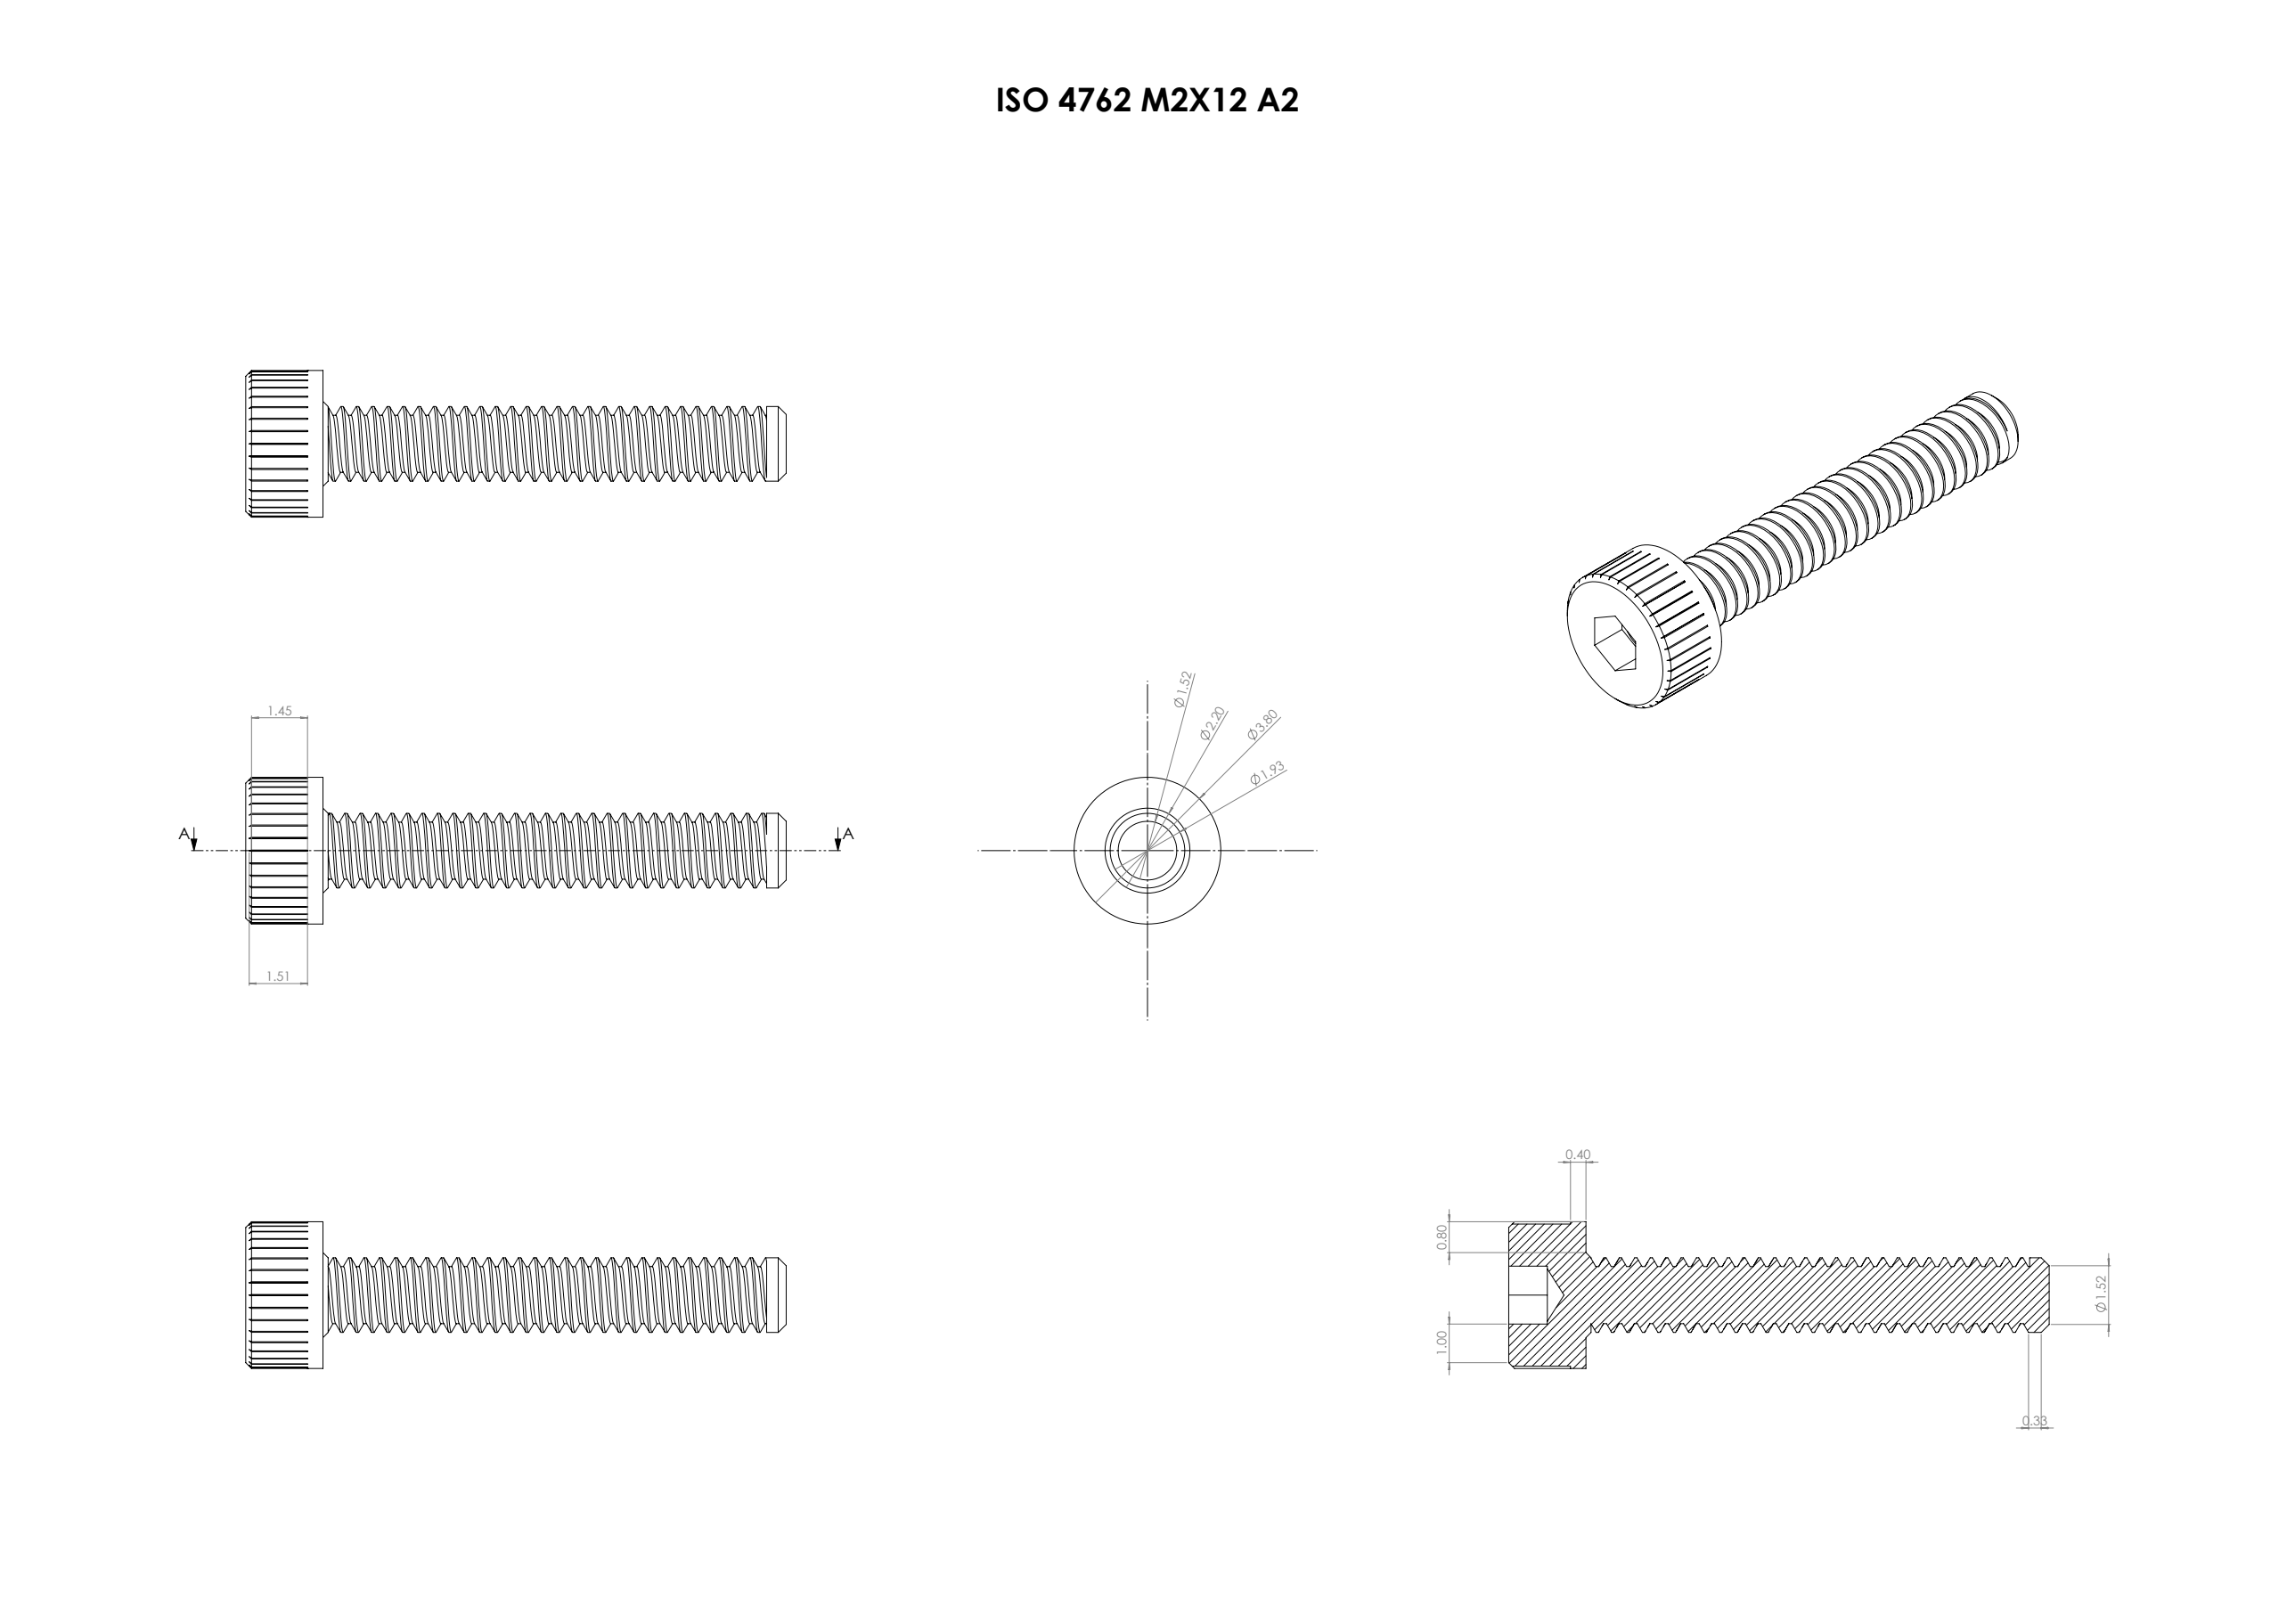
ISO-10303-21;
HEADER;
/* Generated by software containing ST-Developer
 * from STEP Tools, Inc. (www.steptools.com) 
 */

FILE_DESCRIPTION(
/* description */ (''),
/* implementation_level */ '2;1');

FILE_NAME(
/* name */ '15_ISO_4762_M2x12_A2.step',
/* time_stamp */ '2026-10-19T23:00:43-07:00',
/* author */ (''),
/* organization */ (''),
/* preprocessor_version */ 'ST-DEVELOPER v20.2',
/* originating_system */ 'Autodesk Translation Framework v15.15.0.0',
/* authorisation */ '');

FILE_SCHEMA (('AUTOMOTIVE_DESIGN { 1 0 10303 214 3 1 1 }'));
ENDSEC;

DATA;
#10=MECHANICAL_DESIGN_GEOMETRIC_PRESENTATION_REPRESENTATION('',(#1011),#55002);
#251=(
BOUNDED_CURVE()
B_SPLINE_CURVE(2,(#43783,#43784,#43785),.UNSPECIFIED.,.F.,.F.)
B_SPLINE_CURVE_WITH_KNOTS((3,3),(0.,0.00841282944278042),.UNSPECIFIED.)
CURVE()
GEOMETRIC_REPRESENTATION_ITEM()
RATIONAL_B_SPLINE_CURVE((1.,1.00035365746955,1.00043184882983))
REPRESENTATION_ITEM('')
);
#252=(
BOUNDED_CURVE()
B_SPLINE_CURVE(2,(#43789,#43790,#43791),.UNSPECIFIED.,.F.,.F.)
B_SPLINE_CURVE_WITH_KNOTS((3,3),(0.0131888113576721,0.0216016408002996),
 .UNSPECIFIED.)
CURVE()
GEOMETRIC_REPRESENTATION_ITEM()
RATIONAL_B_SPLINE_CURVE((1.00043184882948,1.00035365746926,1.))
REPRESENTATION_ITEM('')
);
#253=(
BOUNDED_CURVE()
B_SPLINE_CURVE(2,(#43804,#43805,#43806),.UNSPECIFIED.,.F.,.F.)
B_SPLINE_CURVE_WITH_KNOTS((3,3),(0.,0.0084128294426201),.UNSPECIFIED.)
CURVE()
GEOMETRIC_REPRESENTATION_ITEM()
RATIONAL_B_SPLINE_CURVE((1.,1.00035365746986,1.00043184883023))
REPRESENTATION_ITEM('')
);
#254=(
BOUNDED_CURVE()
B_SPLINE_CURVE(2,(#43810,#43811,#43812),.UNSPECIFIED.,.F.,.F.)
B_SPLINE_CURVE_WITH_KNOTS((3,3),(0.0131888113575809,0.0216016408002996),
 .UNSPECIFIED.)
CURVE()
GEOMETRIC_REPRESENTATION_ITEM()
RATIONAL_B_SPLINE_CURVE((1.00043184883059,1.00035365747017,1.))
REPRESENTATION_ITEM('')
);
#255=(
BOUNDED_CURVE()
B_SPLINE_CURVE(2,(#43825,#43826,#43827),.UNSPECIFIED.,.F.,.F.)
B_SPLINE_CURVE_WITH_KNOTS((3,3),(0.,0.00841282944278058),.UNSPECIFIED.)
CURVE()
GEOMETRIC_REPRESENTATION_ITEM()
RATIONAL_B_SPLINE_CURVE((1.,1.00035365746906,1.00043184882924))
REPRESENTATION_ITEM('')
);
#256=(
BOUNDED_CURVE()
B_SPLINE_CURVE(2,(#43831,#43832,#43833),.UNSPECIFIED.,.F.,.F.)
B_SPLINE_CURVE_WITH_KNOTS((3,3),(0.0131888113576548,0.0216016408002996),
 .UNSPECIFIED.)
CURVE()
GEOMETRIC_REPRESENTATION_ITEM()
RATIONAL_B_SPLINE_CURVE((1.00043184882846,1.00035365746842,1.))
REPRESENTATION_ITEM('')
);
#257=(
BOUNDED_CURVE()
B_SPLINE_CURVE(2,(#43846,#43847,#43848),.UNSPECIFIED.,.F.,.F.)
B_SPLINE_CURVE_WITH_KNOTS((3,3),(0.,0.00841282944280584),.UNSPECIFIED.)
CURVE()
GEOMETRIC_REPRESENTATION_ITEM()
RATIONAL_B_SPLINE_CURVE((1.,1.00035365746775,1.00043184882763))
REPRESENTATION_ITEM('')
);
#258=(
BOUNDED_CURVE()
B_SPLINE_CURVE(2,(#43852,#43853,#43854),.UNSPECIFIED.,.F.,.F.)
B_SPLINE_CURVE_WITH_KNOTS((3,3),(0.0131888113576015,0.0216016408002996),
 .UNSPECIFIED.)
CURVE()
GEOMETRIC_REPRESENTATION_ITEM()
RATIONAL_B_SPLINE_CURVE((1.00043184882681,1.00035365746707,1.))
REPRESENTATION_ITEM('')
);
#259=(
BOUNDED_CURVE()
B_SPLINE_CURVE(2,(#43867,#43868,#43869),.UNSPECIFIED.,.F.,.F.)
B_SPLINE_CURVE_WITH_KNOTS((3,3),(0.,0.00841282944278488),.UNSPECIFIED.)
CURVE()
GEOMETRIC_REPRESENTATION_ITEM()
RATIONAL_B_SPLINE_CURVE((1.,1.0003536574676,1.00043184882745))
REPRESENTATION_ITEM('')
);
#260=(
BOUNDED_CURVE()
B_SPLINE_CURVE(2,(#43873,#43874,#43875),.UNSPECIFIED.,.F.,.F.)
B_SPLINE_CURVE_WITH_KNOTS((3,3),(0.0131888113575949,0.0216016408002996),
 .UNSPECIFIED.)
CURVE()
GEOMETRIC_REPRESENTATION_ITEM()
RATIONAL_B_SPLINE_CURVE((1.000431848828,1.00035365746804,1.))
REPRESENTATION_ITEM('')
);
#261=(
BOUNDED_CURVE()
B_SPLINE_CURVE(2,(#43888,#43889,#43890),.UNSPECIFIED.,.F.,.F.)
B_SPLINE_CURVE_WITH_KNOTS((3,3),(0.,0.00841282944265237),.UNSPECIFIED.)
CURVE()
GEOMETRIC_REPRESENTATION_ITEM()
RATIONAL_B_SPLINE_CURVE((1.,1.00035365746874,1.00043184882885))
REPRESENTATION_ITEM('')
);
#262=(
BOUNDED_CURVE()
B_SPLINE_CURVE(2,(#43894,#43895,#43896),.UNSPECIFIED.,.F.,.F.)
B_SPLINE_CURVE_WITH_KNOTS((3,3),(0.0131888113575151,0.0216016408002996),
 .UNSPECIFIED.)
CURVE()
GEOMETRIC_REPRESENTATION_ITEM()
RATIONAL_B_SPLINE_CURVE((1.00043184882745,1.0003536574676,1.))
REPRESENTATION_ITEM('')
);
#263=(
BOUNDED_CURVE()
B_SPLINE_CURVE(2,(#43909,#43910,#43911),.UNSPECIFIED.,.F.,.F.)
B_SPLINE_CURVE_WITH_KNOTS((3,3),(0.,0.00841282944265245),.UNSPECIFIED.)
CURVE()
GEOMETRIC_REPRESENTATION_ITEM()
RATIONAL_B_SPLINE_CURVE((1.,1.00035365746621,1.00043184882576))
REPRESENTATION_ITEM('')
);
#264=(
BOUNDED_CURVE()
B_SPLINE_CURVE(2,(#43915,#43916,#43917),.UNSPECIFIED.,.F.,.F.)
B_SPLINE_CURVE_WITH_KNOTS((3,3),(0.013188811357676,0.0216016408002996),
 .UNSPECIFIED.)
CURVE()
GEOMETRIC_REPRESENTATION_ITEM()
RATIONAL_B_SPLINE_CURVE((1.00043184882966,1.0003536574694,1.))
REPRESENTATION_ITEM('')
);
#265=(
BOUNDED_CURVE()
B_SPLINE_CURVE(2,(#43930,#43931,#43932),.UNSPECIFIED.,.F.,.F.)
B_SPLINE_CURVE_WITH_KNOTS((3,3),(0.,0.00841282944263587),.UNSPECIFIED.)
CURVE()
GEOMETRIC_REPRESENTATION_ITEM()
RATIONAL_B_SPLINE_CURVE((1.,1.00035365746699,1.00043184882672))
REPRESENTATION_ITEM('')
);
#266=(
BOUNDED_CURVE()
B_SPLINE_CURVE(2,(#43936,#43937,#43938),.UNSPECIFIED.,.F.,.F.)
B_SPLINE_CURVE_WITH_KNOTS((3,3),(0.0131888113575321,0.0216016408002996),
 .UNSPECIFIED.)
CURVE()
GEOMETRIC_REPRESENTATION_ITEM()
RATIONAL_B_SPLINE_CURVE((1.00043184883015,1.00035365746981,1.))
REPRESENTATION_ITEM('')
);
#267=(
BOUNDED_CURVE()
B_SPLINE_CURVE(2,(#43951,#43952,#43953),.UNSPECIFIED.,.F.,.F.)
B_SPLINE_CURVE_WITH_KNOTS((3,3),(0.,0.00841282944268715),.UNSPECIFIED.)
CURVE()
GEOMETRIC_REPRESENTATION_ITEM()
RATIONAL_B_SPLINE_CURVE((1.,1.00035365746714,1.0004318488269))
REPRESENTATION_ITEM('')
);
#268=(
BOUNDED_CURVE()
B_SPLINE_CURVE(2,(#43957,#43958,#43959),.UNSPECIFIED.,.F.,.F.)
B_SPLINE_CURVE_WITH_KNOTS((3,3),(0.0131888113576173,0.0216016408002996),
 .UNSPECIFIED.)
CURVE()
GEOMETRIC_REPRESENTATION_ITEM()
RATIONAL_B_SPLINE_CURVE((1.00043184882651,1.00035365746683,1.))
REPRESENTATION_ITEM('')
);
#269=(
BOUNDED_CURVE()
B_SPLINE_CURVE(2,(#43972,#43973,#43974),.UNSPECIFIED.,.F.,.F.)
B_SPLINE_CURVE_WITH_KNOTS((3,3),(0.,0.00841282944268232),.UNSPECIFIED.)
CURVE()
GEOMETRIC_REPRESENTATION_ITEM()
RATIONAL_B_SPLINE_CURVE((1.,1.00035365746714,1.0004318488269))
REPRESENTATION_ITEM('')
);
#270=(
BOUNDED_CURVE()
B_SPLINE_CURVE(2,(#43978,#43979,#43980),.UNSPECIFIED.,.F.,.F.)
B_SPLINE_CURVE_WITH_KNOTS((3,3),(0.0131888113576523,0.0216016408002997),
 .UNSPECIFIED.)
CURVE()
GEOMETRIC_REPRESENTATION_ITEM()
RATIONAL_B_SPLINE_CURVE((1.00043184882641,1.00035365746674,1.))
REPRESENTATION_ITEM('')
);
#271=(
BOUNDED_CURVE()
B_SPLINE_CURVE(2,(#43993,#43994,#43995),.UNSPECIFIED.,.F.,.F.)
B_SPLINE_CURVE_WITH_KNOTS((3,3),(0.,0.00841282944262782),.UNSPECIFIED.)
CURVE()
GEOMETRIC_REPRESENTATION_ITEM()
RATIONAL_B_SPLINE_CURVE((1.,1.00035365747069,1.00043184883123))
REPRESENTATION_ITEM('')
);
#272=(
BOUNDED_CURVE()
B_SPLINE_CURVE(2,(#43999,#44000,#44001),.UNSPECIFIED.,.F.,.F.)
B_SPLINE_CURVE_WITH_KNOTS((3,3),(0.0131888113575803,0.0216016408002996),
 .UNSPECIFIED.)
CURVE()
GEOMETRIC_REPRESENTATION_ITEM()
RATIONAL_B_SPLINE_CURVE((1.00043184883154,1.00035365747094,1.))
REPRESENTATION_ITEM('')
);
#273=(
BOUNDED_CURVE()
B_SPLINE_CURVE(2,(#44014,#44015,#44016),.UNSPECIFIED.,.F.,.F.)
B_SPLINE_CURVE_WITH_KNOTS((3,3),(0.,0.00841282944278058),.UNSPECIFIED.)
CURVE()
GEOMETRIC_REPRESENTATION_ITEM()
RATIONAL_B_SPLINE_CURVE((1.,1.00035365746906,1.00043184882924))
REPRESENTATION_ITEM('')
);
#274=(
BOUNDED_CURVE()
B_SPLINE_CURVE(2,(#44020,#44021,#44022),.UNSPECIFIED.,.F.,.F.)
B_SPLINE_CURVE_WITH_KNOTS((3,3),(0.0131888113576548,0.0216016408002996),
 .UNSPECIFIED.)
CURVE()
GEOMETRIC_REPRESENTATION_ITEM()
RATIONAL_B_SPLINE_CURVE((1.00043184882846,1.00035365746842,1.))
REPRESENTATION_ITEM('')
);
#275=(
BOUNDED_CURVE()
B_SPLINE_CURVE(2,(#44035,#44036,#44037),.UNSPECIFIED.,.F.,.F.)
B_SPLINE_CURVE_WITH_KNOTS((3,3),(0.,0.00841282944280138),.UNSPECIFIED.)
CURVE()
GEOMETRIC_REPRESENTATION_ITEM()
RATIONAL_B_SPLINE_CURVE((1.,1.00035365746471,1.00043184882392))
REPRESENTATION_ITEM('')
);
#276=(
BOUNDED_CURVE()
B_SPLINE_CURVE(2,(#44041,#44042,#44043),.UNSPECIFIED.,.F.,.F.)
B_SPLINE_CURVE_WITH_KNOTS((3,3),(0.0131888113575931,0.0216016408002996),
 .UNSPECIFIED.)
CURVE()
GEOMETRIC_REPRESENTATION_ITEM()
RATIONAL_B_SPLINE_CURVE((1.00043184882494,1.00035365746554,1.))
REPRESENTATION_ITEM('')
);
#277=(
BOUNDED_CURVE()
B_SPLINE_CURVE(2,(#44056,#44057,#44058),.UNSPECIFIED.,.F.,.F.)
B_SPLINE_CURVE_WITH_KNOTS((3,3),(0.,0.00841282944261464),.UNSPECIFIED.)
CURVE()
GEOMETRIC_REPRESENTATION_ITEM()
RATIONAL_B_SPLINE_CURVE((1.,1.00035365746679,1.00043184882648))
REPRESENTATION_ITEM('')
);
#278=(
BOUNDED_CURVE()
B_SPLINE_CURVE(2,(#44062,#44063,#44064),.UNSPECIFIED.,.F.,.F.)
B_SPLINE_CURVE_WITH_KNOTS((3,3),(0.0131888113575887,0.0216016408002996),
 .UNSPECIFIED.)
CURVE()
GEOMETRIC_REPRESENTATION_ITEM()
RATIONAL_B_SPLINE_CURVE((1.00043184882758,1.0003536574677,1.))
REPRESENTATION_ITEM('')
);
#279=(
BOUNDED_CURVE()
B_SPLINE_CURVE(2,(#44077,#44078,#44079),.UNSPECIFIED.,.F.,.F.)
B_SPLINE_CURVE_WITH_KNOTS((3,3),(0.,0.00841282944265251),.UNSPECIFIED.)
CURVE()
GEOMETRIC_REPRESENTATION_ITEM()
RATIONAL_B_SPLINE_CURVE((1.,1.00035365746762,1.00043184882748))
REPRESENTATION_ITEM('')
);
#280=(
BOUNDED_CURVE()
B_SPLINE_CURVE(2,(#44083,#44084,#44085),.UNSPECIFIED.,.F.,.F.)
B_SPLINE_CURVE_WITH_KNOTS((3,3),(0.0131888113576473,0.0216016408002996),
 .UNSPECIFIED.)
CURVE()
GEOMETRIC_REPRESENTATION_ITEM()
RATIONAL_B_SPLINE_CURVE((1.00043184883165,1.00035365747103,1.))
REPRESENTATION_ITEM('')
);
#281=(
BOUNDED_CURVE()
B_SPLINE_CURVE(2,(#44098,#44099,#44100),.UNSPECIFIED.,.F.,.F.)
B_SPLINE_CURVE_WITH_KNOTS((3,3),(0.,0.00841282944262983),.UNSPECIFIED.)
CURVE()
GEOMETRIC_REPRESENTATION_ITEM()
RATIONAL_B_SPLINE_CURVE((1.,1.00035365747139,1.00043184883209))
REPRESENTATION_ITEM('')
);
#282=(
BOUNDED_CURVE()
B_SPLINE_CURVE(2,(#44104,#44105,#44106),.UNSPECIFIED.,.F.,.F.)
B_SPLINE_CURVE_WITH_KNOTS((3,3),(0.0131888113576388,0.0216016408002996),
 .UNSPECIFIED.)
CURVE()
GEOMETRIC_REPRESENTATION_ITEM()
RATIONAL_B_SPLINE_CURVE((1.00043184882737,1.00035365746753,1.))
REPRESENTATION_ITEM('')
);
#283=(
BOUNDED_CURVE()
B_SPLINE_CURVE(2,(#44119,#44120,#44121),.UNSPECIFIED.,.F.,.F.)
B_SPLINE_CURVE_WITH_KNOTS((3,3),(0.,0.00841282944261306),.UNSPECIFIED.)
CURVE()
GEOMETRIC_REPRESENTATION_ITEM()
RATIONAL_B_SPLINE_CURVE((1.,1.00035365747318,1.00043184883428))
REPRESENTATION_ITEM('')
);
#284=(
BOUNDED_CURVE()
B_SPLINE_CURVE(2,(#44125,#44126,#44127),.UNSPECIFIED.,.F.,.F.)
B_SPLINE_CURVE_WITH_KNOTS((3,3),(0.0131888113575341,0.0216016408002996),
 .UNSPECIFIED.)
CURVE()
GEOMETRIC_REPRESENTATION_ITEM()
RATIONAL_B_SPLINE_CURVE((1.00043184882813,1.00035365746816,1.))
REPRESENTATION_ITEM('')
);
#285=(
BOUNDED_CURVE()
B_SPLINE_CURVE(2,(#44142,#44143,#44144),.UNSPECIFIED.,.F.,.F.)
B_SPLINE_CURVE_WITH_KNOTS((3,3),(0.,0.00841282944268199),.UNSPECIFIED.)
CURVE()
GEOMETRIC_REPRESENTATION_ITEM()
RATIONAL_B_SPLINE_CURVE((1.,1.00035365746877,1.00043184882888))
REPRESENTATION_ITEM('')
);
#286=(
BOUNDED_CURVE()
B_SPLINE_CURVE(2,(#44148,#44149,#44150),.UNSPECIFIED.,.F.,.F.)
B_SPLINE_CURVE_WITH_KNOTS((3,3),(0.0131888113576103,0.0216016408002996),
 .UNSPECIFIED.)
CURVE()
GEOMETRIC_REPRESENTATION_ITEM()
RATIONAL_B_SPLINE_CURVE((1.00043184882915,1.00035365746898,1.))
REPRESENTATION_ITEM('')
);
#287=(
BOUNDED_CURVE()
B_SPLINE_CURVE(2,(#44163,#44164,#44165),.UNSPECIFIED.,.F.,.F.)
B_SPLINE_CURVE_WITH_KNOTS((3,3),(0.,0.00841282944276111),.UNSPECIFIED.)
CURVE()
GEOMETRIC_REPRESENTATION_ITEM()
RATIONAL_B_SPLINE_CURVE((1.,1.00035365746789,1.00043184882782))
REPRESENTATION_ITEM('')
);
#288=(
BOUNDED_CURVE()
B_SPLINE_CURVE(2,(#44169,#44170,#44171),.UNSPECIFIED.,.F.,.F.)
B_SPLINE_CURVE_WITH_KNOTS((3,3),(0.013188811357663,0.0216016408002997),
 .UNSPECIFIED.)
CURVE()
GEOMETRIC_REPRESENTATION_ITEM()
RATIONAL_B_SPLINE_CURVE((1.00043184882852,1.00035365746847,1.))
REPRESENTATION_ITEM('')
);
#289=(
BOUNDED_CURVE()
B_SPLINE_CURVE(2,(#44184,#44185,#44186),.UNSPECIFIED.,.F.,.F.)
B_SPLINE_CURVE_WITH_KNOTS((3,3),(0.,0.00841282944263208),.UNSPECIFIED.)
CURVE()
GEOMETRIC_REPRESENTATION_ITEM()
RATIONAL_B_SPLINE_CURVE((1.,1.00035365746816,1.00043184882815))
REPRESENTATION_ITEM('')
);
#290=(
BOUNDED_CURVE()
B_SPLINE_CURVE(2,(#44190,#44191,#44192),.UNSPECIFIED.,.F.,.F.)
B_SPLINE_CURVE_WITH_KNOTS((3,3),(0.013188811357748,0.0216016408002996),
 .UNSPECIFIED.)
CURVE()
GEOMETRIC_REPRESENTATION_ITEM()
RATIONAL_B_SPLINE_CURVE((1.00043184883132,1.00035365747076,1.))
REPRESENTATION_ITEM('')
);
#291=(
BOUNDED_CURVE()
B_SPLINE_CURVE(2,(#44205,#44206,#44207),.UNSPECIFIED.,.F.,.F.)
B_SPLINE_CURVE_WITH_KNOTS((3,3),(0.,0.00841282944264326),.UNSPECIFIED.)
CURVE()
GEOMETRIC_REPRESENTATION_ITEM()
RATIONAL_B_SPLINE_CURVE((1.,1.00035365746759,1.00043184882744))
REPRESENTATION_ITEM('')
);
#292=(
BOUNDED_CURVE()
B_SPLINE_CURVE(2,(#44211,#44212,#44213),.UNSPECIFIED.,.F.,.F.)
B_SPLINE_CURVE_WITH_KNOTS((3,3),(0.0131888113575487,0.0216016408002996),
 .UNSPECIFIED.)
CURVE()
GEOMETRIC_REPRESENTATION_ITEM()
RATIONAL_B_SPLINE_CURVE((1.0004318488259,1.00035365746632,1.))
REPRESENTATION_ITEM('')
);
#293=(
BOUNDED_CURVE()
B_SPLINE_CURVE(2,(#44226,#44227,#44228),.UNSPECIFIED.,.F.,.F.)
B_SPLINE_CURVE_WITH_KNOTS((3,3),(0.,0.00841282944280138),.UNSPECIFIED.)
CURVE()
GEOMETRIC_REPRESENTATION_ITEM()
RATIONAL_B_SPLINE_CURVE((1.,1.00035365746471,1.00043184882392))
REPRESENTATION_ITEM('')
);
#294=(
BOUNDED_CURVE()
B_SPLINE_CURVE(2,(#44232,#44233,#44234),.UNSPECIFIED.,.F.,.F.)
B_SPLINE_CURVE_WITH_KNOTS((3,3),(0.0131888113575931,0.0216016408002996),
 .UNSPECIFIED.)
CURVE()
GEOMETRIC_REPRESENTATION_ITEM()
RATIONAL_B_SPLINE_CURVE((1.00043184882494,1.00035365746554,1.))
REPRESENTATION_ITEM('')
);
#295=(
BOUNDED_CURVE()
B_SPLINE_CURVE(2,(#44247,#44248,#44249),.UNSPECIFIED.,.F.,.F.)
B_SPLINE_CURVE_WITH_KNOTS((3,3),(0.,0.00841282944270105),.UNSPECIFIED.)
CURVE()
GEOMETRIC_REPRESENTATION_ITEM()
RATIONAL_B_SPLINE_CURVE((1.,1.000353657467,1.00043184882673))
REPRESENTATION_ITEM('')
);
#296=(
BOUNDED_CURVE()
B_SPLINE_CURVE(2,(#44253,#44254,#44255),.UNSPECIFIED.,.F.,.F.)
B_SPLINE_CURVE_WITH_KNOTS((3,3),(0.0131888113574971,0.0216016408002996),
 .UNSPECIFIED.)
CURVE()
GEOMETRIC_REPRESENTATION_ITEM()
RATIONAL_B_SPLINE_CURVE((1.00043184882773,1.00035365746783,1.))
REPRESENTATION_ITEM('')
);
#297=(
BOUNDED_CURVE()
B_SPLINE_CURVE(2,(#44268,#44269,#44270),.UNSPECIFIED.,.F.,.F.)
B_SPLINE_CURVE_WITH_KNOTS((3,3),(0.,0.00841282944264652),.UNSPECIFIED.)
CURVE()
GEOMETRIC_REPRESENTATION_ITEM()
RATIONAL_B_SPLINE_CURVE((1.,1.00035365746972,1.00043184883004))
REPRESENTATION_ITEM('')
);
#298=(
BOUNDED_CURVE()
B_SPLINE_CURVE(2,(#44274,#44275,#44276),.UNSPECIFIED.,.F.,.F.)
B_SPLINE_CURVE_WITH_KNOTS((3,3),(0.0131888113576371,0.0216016408002996),
 .UNSPECIFIED.)
CURVE()
GEOMETRIC_REPRESENTATION_ITEM()
RATIONAL_B_SPLINE_CURVE((1.00043184882659,1.00035365746689,1.))
REPRESENTATION_ITEM('')
);
#299=(
BOUNDED_CURVE()
B_SPLINE_CURVE(2,(#44289,#44290,#44291),.UNSPECIFIED.,.F.,.F.)
B_SPLINE_CURVE_WITH_KNOTS((3,3),(0.,0.00841282944262983),.UNSPECIFIED.)
CURVE()
GEOMETRIC_REPRESENTATION_ITEM()
RATIONAL_B_SPLINE_CURVE((1.,1.00035365747139,1.00043184883209))
REPRESENTATION_ITEM('')
);
#300=(
BOUNDED_CURVE()
B_SPLINE_CURVE(2,(#44295,#44296,#44297),.UNSPECIFIED.,.F.,.F.)
B_SPLINE_CURVE_WITH_KNOTS((3,3),(0.0131888113576388,0.0216016408002996),
 .UNSPECIFIED.)
CURVE()
GEOMETRIC_REPRESENTATION_ITEM()
RATIONAL_B_SPLINE_CURVE((1.00043184882737,1.00035365746753,1.))
REPRESENTATION_ITEM('')
);
#301=(
BOUNDED_CURVE()
B_SPLINE_CURVE(2,(#44310,#44311,#44312),.UNSPECIFIED.,.F.,.F.)
B_SPLINE_CURVE_WITH_KNOTS((3,3),(0.,0.00841282944264003),.UNSPECIFIED.)
CURVE()
GEOMETRIC_REPRESENTATION_ITEM()
RATIONAL_B_SPLINE_CURVE((1.,1.0003536574673,1.00043184882709))
REPRESENTATION_ITEM('')
);
#302=(
BOUNDED_CURVE()
B_SPLINE_CURVE(2,(#44316,#44317,#44318),.UNSPECIFIED.,.F.,.F.)
B_SPLINE_CURVE_WITH_KNOTS((3,3),(0.0131888113576155,0.0216016408002996),
 .UNSPECIFIED.)
CURVE()
GEOMETRIC_REPRESENTATION_ITEM()
RATIONAL_B_SPLINE_CURVE((1.00043184882608,1.00035365746647,1.))
REPRESENTATION_ITEM('')
);
#303=(
BOUNDED_CURVE()
B_SPLINE_CURVE(2,(#44331,#44332,#44333),.UNSPECIFIED.,.F.,.F.)
B_SPLINE_CURVE_WITH_KNOTS((3,3),(0.,0.00841282944269557),.UNSPECIFIED.)
CURVE()
GEOMETRIC_REPRESENTATION_ITEM()
RATIONAL_B_SPLINE_CURVE((1.,1.00035365746722,1.000431848827))
REPRESENTATION_ITEM('')
);
#304=(
BOUNDED_CURVE()
B_SPLINE_CURVE(2,(#44337,#44338,#44339),.UNSPECIFIED.,.F.,.F.)
B_SPLINE_CURVE_WITH_KNOTS((3,3),(0.0131888113576143,0.0216016408002996),
 .UNSPECIFIED.)
CURVE()
GEOMETRIC_REPRESENTATION_ITEM()
RATIONAL_B_SPLINE_CURVE((1.00043184882947,1.00035365746925,1.))
REPRESENTATION_ITEM('')
);
#305=(
BOUNDED_CURVE()
B_SPLINE_CURVE(2,(#44352,#44353,#44354),.UNSPECIFIED.,.F.,.F.)
B_SPLINE_CURVE_WITH_KNOTS((3,3),(0.,0.00841282944278065),.UNSPECIFIED.)
CURVE()
GEOMETRIC_REPRESENTATION_ITEM()
RATIONAL_B_SPLINE_CURVE((1.,1.00035365746947,1.00043184882974))
REPRESENTATION_ITEM('')
);
#306=(
BOUNDED_CURVE()
B_SPLINE_CURVE(2,(#44358,#44359,#44360),.UNSPECIFIED.,.F.,.F.)
B_SPLINE_CURVE_WITH_KNOTS((3,3),(0.0131888113576697,0.0216016408002996),
 .UNSPECIFIED.)
CURVE()
GEOMETRIC_REPRESENTATION_ITEM()
RATIONAL_B_SPLINE_CURVE((1.00043184882899,1.00035365746886,1.))
REPRESENTATION_ITEM('')
);
#307=(
BOUNDED_CURVE()
B_SPLINE_CURVE(2,(#44373,#44374,#44375),.UNSPECIFIED.,.F.,.F.)
B_SPLINE_CURVE_WITH_KNOTS((3,3),(0.,0.00841282944263208),.UNSPECIFIED.)
CURVE()
GEOMETRIC_REPRESENTATION_ITEM()
RATIONAL_B_SPLINE_CURVE((1.,1.00035365746816,1.00043184882815))
REPRESENTATION_ITEM('')
);
#308=(
BOUNDED_CURVE()
B_SPLINE_CURVE(2,(#44379,#44380,#44381),.UNSPECIFIED.,.F.,.F.)
B_SPLINE_CURVE_WITH_KNOTS((3,3),(0.013188811357748,0.0216016408002996),
 .UNSPECIFIED.)
CURVE()
GEOMETRIC_REPRESENTATION_ITEM()
RATIONAL_B_SPLINE_CURVE((1.00043184883132,1.00035365747076,1.))
REPRESENTATION_ITEM('')
);
#309=(
BOUNDED_CURVE()
B_SPLINE_CURVE(2,(#44394,#44395,#44396),.UNSPECIFIED.,.F.,.F.)
B_SPLINE_CURVE_WITH_KNOTS((3,3),(0.,0.00841282944273455),.UNSPECIFIED.)
CURVE()
GEOMETRIC_REPRESENTATION_ITEM()
RATIONAL_B_SPLINE_CURVE((1.,1.00035365746539,1.00043184882476))
REPRESENTATION_ITEM('')
);
#310=(
BOUNDED_CURVE()
B_SPLINE_CURVE(2,(#44400,#44401,#44402),.UNSPECIFIED.,.F.,.F.)
B_SPLINE_CURVE_WITH_KNOTS((3,3),(0.0131888113576539,0.0216016408002996),
 .UNSPECIFIED.)
CURVE()
GEOMETRIC_REPRESENTATION_ITEM()
RATIONAL_B_SPLINE_CURVE((1.00043184882929,1.0003536574691,1.))
REPRESENTATION_ITEM('')
);
#311=(
BOUNDED_CURVE()
B_SPLINE_CURVE(2,(#44415,#44416,#44417),.UNSPECIFIED.,.F.,.F.)
B_SPLINE_CURVE_WITH_KNOTS((3,3),(0.,0.00841282944270133),.UNSPECIFIED.)
CURVE()
GEOMETRIC_REPRESENTATION_ITEM()
RATIONAL_B_SPLINE_CURVE((1.,1.00035365747008,1.00043184883048))
REPRESENTATION_ITEM('')
);
#312=(
BOUNDED_CURVE()
B_SPLINE_CURVE(2,(#44421,#44422,#44423),.UNSPECIFIED.,.F.,.F.)
B_SPLINE_CURVE_WITH_KNOTS((3,3),(0.0131888113576197,0.0216016408002996),
 .UNSPECIFIED.)
CURVE()
GEOMETRIC_REPRESENTATION_ITEM()
RATIONAL_B_SPLINE_CURVE((1.00043184882798,1.00035365746803,1.))
REPRESENTATION_ITEM('')
);
#313=(
BOUNDED_CURVE()
B_SPLINE_CURVE(2,(#44436,#44437,#44438),.UNSPECIFIED.,.F.,.F.)
B_SPLINE_CURVE_WITH_KNOTS((3,3),(0.,0.00841282944261464),.UNSPECIFIED.)
CURVE()
GEOMETRIC_REPRESENTATION_ITEM()
RATIONAL_B_SPLINE_CURVE((1.,1.00035365746679,1.00043184882648))
REPRESENTATION_ITEM('')
);
#314=(
BOUNDED_CURVE()
B_SPLINE_CURVE(2,(#44442,#44443,#44444),.UNSPECIFIED.,.F.,.F.)
B_SPLINE_CURVE_WITH_KNOTS((3,3),(0.0131888113575887,0.0216016408002996),
 .UNSPECIFIED.)
CURVE()
GEOMETRIC_REPRESENTATION_ITEM()
RATIONAL_B_SPLINE_CURVE((1.00043184882758,1.0003536574677,1.))
REPRESENTATION_ITEM('')
);
#315=(
BOUNDED_CURVE()
B_SPLINE_CURVE(2,(#44457,#44458,#44459),.UNSPECIFIED.,.F.,.F.)
B_SPLINE_CURVE_WITH_KNOTS((3,3),(0.,0.00841282944264924),.UNSPECIFIED.)
CURVE()
GEOMETRIC_REPRESENTATION_ITEM()
RATIONAL_B_SPLINE_CURVE((1.,1.00035365746952,1.00043184882981))
REPRESENTATION_ITEM('')
);
#316=(
BOUNDED_CURVE()
B_SPLINE_CURVE(2,(#44463,#44464,#44465),.UNSPECIFIED.,.F.,.F.)
B_SPLINE_CURVE_WITH_KNOTS((3,3),(0.0131888113576407,0.0216016408002996),
 .UNSPECIFIED.)
CURVE()
GEOMETRIC_REPRESENTATION_ITEM()
RATIONAL_B_SPLINE_CURVE((1.00043184882821,1.00035365746821,1.))
REPRESENTATION_ITEM('')
);
#317=(
BOUNDED_CURVE()
B_SPLINE_CURVE(2,(#44478,#44479,#44480),.UNSPECIFIED.,.F.,.F.)
B_SPLINE_CURVE_WITH_KNOTS((3,3),(0.,0.00841282944262983),.UNSPECIFIED.)
CURVE()
GEOMETRIC_REPRESENTATION_ITEM()
RATIONAL_B_SPLINE_CURVE((1.,1.00035365747139,1.00043184883209))
REPRESENTATION_ITEM('')
);
#318=(
BOUNDED_CURVE()
B_SPLINE_CURVE(2,(#44484,#44485,#44486),.UNSPECIFIED.,.F.,.F.)
B_SPLINE_CURVE_WITH_KNOTS((3,3),(0.0131888113576388,0.0216016408002996),
 .UNSPECIFIED.)
CURVE()
GEOMETRIC_REPRESENTATION_ITEM()
RATIONAL_B_SPLINE_CURVE((1.00043184882737,1.00035365746753,1.))
REPRESENTATION_ITEM('')
);
#319=(
BOUNDED_CURVE()
B_SPLINE_CURVE(2,(#44499,#44500,#44501),.UNSPECIFIED.,.F.,.F.)
B_SPLINE_CURVE_WITH_KNOTS((3,3),(0.,0.0084128294426321),.UNSPECIFIED.)
CURVE()
GEOMETRIC_REPRESENTATION_ITEM()
RATIONAL_B_SPLINE_CURVE((1.,1.00035365746883,1.00043184882896))
REPRESENTATION_ITEM('')
);
#320=(
BOUNDED_CURVE()
B_SPLINE_CURVE(2,(#44505,#44506,#44507),.UNSPECIFIED.,.F.,.F.)
B_SPLINE_CURVE_WITH_KNOTS((3,3),(0.0131888113575073,0.0216016408002996),
 .UNSPECIFIED.)
CURVE()
GEOMETRIC_REPRESENTATION_ITEM()
RATIONAL_B_SPLINE_CURVE((1.00043184882395,1.00035365746473,1.))
REPRESENTATION_ITEM('')
);
#321=(
BOUNDED_CURVE()
B_SPLINE_CURVE(2,(#44560,#44561,#44562),.UNSPECIFIED.,.F.,.F.)
B_SPLINE_CURVE_WITH_KNOTS((3,3),(0.,0.00841282944285724),.UNSPECIFIED.)
CURVE()
GEOMETRIC_REPRESENTATION_ITEM()
RATIONAL_B_SPLINE_CURVE((1.,1.00035365746964,1.00043184882994))
REPRESENTATION_ITEM('')
);
#322=(
BOUNDED_CURVE()
B_SPLINE_CURVE(2,(#44564,#44565,#44566),.UNSPECIFIED.,.F.,.F.)
B_SPLINE_CURVE_WITH_KNOTS((3,3),(0.0131888113574265,0.0216016408002996),
 .UNSPECIFIED.)
CURVE()
GEOMETRIC_REPRESENTATION_ITEM()
RATIONAL_B_SPLINE_CURVE((1.00043184882266,1.00035365746368,1.))
REPRESENTATION_ITEM('')
);
#474=B_SPLINE_SURFACE_WITH_KNOTS('',3,3,((#42155,#42156,#42157,#42158,#42159,
#42160,#42161,#42162,#42163,#42164,#42165,#42166,#42167,#42168,#42169,#42170,
#42171,#42172,#42173,#42174,#42175,#42176,#42177,#42178,#42179,#42180,#42181,
#42182,#42183,#42184,#42185,#42186,#42187,#42188,#42189,#42190,#42191,#42192,
#42193,#42194,#42195,#42196,#42197,#42198,#42199,#42200,#42201,#42202,#42203,
#42204,#42205,#42206,#42207,#42208,#42209,#42210,#42211,#42212,#42213,#42214,
#42215,#42216,#42217,#42218,#42219,#42220,#42221,#42222,#42223,#42224,#42225,
#42226,#42227,#42228,#42229,#42230,#42231,#42232,#42233,#42234,#42235,#42236,
#42237,#42238,#42239,#42240,#42241,#42242,#42243,#42244,#42245,#42246,#42247,
#42248,#42249,#42250,#42251,#42252,#42253,#42254,#42255,#42256,#42257,#42258,
#42259,#42260,#42261,#42262,#42263,#42264,#42265,#42266,#42267,#42268,#42269,
#42270,#42271,#42272,#42273,#42274,#42275,#42276,#42277,#42278,#42279,#42280,
#42281,#42282,#42283,#42284,#42285,#42286,#42287,#42288,#42289,#42290,#42291,
#42292,#42293,#42294,#42295,#42296,#42297,#42298,#42299,#42300,#42301,#42302,
#42303,#42304,#42305,#42306,#42307,#42308,#42309,#42310,#42311,#42312,#42313,
#42314,#42315,#42316,#42317,#42318,#42319,#42320,#42321,#42322,#42323,#42324,
#42325,#42326,#42327,#42328,#42329,#42330,#42331,#42332,#42333,#42334,#42335,
#42336,#42337,#42338),(#42339,#42340,#42341,#42342,#42343,#42344,#42345,
#42346,#42347,#42348,#42349,#42350,#42351,#42352,#42353,#42354,#42355,#42356,
#42357,#42358,#42359,#42360,#42361,#42362,#42363,#42364,#42365,#42366,#42367,
#42368,#42369,#42370,#42371,#42372,#42373,#42374,#42375,#42376,#42377,#42378,
#42379,#42380,#42381,#42382,#42383,#42384,#42385,#42386,#42387,#42388,#42389,
#42390,#42391,#42392,#42393,#42394,#42395,#42396,#42397,#42398,#42399,#42400,
#42401,#42402,#42403,#42404,#42405,#42406,#42407,#42408,#42409,#42410,#42411,
#42412,#42413,#42414,#42415,#42416,#42417,#42418,#42419,#42420,#42421,#42422,
#42423,#42424,#42425,#42426,#42427,#42428,#42429,#42430,#42431,#42432,#42433,
#42434,#42435,#42436,#42437,#42438,#42439,#42440,#42441,#42442,#42443,#42444,
#42445,#42446,#42447,#42448,#42449,#42450,#42451,#42452,#42453,#42454,#42455,
#42456,#42457,#42458,#42459,#42460,#42461,#42462,#42463,#42464,#42465,#42466,
#42467,#42468,#42469,#42470,#42471,#42472,#42473,#42474,#42475,#42476,#42477,
#42478,#42479,#42480,#42481,#42482,#42483,#42484,#42485,#42486,#42487,#42488,
#42489,#42490,#42491,#42492,#42493,#42494,#42495,#42496,#42497,#42498,#42499,
#42500,#42501,#42502,#42503,#42504,#42505,#42506,#42507,#42508,#42509,#42510,
#42511,#42512,#42513,#42514,#42515,#42516,#42517,#42518,#42519,#42520,#42521,
#42522),(#42523,#42524,#42525,#42526,#42527,#42528,#42529,#42530,#42531,
#42532,#42533,#42534,#42535,#42536,#42537,#42538,#42539,#42540,#42541,#42542,
#42543,#42544,#42545,#42546,#42547,#42548,#42549,#42550,#42551,#42552,#42553,
#42554,#42555,#42556,#42557,#42558,#42559,#42560,#42561,#42562,#42563,#42564,
#42565,#42566,#42567,#42568,#42569,#42570,#42571,#42572,#42573,#42574,#42575,
#42576,#42577,#42578,#42579,#42580,#42581,#42582,#42583,#42584,#42585,#42586,
#42587,#42588,#42589,#42590,#42591,#42592,#42593,#42594,#42595,#42596,#42597,
#42598,#42599,#42600,#42601,#42602,#42603,#42604,#42605,#42606,#42607,#42608,
#42609,#42610,#42611,#42612,#42613,#42614,#42615,#42616,#42617,#42618,#42619,
#42620,#42621,#42622,#42623,#42624,#42625,#42626,#42627,#42628,#42629,#42630,
#42631,#42632,#42633,#42634,#42635,#42636,#42637,#42638,#42639,#42640,#42641,
#42642,#42643,#42644,#42645,#42646,#42647,#42648,#42649,#42650,#42651,#42652,
#42653,#42654,#42655,#42656,#42657,#42658,#42659,#42660,#42661,#42662,#42663,
#42664,#42665,#42666,#42667,#42668,#42669,#42670,#42671,#42672,#42673,#42674,
#42675,#42676,#42677,#42678,#42679,#42680,#42681,#42682,#42683,#42684,#42685,
#42686,#42687,#42688,#42689,#42690,#42691,#42692,#42693,#42694,#42695,#42696,
#42697,#42698,#42699,#42700,#42701,#42702,#42703,#42704,#42705,#42706),
(#42707,#42708,#42709,#42710,#42711,#42712,#42713,#42714,#42715,#42716,
#42717,#42718,#42719,#42720,#42721,#42722,#42723,#42724,#42725,#42726,#42727,
#42728,#42729,#42730,#42731,#42732,#42733,#42734,#42735,#42736,#42737,#42738,
#42739,#42740,#42741,#42742,#42743,#42744,#42745,#42746,#42747,#42748,#42749,
#42750,#42751,#42752,#42753,#42754,#42755,#42756,#42757,#42758,#42759,#42760,
#42761,#42762,#42763,#42764,#42765,#42766,#42767,#42768,#42769,#42770,#42771,
#42772,#42773,#42774,#42775,#42776,#42777,#42778,#42779,#42780,#42781,#42782,
#42783,#42784,#42785,#42786,#42787,#42788,#42789,#42790,#42791,#42792,#42793,
#42794,#42795,#42796,#42797,#42798,#42799,#42800,#42801,#42802,#42803,#42804,
#42805,#42806,#42807,#42808,#42809,#42810,#42811,#42812,#42813,#42814,#42815,
#42816,#42817,#42818,#42819,#42820,#42821,#42822,#42823,#42824,#42825,#42826,
#42827,#42828,#42829,#42830,#42831,#42832,#42833,#42834,#42835,#42836,#42837,
#42838,#42839,#42840,#42841,#42842,#42843,#42844,#42845,#42846,#42847,#42848,
#42849,#42850,#42851,#42852,#42853,#42854,#42855,#42856,#42857,#42858,#42859,
#42860,#42861,#42862,#42863,#42864,#42865,#42866,#42867,#42868,#42869,#42870,
#42871,#42872,#42873,#42874,#42875,#42876,#42877,#42878,#42879,#42880,#42881,
#42882,#42883,#42884,#42885,#42886,#42887,#42888,#42889,#42890)),
 .UNSPECIFIED.,.F.,.F.,.F.,(4,4),(4,1,1,1,1,1,1,1,1,1,1,1,1,1,1,1,1,1,1,
1,1,1,1,1,1,1,1,1,1,1,1,1,1,1,1,1,1,1,1,1,1,1,1,1,1,1,1,1,1,1,1,1,1,1,1,
1,1,1,1,1,1,1,1,1,1,1,1,1,1,1,1,1,1,1,1,1,1,1,1,1,1,1,1,1,1,1,1,1,1,1,1,
1,1,1,1,1,1,1,1,1,1,1,1,1,1,1,1,1,1,1,1,1,1,1,1,1,1,1,1,1,1,1,1,1,1,1,1,
1,1,1,1,1,1,1,1,1,1,1,1,1,1,1,1,1,1,1,1,1,1,1,1,1,1,1,1,1,1,1,1,1,1,1,1,
1,1,1,1,1,1,1,1,1,1,1,1,1,1,1,1,1,1,4),(0.,0.0262983047615874),(13.0216803321501,
14.0189616954093,15.0162430586686,16.0135244219278,17.010805785187,18.0080871484463,
19.0053685117055,20.0026498749647,20.999931238224,21.9972126014832,22.9944939647424,
23.9917753280017,24.9890566912609,25.9863380545202,26.9836194177794,27.9809007810386,
28.9781821442979,29.9754635075571,30.9727448708163,31.9700262340756,32.9673075973348,
33.9645889605941,34.9618703238533,35.9591516871125,36.9564330503718,37.953714413631,
38.9509957768902,39.9482771401495,40.9455585034087,41.942839866668,42.9401212299272,
43.9374025931864,44.9346839564457,45.9319653197049,46.9292466829641,47.9265280462234,
48.9238094094826,49.9210907727419,50.9183721360011,51.9156534992603,52.9129348625196,
53.9102162257788,54.907497589038,55.9047789522973,56.9020603155565,57.8993416788158,
58.896623042075,59.8939044053342,60.8911857685935,61.8884671318527,62.8857484951119,
63.8830298583712,64.8803112216304,65.8775925848897,66.8748739481489,67.8721553114081,
68.8694366746674,69.8667180379266,70.8639994011859,71.8612807644451,72.8585621277043,
73.8558434909636,74.8531248542228,75.850406217482,76.8476875807413,77.8449689440005,
78.8422503072597,79.839531670519,80.8368130337782,81.8340943970375,82.8313757602967,
83.8286571235559,84.8259384868152,85.8232198500744,86.8205012133336,87.8177825765929,
88.8150639398521,89.8123453031114,90.8096266663706,91.8069080296298,92.8041893928891,
93.8014707561483,94.7987521194075,95.7960334826668,96.793314845926,97.7905962091853,
98.7878775724445,99.7851589357037,100.782440298963,101.779721662222,102.777003025481,
103.774284388741,104.771565752,105.768847115259,106.766128478518,107.763409841778,
108.760691205037,109.757972568296,110.755253931555,111.752535294815,112.749816658074,
113.747098021333,114.744379384592,115.741660747852,116.738942111111,117.73622347437,
118.733504837629,119.730786200888,120.728067564148,121.725348927407,122.722630290666,
123.719911653925,124.717193017185,125.714474380444,126.711755743703,127.709037106962,
128.706318470222,129.703599833481,130.70088119674,131.698162559999,132.695443923259,
133.692725286518,134.690006649777,135.687288013036,136.684569376296,137.681850739555,
138.679132102814,139.676413466073,140.673694829332,141.670976192592,142.668257555851,
143.66553891911,144.662820282369,145.660101645629,146.657383008888,147.654664372147,
148.651945735406,149.649227098666,150.646508461925,151.643789825184,152.641071188443,
153.638352551703,154.635633914962,155.632915278221,156.63019664148,157.627478004739,
158.624759367999,159.622040731258,160.619322094517,161.616603457776,162.613884821036,
163.611166184295,164.608447547554,165.605728910813,166.603010274073,167.600291637332,
168.597573000591,169.59485436385,170.59213572711,171.589417090369,172.586698453628,
173.583979816887,174.581261180147,175.578542543406,176.575823906665,177.573105269924,
178.570386633183,179.567667996443,180.564949359702,181.562230722961,182.55951208622,
183.55679344948,184.554074812739,185.551356175998,186.548637539257,187.545918902517,
188.543200265776,189.540481629035,190.537762992294,191.535044355554,192.532325718813,
193.529607082072),.UNSPECIFIED.);
#475=B_SPLINE_SURFACE_WITH_KNOTS('',3,3,((#43016,#43017,#43018,#43019,#43020,
#43021,#43022,#43023,#43024,#43025,#43026,#43027,#43028,#43029,#43030,#43031,
#43032,#43033,#43034,#43035,#43036,#43037,#43038,#43039,#43040,#43041,#43042,
#43043,#43044,#43045,#43046,#43047,#43048,#43049,#43050,#43051,#43052,#43053,
#43054,#43055,#43056,#43057,#43058,#43059,#43060,#43061,#43062,#43063,#43064,
#43065,#43066,#43067,#43068,#43069,#43070,#43071,#43072,#43073,#43074,#43075,
#43076,#43077,#43078,#43079,#43080,#43081,#43082,#43083,#43084,#43085,#43086,
#43087,#43088,#43089,#43090,#43091,#43092,#43093,#43094,#43095,#43096,#43097,
#43098,#43099,#43100,#43101,#43102,#43103,#43104,#43105,#43106,#43107,#43108,
#43109,#43110,#43111,#43112,#43113,#43114,#43115,#43116,#43117,#43118,#43119,
#43120,#43121,#43122,#43123,#43124,#43125,#43126,#43127,#43128,#43129,#43130,
#43131,#43132,#43133,#43134,#43135,#43136,#43137,#43138,#43139,#43140,#43141,
#43142,#43143,#43144,#43145,#43146,#43147,#43148,#43149,#43150,#43151,#43152,
#43153,#43154,#43155,#43156,#43157,#43158,#43159,#43160,#43161,#43162,#43163,
#43164,#43165,#43166,#43167,#43168,#43169,#43170,#43171,#43172,#43173,#43174,
#43175,#43176,#43177,#43178,#43179,#43180,#43181,#43182,#43183,#43184,#43185,
#43186,#43187,#43188,#43189,#43190,#43191,#43192,#43193,#43194,#43195,#43196,
#43197,#43198,#43199),(#43200,#43201,#43202,#43203,#43204,#43205,#43206,
#43207,#43208,#43209,#43210,#43211,#43212,#43213,#43214,#43215,#43216,#43217,
#43218,#43219,#43220,#43221,#43222,#43223,#43224,#43225,#43226,#43227,#43228,
#43229,#43230,#43231,#43232,#43233,#43234,#43235,#43236,#43237,#43238,#43239,
#43240,#43241,#43242,#43243,#43244,#43245,#43246,#43247,#43248,#43249,#43250,
#43251,#43252,#43253,#43254,#43255,#43256,#43257,#43258,#43259,#43260,#43261,
#43262,#43263,#43264,#43265,#43266,#43267,#43268,#43269,#43270,#43271,#43272,
#43273,#43274,#43275,#43276,#43277,#43278,#43279,#43280,#43281,#43282,#43283,
#43284,#43285,#43286,#43287,#43288,#43289,#43290,#43291,#43292,#43293,#43294,
#43295,#43296,#43297,#43298,#43299,#43300,#43301,#43302,#43303,#43304,#43305,
#43306,#43307,#43308,#43309,#43310,#43311,#43312,#43313,#43314,#43315,#43316,
#43317,#43318,#43319,#43320,#43321,#43322,#43323,#43324,#43325,#43326,#43327,
#43328,#43329,#43330,#43331,#43332,#43333,#43334,#43335,#43336,#43337,#43338,
#43339,#43340,#43341,#43342,#43343,#43344,#43345,#43346,#43347,#43348,#43349,
#43350,#43351,#43352,#43353,#43354,#43355,#43356,#43357,#43358,#43359,#43360,
#43361,#43362,#43363,#43364,#43365,#43366,#43367,#43368,#43369,#43370,#43371,
#43372,#43373,#43374,#43375,#43376,#43377,#43378,#43379,#43380,#43381,#43382,
#43383),(#43384,#43385,#43386,#43387,#43388,#43389,#43390,#43391,#43392,
#43393,#43394,#43395,#43396,#43397,#43398,#43399,#43400,#43401,#43402,#43403,
#43404,#43405,#43406,#43407,#43408,#43409,#43410,#43411,#43412,#43413,#43414,
#43415,#43416,#43417,#43418,#43419,#43420,#43421,#43422,#43423,#43424,#43425,
#43426,#43427,#43428,#43429,#43430,#43431,#43432,#43433,#43434,#43435,#43436,
#43437,#43438,#43439,#43440,#43441,#43442,#43443,#43444,#43445,#43446,#43447,
#43448,#43449,#43450,#43451,#43452,#43453,#43454,#43455,#43456,#43457,#43458,
#43459,#43460,#43461,#43462,#43463,#43464,#43465,#43466,#43467,#43468,#43469,
#43470,#43471,#43472,#43473,#43474,#43475,#43476,#43477,#43478,#43479,#43480,
#43481,#43482,#43483,#43484,#43485,#43486,#43487,#43488,#43489,#43490,#43491,
#43492,#43493,#43494,#43495,#43496,#43497,#43498,#43499,#43500,#43501,#43502,
#43503,#43504,#43505,#43506,#43507,#43508,#43509,#43510,#43511,#43512,#43513,
#43514,#43515,#43516,#43517,#43518,#43519,#43520,#43521,#43522,#43523,#43524,
#43525,#43526,#43527,#43528,#43529,#43530,#43531,#43532,#43533,#43534,#43535,
#43536,#43537,#43538,#43539,#43540,#43541,#43542,#43543,#43544,#43545,#43546,
#43547,#43548,#43549,#43550,#43551,#43552,#43553,#43554,#43555,#43556,#43557,
#43558,#43559,#43560,#43561,#43562,#43563,#43564,#43565,#43566,#43567),
(#43568,#43569,#43570,#43571,#43572,#43573,#43574,#43575,#43576,#43577,
#43578,#43579,#43580,#43581,#43582,#43583,#43584,#43585,#43586,#43587,#43588,
#43589,#43590,#43591,#43592,#43593,#43594,#43595,#43596,#43597,#43598,#43599,
#43600,#43601,#43602,#43603,#43604,#43605,#43606,#43607,#43608,#43609,#43610,
#43611,#43612,#43613,#43614,#43615,#43616,#43617,#43618,#43619,#43620,#43621,
#43622,#43623,#43624,#43625,#43626,#43627,#43628,#43629,#43630,#43631,#43632,
#43633,#43634,#43635,#43636,#43637,#43638,#43639,#43640,#43641,#43642,#43643,
#43644,#43645,#43646,#43647,#43648,#43649,#43650,#43651,#43652,#43653,#43654,
#43655,#43656,#43657,#43658,#43659,#43660,#43661,#43662,#43663,#43664,#43665,
#43666,#43667,#43668,#43669,#43670,#43671,#43672,#43673,#43674,#43675,#43676,
#43677,#43678,#43679,#43680,#43681,#43682,#43683,#43684,#43685,#43686,#43687,
#43688,#43689,#43690,#43691,#43692,#43693,#43694,#43695,#43696,#43697,#43698,
#43699,#43700,#43701,#43702,#43703,#43704,#43705,#43706,#43707,#43708,#43709,
#43710,#43711,#43712,#43713,#43714,#43715,#43716,#43717,#43718,#43719,#43720,
#43721,#43722,#43723,#43724,#43725,#43726,#43727,#43728,#43729,#43730,#43731,
#43732,#43733,#43734,#43735,#43736,#43737,#43738,#43739,#43740,#43741,#43742,
#43743,#43744,#43745,#43746,#43747,#43748,#43749,#43750,#43751)),
 .UNSPECIFIED.,.F.,.F.,.F.,(4,4),(4,1,1,1,1,1,1,1,1,1,1,1,1,1,1,1,1,1,1,
1,1,1,1,1,1,1,1,1,1,1,1,1,1,1,1,1,1,1,1,1,1,1,1,1,1,1,1,1,1,1,1,1,1,1,1,
1,1,1,1,1,1,1,1,1,1,1,1,1,1,1,1,1,1,1,1,1,1,1,1,1,1,1,1,1,1,1,1,1,1,1,1,
1,1,1,1,1,1,1,1,1,1,1,1,1,1,1,1,1,1,1,1,1,1,1,1,1,1,1,1,1,1,1,1,1,1,1,1,
1,1,1,1,1,1,1,1,1,1,1,1,1,1,1,1,1,1,1,1,1,1,1,1,1,1,1,1,1,1,1,1,1,1,1,1,
1,1,1,1,1,1,1,1,1,1,1,1,1,1,1,1,1,1,4),(0.,0.0262983047615874),(16.3287821777263,
17.3260635409855,18.3233449042448,19.320626267504,20.3179076307632,21.3151889940225,
22.3124703572817,23.3097517205409,24.3070330838002,25.3043144470594,26.3015958103187,
27.2988771735779,28.2961585368371,29.2934399000964,30.2907212633556,31.2880026266148,
32.2852839898741,33.2825653531333,34.2798467163926,35.2771280796518,36.274409442911,
37.2716908061703,38.2689721694295,39.2662535326887,40.263534895948,41.2608162592072,
42.2580976224665,43.2553789857257,44.2526603489849,45.2499417122442,46.2472230755034,
47.2445044387626,48.2417858020219,49.2390671652811,50.2363485285403,51.2336298917996,
52.2309112550588,53.2281926183181,54.2254739815773,55.2227553448365,56.2200367080958,
57.217318071355,58.2145994346142,59.2118807978735,60.2091621611327,61.206443524392,
62.2037248876512,63.2010062509104,64.1982876141697,65.1955689774289,66.1928503406881,
67.1901317039474,68.1874130672066,69.1846944304658,70.1819757937251,71.1792571569843,
72.1765385202436,73.1738198835028,74.171101246762,75.1683826100213,76.1656639732805,
77.1629453365397,78.160226699799,79.1575080630582,80.1547894263174,81.1520707895767,
82.1493521528359,83.1466335160952,84.1439148793544,85.1411962426136,86.1384776058729,
87.1357589691321,88.1330403323914,89.1303216956506,90.1276030589098,91.1248844221691,
92.1221657854283,93.1194471486875,94.1167285119468,95.114009875206,96.1112912384653,
97.1085726017245,98.1058539649837,99.103135328243,100.100416691502,101.097698054761,
102.094979418021,103.09226078128,104.089542144539,105.086823507798,106.084104871058,
107.081386234317,108.078667597576,109.075948960835,110.073230324095,111.070511687354,
112.067793050613,113.065074413872,114.062355777132,115.059637140391,116.05691850365,
117.054199866909,118.051481230168,119.048762593428,120.046043956687,121.043325319946,
122.040606683205,123.037888046465,124.035169409724,125.032450772983,126.029732136242,
127.027013499502,128.024294862761,129.02157622602,130.018857589279,131.016138952539,
132.013420315798,133.010701679057,134.007983042316,135.005264405576,136.002545768835,
136.999827132094,137.997108495353,138.994389858612,139.991671221872,140.988952585131,
141.98623394839,142.983515311649,143.980796674909,144.978078038168,145.975359401427,
146.972640764686,147.969922127946,148.967203491205,149.964484854464,150.961766217723,
151.959047580983,152.956328944242,153.953610307501,154.95089167076,155.948173034019,
156.945454397279,157.942735760538,158.940017123797,159.937298487056,160.934579850316,
161.931861213575,162.929142576834,163.926423940093,164.923705303353,165.920986666612,
166.918268029871,167.91554939313,168.91283075639,169.910112119649,170.907393482908,
171.904674846167,172.901956209427,173.899237572686,174.896518935945,175.893800299204,
176.891081662463,177.888363025723,178.885644388982,179.882925752241,180.8802071155,
181.87748847876,182.874769842019,183.872051205278,184.869332568537,185.866613931797,
186.863895295056,187.861176658315,188.858458021574,189.855739384834,190.853020748093,
191.850302111352,192.847583474611,193.84486483787,194.84214620113,195.839427564389,
196.836708927648),.UNSPECIFIED.);
#568=B_SPLINE_CURVE_WITH_KNOTS('',3,(#39980,#39981,#39982,#39983,#39984,
#39985,#39986,#39987,#39988,#39989,#39990,#39991,#39992),.UNSPECIFIED.,
 .F.,.F.,(4,3,3,3,4),(-5.66236639740239,-4.98640681629618,-3.98912545303695,
-2.99184408977771,-2.0654640260217),.UNSPECIFIED.);
#569=B_SPLINE_CURVE_WITH_KNOTS('',3,(#40000,#40001,#40002,#40003,#40004,
#40005,#40006,#40007,#40008,#40009),.UNSPECIFIED.,.F.,.F.,(4,3,3,4),(0.,
0.997281363259236,1.99456272651847,2.68628293579911),.UNSPECIFIED.);
#570=B_SPLINE_CURVE_WITH_KNOTS('',3,(#40014,#40015,#40016,#40017,#40018,
#40019,#40020,#40021,#40022,#40023,#40024,#40025,#40026,#40027,#40028,#40029,
#40030,#40031,#40032,#40033,#40034,#40035),.UNSPECIFIED.,.F.,.F.,(4,3,3,
3,3,3,3,4),(-11.945551704582,-10.9700949958516,-9.97281363259237,-8.97553226933314,
-7.9782509060739,-6.98096954281466,-5.98368817955542,-5.66236639740239),
 .UNSPECIFIED.);
#571=B_SPLINE_CURVE_WITH_KNOTS('',3,(#40036,#40037,#40038,#40039,#40040,
#40041,#40042,#40043,#40044,#40045,#40046,#40047,#40048,#40049,#40050,#40051,
#40052,#40053,#40054,#40055,#40056,#40057),.UNSPECIFIED.,.F.,.F.,(4,3,3,
3,3,3,3,4),(2.68628293579911,2.99184408977771,3.98912545303695,4.98640681629619,
5.98368817955542,6.98096954281466,7.9782509060739,8.9694682429787),
 .UNSPECIFIED.);
#572=B_SPLINE_CURVE_WITH_KNOTS('',3,(#40062,#40063,#40064,#40065,#40066,
#40067,#40068,#40069,#40070,#40071,#40072,#40073,#40074,#40075,#40076,#40077,
#40078,#40079,#40080,#40081,#40082,#40083,#40084,#40085,#40086),
 .UNSPECIFIED.,.F.,.F.,(4,3,3,3,3,3,3,3,4),(-18.2287370117616,-17.9510645386663,
-16.953783175407,-15.9565018121478,-14.9592204488886,-13.9619390856293,
-12.9646577223701,-11.9673763591108,-11.945551704582),.UNSPECIFIED.);
#573=B_SPLINE_CURVE_WITH_KNOTS('',3,(#40087,#40088,#40089,#40090,#40091,
#40092,#40093,#40094,#40095,#40096,#40097,#40098,#40099,#40100,#40101,#40102,
#40103,#40104,#40105,#40106,#40107,#40108),.UNSPECIFIED.,.F.,.F.,(4,3,3,
3,3,3,3,4),(8.9694682429787,9.97281363259238,10.9700949958516,11.9673763591108,
12.9646577223701,13.9619390856293,14.9592204488886,15.2526535501583),
 .UNSPECIFIED.);
#574=B_SPLINE_CURVE_WITH_KNOTS('',3,(#40113,#40114,#40115,#40116,#40117,
#40118,#40119,#40120,#40121,#40122,#40123,#40124,#40125,#40126,#40127,#40128,
#40129,#40130,#40131,#40132,#40133,#40134),.UNSPECIFIED.,.F.,.F.,(4,3,3,
3,3,3,3,4),(-24.5119223189412,-23.9347527182217,-22.9374713549625,-21.9401899917032,
-20.942908628444,-19.9456272651847,-18.9483459019255,-18.2287370117616),
 .UNSPECIFIED.);
#575=B_SPLINE_CURVE_WITH_KNOTS('',3,(#40135,#40136,#40137,#40138,#40139,
#40140,#40141,#40142,#40143,#40144,#40145,#40146,#40147,#40148,#40149,#40150,
#40151,#40152,#40153,#40154,#40155,#40156),.UNSPECIFIED.,.F.,.F.,(4,3,3,
3,3,3,3,4),(15.2526535501583,15.9565018121478,16.953783175407,17.9510645386663,
18.9483459019255,19.9456272651847,20.942908628444,21.5358388573379),
 .UNSPECIFIED.);
#576=B_SPLINE_CURVE_WITH_KNOTS('',3,(#40161,#40162,#40163,#40164,#40165,
#40166,#40167,#40168,#40169,#40170,#40171,#40172,#40173,#40174,#40175,#40176,
#40177,#40178,#40179,#40180,#40181,#40182),.UNSPECIFIED.,.F.,.F.,(4,3,3,
3,3,3,3,4),(-30.7951076261207,-29.9184408977771,-28.9211595345179,-27.9238781712586,
-26.9265968079994,-25.9293154447402,-24.9320340814809,-24.5119223189412),
 .UNSPECIFIED.);
#577=B_SPLINE_CURVE_WITH_KNOTS('',3,(#40183,#40184,#40185,#40186,#40187,
#40188,#40189,#40190,#40191,#40192,#40193,#40194,#40195,#40196,#40197,#40198,
#40199,#40200,#40201,#40202,#40203,#40204),.UNSPECIFIED.,.F.,.F.,(4,3,3,
3,3,3,3,4),(21.5358388573379,21.9401899917032,22.9374713549625,23.9347527182217,
24.9320340814809,25.9293154447402,26.9265968079994,27.8190241645175),
 .UNSPECIFIED.);
#578=B_SPLINE_CURVE_WITH_KNOTS('',3,(#40209,#40210,#40211,#40212,#40213,
#40214,#40215,#40216,#40217,#40218,#40219,#40220,#40221,#40222,#40223,#40224,
#40225,#40226,#40227,#40228,#40229,#40230,#40231,#40232,#40233),
 .UNSPECIFIED.,.F.,.F.,(4,3,3,3,3,3,3,3,4),(-37.0782929333003,-36.8994104405918,
-35.9021290773325,-34.9048477140733,-33.9075663508141,-32.9102849875548,
-31.9130036242956,-30.9157222610364,-30.7951076261207),.UNSPECIFIED.);
#579=B_SPLINE_CURVE_WITH_KNOTS('',3,(#40234,#40235,#40236,#40237,#40238,
#40239,#40240,#40241,#40242,#40243,#40244,#40245,#40246,#40247,#40248,#40249,
#40250,#40251,#40252,#40253,#40254,#40255,#40256,#40257,#40258),
 .UNSPECIFIED.,.F.,.F.,(4,3,3,3,3,3,3,3,4),(27.8190241645175,27.9238781712587,
28.9211595345179,29.9184408977771,30.9157222610364,31.9130036242956,32.9102849875548,
33.9075663508141,34.1022094716971),.UNSPECIFIED.);
#580=B_SPLINE_CURVE_WITH_KNOTS('',3,(#40263,#40264,#40265,#40266,#40267,
#40268,#40269,#40270,#40271,#40272,#40273,#40274,#40275,#40276,#40277,#40278,
#40279,#40280,#40281,#40282,#40283,#40284),.UNSPECIFIED.,.F.,.F.,(4,3,3,
3,3,3,3,4),(-43.3614782404799,-42.8830986201472,-41.885817256888,-40.8885358936287,
-39.8912545303695,-38.8939731671102,-37.896691803851,-37.0782929333003),
 .UNSPECIFIED.);
#581=B_SPLINE_CURVE_WITH_KNOTS('',3,(#40285,#40286,#40287,#40288,#40289,
#40290,#40291,#40292,#40293,#40294,#40295,#40296,#40297,#40298,#40299,#40300,
#40301,#40302,#40303,#40304,#40305,#40306),.UNSPECIFIED.,.F.,.F.,(4,3,3,
3,3,3,3,4),(34.1022094716971,34.9048477140733,35.9021290773325,36.8994104405918,
37.896691803851,38.8939731671102,39.8912545303695,40.3853947788766),
 .UNSPECIFIED.);
#582=B_SPLINE_CURVE_WITH_KNOTS('',3,(#40311,#40312,#40313,#40314,#40315,
#40316,#40317,#40318,#40319,#40320,#40321,#40322,#40323,#40324,#40325,#40326,
#40327,#40328,#40329,#40330,#40331,#40332),.UNSPECIFIED.,.F.,.F.,(4,3,3,
3,3,3,3,4),(-49.6446635476595,-48.8667867997026,-47.8695054364434,-46.8722240731841,
-45.8749427099249,-44.8776613466657,-43.8803799834064,-43.3614782404799),
 .UNSPECIFIED.);
#583=B_SPLINE_CURVE_WITH_KNOTS('',3,(#40333,#40334,#40335,#40336,#40337,
#40338,#40339,#40340,#40341,#40342,#40343,#40344,#40345,#40346,#40347,#40348,
#40349,#40350,#40351,#40352,#40353,#40354),.UNSPECIFIED.,.F.,.F.,(4,3,3,
3,3,3,3,4),(40.3853947788766,40.8885358936287,41.885817256888,42.8830986201472,
43.8803799834064,44.8776613466657,45.8749427099249,46.6685800860562),
 .UNSPECIFIED.);
#584=B_SPLINE_CURVE_WITH_KNOTS('',3,(#40359,#40360,#40361,#40362,#40363,
#40364,#40365,#40366,#40367,#40368,#40369,#40370,#40371,#40372,#40373,#40374,
#40375,#40376,#40377,#40378,#40379,#40380,#40381,#40382,#40383),
 .UNSPECIFIED.,.F.,.F.,(4,3,3,3,3,3,3,3,4),(-55.9278488548391,-55.8477563425173,
-54.8504749792581,-53.8531936159988,-52.8559122527396,-51.8586308894803,
-50.8613495262211,-49.8640681629619,-49.6446635476595),.UNSPECIFIED.);
#585=B_SPLINE_CURVE_WITH_KNOTS('',3,(#40384,#40385,#40386,#40387,#40388,
#40389,#40390,#40391,#40392,#40393,#40394,#40395,#40396,#40397,#40398,#40399,
#40400,#40401,#40402,#40403,#40404,#40405,#40406,#40407,#40408),
 .UNSPECIFIED.,.F.,.F.,(4,3,3,3,3,3,3,3,4),(46.6685800860562,46.8722240731842,
47.8695054364434,48.8667867997026,49.8640681629619,50.8613495262211,51.8586308894803,
52.8559122527396,52.9517653932358),.UNSPECIFIED.);
#586=B_SPLINE_CURVE_WITH_KNOTS('',3,(#40413,#40414,#40415,#40416,#40417,
#40418,#40419,#40420,#40421,#40422,#40423,#40424,#40425,#40426,#40427,#40428,
#40429,#40430,#40431,#40432,#40433,#40434),.UNSPECIFIED.,.F.,.F.,(4,3,3,
3,3,3,3,4),(-62.2110341620187,-61.8314445220727,-60.8341631588134,-59.8368817955542,
-58.839600432295,-57.8423190690358,-56.8450377057765,-55.9278488548391),
 .UNSPECIFIED.);
#587=B_SPLINE_CURVE_WITH_KNOTS('',3,(#40435,#40436,#40437,#40438,#40439,
#40440,#40441,#40442,#40443,#40444,#40445,#40446,#40447,#40448,#40449,#40450,
#40451,#40452,#40453,#40454,#40455,#40456),.UNSPECIFIED.,.F.,.F.,(4,3,3,
3,3,3,3,4),(52.9517653932358,53.8531936159988,54.8504749792581,55.8477563425173,
56.8450377057765,57.8423190690358,58.839600432295,59.2349507004154),
 .UNSPECIFIED.);
#588=B_SPLINE_CURVE_WITH_KNOTS('',3,(#40461,#40462,#40463,#40464,#40465,
#40466,#40467,#40468,#40469,#40470,#40471,#40472,#40473,#40474,#40475,#40476,
#40477,#40478,#40479,#40480,#40481,#40482),.UNSPECIFIED.,.F.,.F.,(4,3,3,
3,3,3,3,4),(-68.4942194691983,-67.8151327016281,-66.8178513383689,-65.8205699751096,
-64.8232886118504,-63.8260072485912,-62.8287258853319,-62.2110341620187),
 .UNSPECIFIED.);
#589=B_SPLINE_CURVE_WITH_KNOTS('',3,(#40483,#40484,#40485,#40486,#40487,
#40488,#40489,#40490,#40491,#40492,#40493,#40494,#40495,#40496,#40497,#40498,
#40499,#40500,#40501,#40502,#40503,#40504),.UNSPECIFIED.,.F.,.F.,(4,3,3,
3,3,3,3,4),(59.2349507004154,59.8368817955542,60.8341631588135,61.8314445220727,
62.8287258853319,63.8260072485912,64.8232886118504,65.518136007595),
 .UNSPECIFIED.);
#590=B_SPLINE_CURVE_WITH_KNOTS('',3,(#40509,#40510,#40511,#40512,#40513,
#40514,#40515,#40516,#40517,#40518,#40519,#40520,#40521,#40522,#40523,#40524,
#40525,#40526,#40527,#40528,#40529,#40530),.UNSPECIFIED.,.F.,.F.,(4,3,3,
3,3,3,3,4),(-74.7774047763779,-73.7988208811836,-72.8015395179243,-71.8042581546651,
-70.8069767914058,-69.8096954281466,-68.8124140648874,-68.4942194691983),
 .UNSPECIFIED.);
#591=B_SPLINE_CURVE_WITH_KNOTS('',3,(#40531,#40532,#40533,#40534,#40535,
#40536,#40537,#40538,#40539,#40540,#40541,#40542,#40543,#40544,#40545,#40546,
#40547,#40548,#40549,#40550,#40551,#40552),.UNSPECIFIED.,.F.,.F.,(4,3,3,
3,3,3,3,4),(65.518136007595,65.8205699751097,66.8178513383689,67.8151327016281,
68.8124140648874,69.8096954281466,70.8069767914059,71.8013213147746),
 .UNSPECIFIED.);
#592=B_SPLINE_CURVE_WITH_KNOTS('',3,(#40557,#40558,#40559,#40560,#40561,
#40562,#40563,#40564,#40565,#40566,#40567,#40568,#40569,#40570,#40571,#40572,
#40573,#40574,#40575,#40576,#40577,#40578,#40579,#40580,#40581),
 .UNSPECIFIED.,.F.,.F.,(4,3,3,3,3,3,3,3,4),(-81.0605900835575,-80.7797904239982,
-79.782509060739,-78.7852276974797,-77.7879463342205,-76.7906649709613,
-75.793383607702,-74.7961022444428,-74.7774047763779),.UNSPECIFIED.);
#593=B_SPLINE_CURVE_WITH_KNOTS('',3,(#40582,#40583,#40584,#40585,#40586,
#40587,#40588,#40589,#40590,#40591,#40592,#40593,#40594,#40595,#40596,#40597,
#40598,#40599,#40600,#40601,#40602,#40603),.UNSPECIFIED.,.F.,.F.,(4,3,3,
3,3,3,3,4),(71.8013213147746,72.8015395179243,73.7988208811836,74.7961022444428,
75.793383607702,76.7906649709613,77.7879463342205,78.0845066219542),
 .UNSPECIFIED.);
#594=B_SPLINE_CURVE_WITH_KNOTS('',3,(#40608,#40609,#40610,#40611,#40612,
#40613,#40614,#40615,#40616,#40617,#40618,#40619,#40620,#40621,#40622,#40623,
#40624,#40625,#40626,#40627,#40628,#40629),.UNSPECIFIED.,.F.,.F.,(4,3,3,
3,3,3,3,4),(-87.3437753907371,-86.7634786035536,-85.7661972402944,-84.7689158770352,
-83.7716345137759,-82.7743531505167,-81.7770717872575,-81.0605900835575),
 .UNSPECIFIED.);
#595=B_SPLINE_CURVE_WITH_KNOTS('',3,(#40630,#40631,#40632,#40633,#40634,
#40635,#40636,#40637,#40638,#40639,#40640,#40641,#40642,#40643,#40644,#40645,
#40646,#40647,#40648,#40649,#40650,#40651),.UNSPECIFIED.,.F.,.F.,(4,3,3,
3,3,3,3,4),(78.0845066219542,78.7852276974798,79.782509060739,80.7797904239982,
81.7770717872575,82.7743531505167,83.7716345137759,84.3676919291338),
 .UNSPECIFIED.);
#596=B_SPLINE_CURVE_WITH_KNOTS('',3,(#40656,#40657,#40658,#40659,#40660,
#40661,#40662,#40663,#40664,#40665,#40666,#40667,#40668,#40669,#40670,#40671,
#40672,#40673,#40674,#40675,#40676,#40677),.UNSPECIFIED.,.F.,.F.,(4,3,3,
3,3,3,3,4),(-93.6269606979167,-92.7471667831091,-91.7498854198498,-90.7526040565906,
-89.7553226933313,-88.7580413300721,-87.7607599668129,-87.3437753907371),
 .UNSPECIFIED.);
#597=B_SPLINE_CURVE_WITH_KNOTS('',3,(#40678,#40679,#40680,#40681,#40682,
#40683,#40684,#40685,#40686,#40687,#40688,#40689,#40690,#40691,#40692,#40693,
#40694,#40695,#40696,#40697,#40698,#40699),.UNSPECIFIED.,.F.,.F.,(4,3,3,
3,3,3,3,4),(84.3676919291338,84.7689158770352,85.7661972402944,86.7634786035537,
87.7607599668129,88.7580413300721,89.7553226933314,90.6508772363134),
 .UNSPECIFIED.);
#598=B_SPLINE_CURVE_WITH_KNOTS('',3,(#40704,#40705,#40706,#40707,#40708,
#40709,#40710,#40711,#40712,#40713,#40714,#40715,#40716,#40717,#40718,#40719,
#40720,#40721,#40722,#40723,#40724,#40725,#40726,#40727,#40728),
 .UNSPECIFIED.,.F.,.F.,(4,3,3,3,3,3,3,3,4),(-99.9101460050962,-99.7281363259237,
-98.7308549626645,-97.7335735994052,-96.736292236146,-95.7390108728868,
-94.7417295096275,-93.7444481463683,-93.6269606979167),.UNSPECIFIED.);
#599=B_SPLINE_CURVE_WITH_KNOTS('',3,(#40729,#40730,#40731,#40732,#40733,
#40734,#40735,#40736,#40737,#40738,#40739,#40740,#40741,#40742,#40743,#40744,
#40745,#40746,#40747,#40748,#40749,#40750,#40751,#40752,#40753),
 .UNSPECIFIED.,.F.,.F.,(4,3,3,3,3,3,3,3,4),(90.6508772363134,90.7526040565906,
91.7498854198498,92.7471667831091,93.7444481463683,94.7417295096275,95.7390108728868,
96.736292236146,96.934062543493),.UNSPECIFIED.);
#600=B_SPLINE_CURVE_WITH_KNOTS('',3,(#40758,#40759,#40760,#40761,#40762,
#40763,#40764,#40765,#40766,#40767,#40768,#40769,#40770,#40771,#40772,#40773,
#40774,#40775,#40776,#40777,#40778,#40779),.UNSPECIFIED.,.F.,.F.,(4,3,3,
3,3,3,3,4),(-106.193331312276,-105.711824505479,-104.71454314222,-103.717261778961,
-102.719980415701,-101.722699052442,-100.725417689183,-99.9101460050962),
 .UNSPECIFIED.);
#601=B_SPLINE_CURVE_WITH_KNOTS('',3,(#40780,#40781,#40782,#40783,#40784,
#40785,#40786,#40787,#40788,#40789,#40790,#40791,#40792,#40793,#40794,#40795,
#40796,#40797,#40798,#40799,#40800,#40801),.UNSPECIFIED.,.F.,.F.,(4,3,3,
3,3,3,3,4),(96.934062543493,97.7335735994053,98.7308549626645,99.7281363259237,
100.725417689183,101.722699052442,102.719980415701,103.217247850673),
 .UNSPECIFIED.);
#602=B_SPLINE_CURVE_WITH_KNOTS('',3,(#40806,#40807,#40808,#40809,#40810,
#40811,#40812,#40813,#40814,#40815,#40816,#40817,#40818,#40819,#40820,#40821,
#40822,#40823,#40824,#40825,#40826,#40827),.UNSPECIFIED.,.F.,.F.,(4,3,3,
3,3,3,3,4),(-112.476516619455,-111.695512685035,-110.698231321775,-109.700949958516,
-108.703668595257,-107.706387231998,-106.709105868738,-106.193331312276),
 .UNSPECIFIED.);
#603=B_SPLINE_CURVE_WITH_KNOTS('',3,(#40828,#40829,#40830,#40831,#40832,
#40833,#40834,#40835,#40836,#40837,#40838,#40839,#40840,#40841,#40842,#40843,
#40844,#40845,#40846,#40847,#40848,#40849),.UNSPECIFIED.,.F.,.F.,(4,3,3,
3,3,3,3,4),(103.217247850673,103.717261778961,104.71454314222,105.711824505479,
106.709105868738,107.706387231998,108.703668595257,109.500433157852),
 .UNSPECIFIED.);
#604=B_SPLINE_CURVE_WITH_KNOTS('',3,(#40854,#40855,#40856,#40857,#40858,
#40859,#40860,#40861,#40862,#40863,#40864,#40865,#40866,#40867,#40868,#40869,
#40870,#40871,#40872,#40873,#40874,#40875,#40876,#40877,#40878),
 .UNSPECIFIED.,.F.,.F.,(4,3,3,3,3,3,3,3,4),(-118.759701926635,-118.676482227849,
-117.67920086459,-116.681919501331,-115.684638138071,-114.687356774812,
-113.690075411553,-112.692794048294,-112.476516619455),.UNSPECIFIED.);
#605=B_SPLINE_CURVE_WITH_KNOTS('',3,(#40879,#40880,#40881,#40882,#40883,
#40884,#40885,#40886,#40887,#40888,#40889,#40890,#40891,#40892,#40893,#40894,
#40895,#40896,#40897,#40898,#40899,#40900,#40901,#40902,#40903),
 .UNSPECIFIED.,.F.,.F.,(4,3,3,3,3,3,3,3,4),(109.500433157852,109.700949958516,
110.698231321775,111.695512685035,112.692794048294,113.690075411553,114.687356774812,
115.684638138072,115.783618465032),.UNSPECIFIED.);
#606=B_SPLINE_CURVE_WITH_KNOTS('',3,(#40908,#40909,#40910,#40911,#40912,
#40913,#40914,#40915,#40916,#40917,#40918,#40919,#40920,#40921,#40922,#40923,
#40924,#40925,#40926,#40927,#40928,#40929),.UNSPECIFIED.,.F.,.F.,(4,3,3,
3,3,3,3,4),(-125.042887233815,-124.660170407405,-123.662889044145,-122.665607680886,
-121.668326317627,-120.671044954368,-119.673763591108,-118.759701926635),
 .UNSPECIFIED.);
#607=B_SPLINE_CURVE_WITH_KNOTS('',3,(#40930,#40931,#40932,#40933,#40934,
#40935,#40936,#40937,#40938,#40939,#40940,#40941,#40942,#40943,#40944,#40945,
#40946,#40947,#40948,#40949,#40950,#40951),.UNSPECIFIED.,.F.,.F.,(4,3,3,
3,3,3,3,4),(115.783618465032,116.681919501331,117.67920086459,118.676482227849,
119.673763591108,120.671044954368,121.668326317627,122.066803772211),
 .UNSPECIFIED.);
#608=B_SPLINE_CURVE_WITH_KNOTS('',3,(#40956,#40957,#40958,#40959,#40960,
#40961,#40962,#40963,#40964,#40965,#40966,#40967,#40968,#40969,#40970,#40971,
#40972,#40973,#40974,#40975,#40976,#40977),.UNSPECIFIED.,.F.,.F.,(4,3,3,
3,3,3,3,4),(-131.326072540994,-130.64385858696,-129.646577223701,-128.649295860442,
-127.652014497182,-126.654733133923,-125.657451770664,-125.042887233815),
 .UNSPECIFIED.);
#609=B_SPLINE_CURVE_WITH_KNOTS('',3,(#40978,#40979,#40980,#40981,#40982,
#40983,#40984,#40985,#40986,#40987,#40988,#40989,#40990,#40991,#40992,#40993,
#40994,#40995,#40996,#40997,#40998,#40999),.UNSPECIFIED.,.F.,.F.,(4,3,3,
3,3,3,3,4),(122.066803772211,122.665607680886,123.662889044145,124.660170407405,
125.657451770664,126.654733133923,127.652014497182,128.349989079391),
 .UNSPECIFIED.);
#610=B_SPLINE_CURVE_WITH_KNOTS('',3,(#41004,#41005,#41006,#41007,#41008,
#41009,#41010,#41011,#41012,#41013,#41014,#41015,#41016,#41017,#41018,#41019,
#41020,#41021,#41022,#41023,#41024,#41025),.UNSPECIFIED.,.F.,.F.,(4,3,3,
3,3,3,3,4),(-137.609257848174,-136.627546766515,-135.630265403256,-134.632984039997,
-133.635702676738,-132.638421313479,-131.641139950219,-131.326072540994),
 .UNSPECIFIED.);
#611=B_SPLINE_CURVE_WITH_KNOTS('',3,(#41026,#41027,#41028,#41029,#41030,
#41031,#41032,#41033,#41034,#41035,#41036,#41037,#41038,#41039,#41040,#41041,
#41042,#41043,#41044,#41045,#41046,#41047),.UNSPECIFIED.,.F.,.F.,(4,3,3,
3,3,3,3,4),(128.349989079391,128.649295860442,129.646577223701,130.64385858696,
131.641139950219,132.638421313479,133.635702676738,134.633174386571),
 .UNSPECIFIED.);
#612=B_SPLINE_CURVE_WITH_KNOTS('',3,(#41052,#41053,#41054,#41055,#41056,
#41057,#41058,#41059,#41060,#41061,#41062,#41063,#41064,#41065,#41066,#41067,
#41068,#41069,#41070,#41071,#41072,#41073,#41074,#41075,#41076),
 .UNSPECIFIED.,.F.,.F.,(4,3,3,3,3,3,3,3,4),(-143.892443155353,-143.60851630933,
-142.611234946071,-141.613953582812,-140.616672219552,-139.619390856293,
-138.622109493034,-137.624828129775,-137.609257848174),.UNSPECIFIED.);
#613=B_SPLINE_CURVE_WITH_KNOTS('',3,(#41077,#41078,#41079,#41080,#41081,
#41082,#41083,#41084,#41085,#41086,#41087,#41088,#41089,#41090,#41091,#41092,
#41093,#41094,#41095,#41096,#41097,#41098),.UNSPECIFIED.,.F.,.F.,(4,3,3,
3,3,3,3,4),(134.633174386571,135.630265403256,136.627546766516,137.624828129775,
138.622109493034,139.619390856293,140.616672219552,140.91635969375),
 .UNSPECIFIED.);
#614=B_SPLINE_CURVE_WITH_KNOTS('',3,(#41103,#41104,#41105,#41106,#41107,
#41108,#41109,#41110,#41111,#41112,#41113,#41114,#41115,#41116,#41117,#41118,
#41119,#41120,#41121,#41122,#41123,#41124),.UNSPECIFIED.,.F.,.F.,(4,3,3,
3,3,3,3,4),(-150.175628462533,-149.592204488886,-148.594923125626,-147.597641762367,
-146.600360399108,-145.603079035849,-144.605797672589,-143.892443155353),
 .UNSPECIFIED.);
#615=B_SPLINE_CURVE_WITH_KNOTS('',3,(#41125,#41126,#41127,#41128,#41129,
#41130,#41131,#41132,#41133,#41134,#41135,#41136,#41137,#41138,#41139,#41140,
#41141,#41142,#41143,#41144,#41145,#41146),.UNSPECIFIED.,.F.,.F.,(4,3,3,
3,3,3,3,4),(140.91635969375,141.613953582812,142.611234946071,143.60851630933,
144.605797672589,145.603079035849,146.600360399108,147.19954500093),
 .UNSPECIFIED.);
#616=B_SPLINE_CURVE_WITH_KNOTS('',3,(#41151,#41152,#41153,#41154,#41155,
#41156,#41157,#41158,#41159,#41160,#41161,#41162,#41163,#41164,#41165,#41166,
#41167,#41168,#41169,#41170,#41171,#41172),.UNSPECIFIED.,.F.,.F.,(4,3,3,
3,3,3,3,4),(-156.458813769712,-155.575892668441,-154.578611305182,-153.581329941923,
-152.584048578663,-151.586767215404,-150.589485852145,-150.175628462533),
 .UNSPECIFIED.);
#617=B_SPLINE_CURVE_WITH_KNOTS('',3,(#41173,#41174,#41175,#41176,#41177,
#41178,#41179,#41180,#41181,#41182,#41183,#41184,#41185,#41186,#41187,#41188,
#41189,#41190,#41191,#41192,#41193,#41194),.UNSPECIFIED.,.F.,.F.,(4,3,3,
3,3,3,3,4),(147.19954500093,147.597641762367,148.594923125626,149.592204488886,
150.589485852145,151.586767215404,152.584048578663,153.482730308109),
 .UNSPECIFIED.);
#618=B_SPLINE_CURVE_WITH_KNOTS('',3,(#41199,#41200,#41201,#41202,#41203,
#41204,#41205,#41206,#41207,#41208,#41209,#41210,#41211,#41212,#41213,#41214,
#41215,#41216,#41217,#41218,#41219,#41220,#41221,#41222,#41223),
 .UNSPECIFIED.,.F.,.F.,(4,3,3,3,3,3,3,3,4),(-162.741999076892,-162.556862211256,
-161.559580847996,-160.562299484737,-159.565018121478,-158.567736758219,
-157.570455394959,-156.5731740317,-156.458813769712),.UNSPECIFIED.);
#619=B_SPLINE_CURVE_WITH_KNOTS('',3,(#41224,#41225,#41226,#41227,#41228,
#41229,#41230,#41231,#41232,#41233,#41234,#41235,#41236,#41237,#41238,#41239,
#41240,#41241,#41242,#41243,#41244,#41245,#41246,#41247,#41248),
 .UNSPECIFIED.,.F.,.F.,(4,3,3,3,3,3,3,3,4),(153.482730308109,153.581329941923,
154.578611305182,155.575892668441,156.5731740317,157.57045539496,158.567736758219,
159.565018121478,159.765915615289),.UNSPECIFIED.);
#620=B_SPLINE_CURVE_WITH_KNOTS('',3,(#41253,#41254,#41255,#41256,#41257,
#41258,#41259,#41260,#41261,#41262,#41263,#41264,#41265,#41266,#41267,#41268,
#41269,#41270,#41271,#41272,#41273,#41274),.UNSPECIFIED.,.F.,.F.,(4,3,3,
3,3,3,3,4),(-169.025184384072,-168.540550390811,-167.543269027552,-166.545987664293,
-165.548706301033,-164.551424937774,-163.554143574515,-162.741999076892),
 .UNSPECIFIED.);
#621=B_SPLINE_CURVE_WITH_KNOTS('',3,(#41275,#41276,#41277,#41278,#41279,
#41280,#41281,#41282,#41283,#41284,#41285,#41286,#41287,#41288,#41289,#41290,
#41291,#41292,#41293,#41294,#41295,#41296),.UNSPECIFIED.,.F.,.F.,(4,3,3,
3,3,3,3,4),(159.765915615289,160.562299484737,161.559580847996,162.556862211256,
163.554143574515,164.551424937774,165.548706301033,166.049100922468),
 .UNSPECIFIED.);
#622=B_SPLINE_CURVE_WITH_KNOTS('',3,(#41301,#41302,#41303,#41304,#41305,
#41306,#41307,#41308,#41309,#41310,#41311,#41312,#41313,#41314,#41315,#41316,
#41317,#41318,#41319,#41320,#41321,#41322),.UNSPECIFIED.,.F.,.F.,(4,3,3,
3,3,3,3,4),(-175.308369691251,-174.524238570367,-173.526957207107,-172.529675843848,
-171.532394480589,-170.53511311733,-169.53783175407,-169.025184384072),
 .UNSPECIFIED.);
#623=B_SPLINE_CURVE_WITH_KNOTS('',3,(#41323,#41324,#41325,#41326,#41327,
#41328,#41329,#41330,#41331,#41332,#41333,#41334,#41335,#41336,#41337,#41338,
#41339,#41340,#41341,#41342,#41343,#41344),.UNSPECIFIED.,.F.,.F.,(4,3,3,
3,3,3,3,4),(166.049100922468,166.545987664293,167.543269027552,168.540550390811,
169.53783175407,170.53511311733,171.532394480589,172.332286229648),
 .UNSPECIFIED.);
#624=B_SPLINE_CURVE_WITH_KNOTS('',3,(#41350,#41351,#41352,#41353,#41354,
#41355,#41356),.UNSPECIFIED.,.F.,.F.,(4,1,1,1,4),(191.637151868977,191.850302111352,
192.847583474611,193.84486483787,194.771244901626),.UNSPECIFIED.);
#625=B_SPLINE_CURVE_WITH_KNOTS('',3,(#41359,#41360,#41361,#41362,#41363),
 .UNSPECIFIED.,.F.,.F.,(4,1,4),(191.637151868977,192.532325718813,193.529607082072),
 .UNSPECIFIED.);
#626=B_SPLINE_CURVE_WITH_KNOTS('',3,(#41368,#41369,#41370,#41371,#41372,
#41373,#41374,#41375,#41376,#41377),.UNSPECIFIED.,.F.,.F.,(4,1,1,1,1,1,
1,4),(185.353966561798,185.866613931797,186.863895295056,187.861176658315,
188.858458021574,189.855739384834,190.853020748093,191.637151868977),
 .UNSPECIFIED.);
#627=B_SPLINE_CURVE_WITH_KNOTS('',3,(#41378,#41379,#41380,#41381,#41382,
#41383,#41384,#41385,#41386,#41387,#41388),.UNSPECIFIED.,.F.,.F.,(4,1,1,
1,1,1,1,1,4),(185.353966561798,185.551356175998,186.548637539257,187.545918902517,
188.543200265776,189.540481629035,190.537762992294,191.535044355554,191.637151868977),
 .UNSPECIFIED.);
#628=B_SPLINE_CURVE_WITH_KNOTS('',3,(#41393,#41394,#41395,#41396,#41397,
#41398,#41399,#41400,#41401,#41402),.UNSPECIFIED.,.F.,.F.,(4,1,1,1,1,1,
1,4),(179.070781254618,179.882925752241,180.8802071155,181.87748847876,
182.874769842019,183.872051205278,184.869332568537,185.353966561798),
 .UNSPECIFIED.);
#629=B_SPLINE_CURVE_WITH_KNOTS('',3,(#41403,#41404,#41405,#41406,#41407,
#41408,#41409,#41410,#41411,#41412),.UNSPECIFIED.,.F.,.F.,(4,1,1,1,1,1,
1,4),(179.070781254618,179.567667996443,180.564949359702,181.562230722961,
182.55951208622,183.55679344948,184.554074812739,185.353966561798),
 .UNSPECIFIED.);
#630=B_SPLINE_CURVE_WITH_KNOTS('',3,(#41417,#41418,#41419,#41420,#41421,
#41422,#41423,#41424,#41425,#41426,#41427),.UNSPECIFIED.,.F.,.F.,(4,1,1,
1,1,1,1,1,4),(172.787595947439,172.901956209427,173.899237572686,174.896518935945,
175.893800299204,176.891081662463,177.888363025723,178.885644388982,179.070781254618),
 .UNSPECIFIED.);
#631=B_SPLINE_CURVE_WITH_KNOTS('',3,(#41428,#41429,#41430,#41431,#41432,
#41433,#41434,#41435,#41436,#41437),.UNSPECIFIED.,.F.,.F.,(4,1,1,1,1,1,
1,4),(172.787595947439,173.583979816887,174.581261180147,175.578542543406,
176.575823906665,177.573105269924,178.570386633183,179.070781254618),
 .UNSPECIFIED.);
#632=B_SPLINE_CURVE_WITH_KNOTS('',3,(#41442,#41443,#41444,#41445,#41446,
#41447,#41448,#41449,#41450,#41451),.UNSPECIFIED.,.F.,.F.,(4,1,1,1,1,1,
1,4),(166.504410640259,166.918268029871,167.91554939313,168.91283075639,
169.910112119649,170.907393482908,171.904674846167,172.787595947439),
 .UNSPECIFIED.);
#633=B_SPLINE_CURVE_WITH_KNOTS('',3,(#41452,#41453,#41454,#41455,#41456,
#41457,#41458,#41459,#41460,#41461,#41462),.UNSPECIFIED.,.F.,.F.,(4,1,1,
1,1,1,1,1,4),(166.504410640259,166.603010274073,167.600291637332,168.597573000591,
169.59485436385,170.59213572711,171.589417090369,172.586698453628,172.787595947439),
 .UNSPECIFIED.);
#634=B_SPLINE_CURVE_WITH_KNOTS('',3,(#41467,#41468,#41469,#41470,#41471,
#41472,#41473,#41474,#41475,#41476),.UNSPECIFIED.,.F.,.F.,(4,1,1,1,1,1,
1,4),(160.22122533308,160.934579850316,161.931861213575,162.929142576834,
163.926423940093,164.923705303353,165.920986666612,166.504410640259),
 .UNSPECIFIED.);
#635=B_SPLINE_CURVE_WITH_KNOTS('',3,(#41477,#41478,#41479,#41480,#41481,
#41482,#41483,#41484,#41485,#41486),.UNSPECIFIED.,.F.,.F.,(4,1,1,1,1,1,
1,4),(160.22122533308,160.619322094517,161.616603457776,162.613884821036,
163.611166184295,164.608447547554,165.605728910813,166.504410640259),
 .UNSPECIFIED.);
#636=B_SPLINE_CURVE_WITH_KNOTS('',3,(#41491,#41492,#41493,#41494,#41495,
#41496,#41497,#41498,#41499,#41500,#41501),.UNSPECIFIED.,.F.,.F.,(4,1,1,
1,1,1,1,1,4),(153.9380400259,153.953610307501,154.95089167076,155.948173034019,
156.945454397279,157.942735760538,158.940017123797,159.937298487056,160.22122533308),
 .UNSPECIFIED.);
#637=B_SPLINE_CURVE_WITH_KNOTS('',3,(#41502,#41503,#41504,#41505,#41506,
#41507,#41508,#41509,#41510,#41511),.UNSPECIFIED.,.F.,.F.,(4,1,1,1,1,1,
1,4),(153.9380400259,154.635633914962,155.632915278221,156.63019664148,
157.627478004739,158.624759367999,159.622040731258,160.22122533308),
 .UNSPECIFIED.);
#638=B_SPLINE_CURVE_WITH_KNOTS('',3,(#41516,#41517,#41518,#41519,#41520,
#41521,#41522,#41523,#41524,#41525),.UNSPECIFIED.,.F.,.F.,(4,1,1,1,1,1,
1,4),(147.65485471872,147.969922127946,148.967203491205,149.964484854464,
150.961766217723,151.959047580983,152.956328944242,153.9380400259),
 .UNSPECIFIED.);
#639=B_SPLINE_CURVE_WITH_KNOTS('',3,(#41526,#41527,#41528,#41529,#41530,
#41531,#41532,#41533,#41534,#41535),.UNSPECIFIED.,.F.,.F.,(4,1,1,1,1,1,
1,4),(147.65485471872,148.651945735406,149.649227098666,150.646508461925,
151.643789825184,152.641071188443,153.638352551703,153.9380400259),
 .UNSPECIFIED.);
#640=B_SPLINE_CURVE_WITH_KNOTS('',3,(#41540,#41541,#41542,#41543,#41544,
#41545,#41546,#41547,#41548,#41549),.UNSPECIFIED.,.F.,.F.,(4,1,1,1,1,1,
1,4),(141.371669411541,141.98623394839,142.983515311649,143.980796674909,
144.978078038168,145.975359401427,146.972640764686,147.65485471872),
 .UNSPECIFIED.);
#641=B_SPLINE_CURVE_WITH_KNOTS('',3,(#41550,#41551,#41552,#41553,#41554,
#41555,#41556,#41557,#41558,#41559,#41560),.UNSPECIFIED.,.F.,.F.,(4,1,1,
1,1,1,1,1,4),(141.371669411541,141.670976192592,142.668257555851,143.66553891911,
144.662820282369,145.660101645629,146.657383008888,147.654664372147,147.65485471872),
 .UNSPECIFIED.);
#642=B_SPLINE_CURVE_WITH_KNOTS('',3,(#41565,#41566,#41567,#41568,#41569,
#41570,#41571,#41572,#41573,#41574),.UNSPECIFIED.,.F.,.F.,(4,1,1,1,1,1,
1,4),(135.088484104361,136.002545768835,136.999827132094,137.997108495353,
138.994389858612,139.991671221872,140.988952585131,141.371669411541),
 .UNSPECIFIED.);
#643=B_SPLINE_CURVE_WITH_KNOTS('',3,(#41575,#41576,#41577,#41578,#41579,
#41580,#41581,#41582,#41583,#41584),.UNSPECIFIED.,.F.,.F.,(4,1,1,1,1,1,
1,4),(135.088484104361,135.687288013036,136.684569376296,137.681850739555,
138.679132102814,139.676413466073,140.673694829332,141.371669411541),
 .UNSPECIFIED.);
#644=B_SPLINE_CURVE_WITH_KNOTS('',3,(#41589,#41590,#41591,#41592,#41593,
#41594,#41595,#41596,#41597,#41598,#41599),.UNSPECIFIED.,.F.,.F.,(4,1,1,
1,1,1,1,1,4),(128.805298797182,129.02157622602,130.018857589279,131.016138952539,
132.013420315798,133.010701679057,134.007983042316,135.005264405576,135.088484104361),
 .UNSPECIFIED.);
#645=B_SPLINE_CURVE_WITH_KNOTS('',3,(#41600,#41601,#41602,#41603,#41604,
#41605,#41606,#41607,#41608,#41609),.UNSPECIFIED.,.F.,.F.,(4,1,1,1,1,1,
1,4),(128.805298797182,129.703599833481,130.70088119674,131.698162559999,
132.695443923259,133.692725286518,134.690006649777,135.088484104361),
 .UNSPECIFIED.);
#646=B_SPLINE_CURVE_WITH_KNOTS('',3,(#41614,#41615,#41616,#41617,#41618,
#41619,#41620,#41621,#41622,#41623),.UNSPECIFIED.,.F.,.F.,(4,1,1,1,1,1,
1,4),(122.522113490002,123.037888046465,124.035169409724,125.032450772983,
126.029732136242,127.027013499502,128.024294862761,128.805298797182),
 .UNSPECIFIED.);
#647=B_SPLINE_CURVE_WITH_KNOTS('',3,(#41624,#41625,#41626,#41627,#41628,
#41629,#41630,#41631,#41632,#41633,#41634),.UNSPECIFIED.,.F.,.F.,(4,1,1,
1,1,1,1,1,4),(122.522113490002,122.722630290666,123.719911653925,124.717193017185,
125.714474380444,126.711755743703,127.709037106962,128.706318470222,128.805298797182),
 .UNSPECIFIED.);
#648=B_SPLINE_CURVE_WITH_KNOTS('',3,(#41639,#41640,#41641,#41642,#41643,
#41644,#41645,#41646,#41647,#41648),.UNSPECIFIED.,.F.,.F.,(4,1,1,1,1,1,
1,4),(116.238928182823,117.054199866909,118.051481230168,119.048762593428,
120.046043956687,121.043325319946,122.040606683205,122.522113490002),
 .UNSPECIFIED.);
#649=B_SPLINE_CURVE_WITH_KNOTS('',3,(#41649,#41650,#41651,#41652,#41653,
#41654,#41655,#41656,#41657,#41658),.UNSPECIFIED.,.F.,.F.,(4,1,1,1,1,1,
1,4),(116.238928182823,116.738942111111,117.73622347437,118.733504837629,
119.730786200888,120.728067564148,121.725348927407,122.522113490002),
 .UNSPECIFIED.);
#650=B_SPLINE_CURVE_WITH_KNOTS('',3,(#41663,#41664,#41665,#41666,#41667,
#41668,#41669,#41670,#41671,#41672,#41673),.UNSPECIFIED.,.F.,.F.,(4,1,1,
1,1,1,1,1,4),(109.955742875643,110.073230324095,111.070511687354,112.067793050613,
113.065074413872,114.062355777132,115.059637140391,116.05691850365,116.238928182823),
 .UNSPECIFIED.);
#651=B_SPLINE_CURVE_WITH_KNOTS('',3,(#41674,#41675,#41676,#41677,#41678,
#41679,#41680,#41681,#41682,#41683),.UNSPECIFIED.,.F.,.F.,(4,1,1,1,1,1,
1,4),(109.955742875643,110.755253931555,111.752535294815,112.749816658074,
113.747098021333,114.744379384592,115.741660747852,116.238928182823),
 .UNSPECIFIED.);
#652=B_SPLINE_CURVE_WITH_KNOTS('',3,(#41688,#41689,#41690,#41691,#41692,
#41693,#41694,#41695,#41696,#41697),.UNSPECIFIED.,.F.,.F.,(4,1,1,1,1,1,
1,4),(103.672557568463,104.089542144539,105.086823507798,106.084104871058,
107.081386234317,108.078667597576,109.075948960835,109.955742875643),
 .UNSPECIFIED.);
#653=B_SPLINE_CURVE_WITH_KNOTS('',3,(#41698,#41699,#41700,#41701,#41702,
#41703,#41704,#41705,#41706,#41707,#41708),.UNSPECIFIED.,.F.,.F.,(4,1,1,
1,1,1,1,1,4),(103.672557568463,103.774284388741,104.771565752,105.768847115259,
106.766128478518,107.763409841778,108.760691205037,109.757972568296,109.955742875643),
 .UNSPECIFIED.);
#654=B_SPLINE_CURVE_WITH_KNOTS('',3,(#41713,#41714,#41715,#41716,#41717,
#41718,#41719,#41720,#41721,#41722),.UNSPECIFIED.,.F.,.F.,(4,1,1,1,1,1,
1,4),(97.3893722612837,98.1058539649837,99.103135328243,100.100416691502,
101.097698054761,102.094979418021,103.09226078128,103.672557568463),
 .UNSPECIFIED.);
#655=B_SPLINE_CURVE_WITH_KNOTS('',3,(#41723,#41724,#41725,#41726,#41727,
#41728,#41729,#41730,#41731,#41732),.UNSPECIFIED.,.F.,.F.,(4,1,1,1,1,1,
1,4),(97.3893722612838,97.7905962091853,98.7878775724445,99.7851589357037,
100.782440298963,101.779721662222,102.777003025481,103.672557568463),
 .UNSPECIFIED.);
#656=B_SPLINE_CURVE_WITH_KNOTS('',3,(#41737,#41738,#41739,#41740,#41741,
#41742,#41743,#41744,#41745,#41746,#41747),.UNSPECIFIED.,.F.,.F.,(4,1,1,
1,1,1,1,1,4),(91.1061869541041,91.1248844221691,92.1221657854283,93.1194471486875,
94.1167285119468,95.114009875206,96.1112912384653,97.1085726017245,97.3893722612837),
 .UNSPECIFIED.);
#657=B_SPLINE_CURVE_WITH_KNOTS('',3,(#41748,#41749,#41750,#41751,#41752,
#41753,#41754,#41755,#41756,#41757),.UNSPECIFIED.,.F.,.F.,(4,1,1,1,1,1,
1,4),(91.1061869541042,91.8069080296298,92.8041893928891,93.8014707561483,
94.7987521194075,95.7960334826668,96.793314845926,97.3893722612838),
 .UNSPECIFIED.);
#658=B_SPLINE_CURVE_WITH_KNOTS('',3,(#41762,#41763,#41764,#41765,#41766,
#41767,#41768,#41769,#41770,#41771),.UNSPECIFIED.,.F.,.F.,(4,1,1,1,1,1,
1,4),(84.8230016469246,85.1411962426136,86.1384776058729,87.1357589691321,
88.1330403323914,89.1303216956506,90.1276030589098,91.1061869541041),
 .UNSPECIFIED.);
#659=B_SPLINE_CURVE_WITH_KNOTS('',3,(#41772,#41773,#41774,#41775,#41776,
#41777,#41778,#41779,#41780,#41781,#41782),.UNSPECIFIED.,.F.,.F.,(4,1,1,
1,1,1,1,1,4),(84.8230016469246,84.8259384868152,85.8232198500744,86.8205012133336,
87.8177825765929,88.8150639398521,89.8123453031114,90.8096266663706,91.1061869541042),
 .UNSPECIFIED.);
#660=B_SPLINE_CURVE_WITH_KNOTS('',3,(#41787,#41788,#41789,#41790,#41791,
#41792,#41793,#41794,#41795,#41796),.UNSPECIFIED.,.F.,.F.,(4,1,1,1,1,1,
1,4),(78.539816339745,79.1575080630582,80.1547894263174,81.1520707895767,
82.1493521528359,83.1466335160952,84.1439148793544,84.8230016469246),
 .UNSPECIFIED.);
#661=B_SPLINE_CURVE_WITH_KNOTS('',3,(#41797,#41798,#41799,#41800,#41801,
#41802,#41803,#41804,#41805,#41806),.UNSPECIFIED.,.F.,.F.,(4,1,1,1,1,1,
1,4),(78.539816339745,78.8422503072597,79.839531670519,80.8368130337782,
81.8340943970375,82.8313757602967,83.8286571235559,84.8230016469246),
 .UNSPECIFIED.);
#662=B_SPLINE_CURVE_WITH_KNOTS('',3,(#41811,#41812,#41813,#41814,#41815,
#41816,#41817,#41818,#41819,#41820),.UNSPECIFIED.,.F.,.F.,(4,1,1,1,1,1,
1,4),(72.2566310325654,73.1738198835028,74.171101246762,75.1683826100213,
76.1656639732805,77.1629453365397,78.160226699799,78.539816339745),
 .UNSPECIFIED.);
#663=B_SPLINE_CURVE_WITH_KNOTS('',3,(#41821,#41822,#41823,#41824,#41825,
#41826,#41827,#41828,#41829,#41830),.UNSPECIFIED.,.F.,.F.,(4,1,1,1,1,1,
1,4),(72.2566310325654,72.8585621277043,73.8558434909636,74.8531248542228,
75.850406217482,76.8476875807413,77.8449689440005,78.539816339745),
 .UNSPECIFIED.);
#664=B_SPLINE_CURVE_WITH_KNOTS('',3,(#41835,#41836,#41837,#41838,#41839,
#41840,#41841,#41842,#41843,#41844,#41845),.UNSPECIFIED.,.F.,.F.,(4,1,1,
1,1,1,1,1,4),(65.9734457253857,66.1928503406881,67.1901317039474,68.1874130672066,
69.1846944304658,70.1819757937251,71.1792571569843,72.1765385202436,72.2566310325654),
 .UNSPECIFIED.);
#665=B_SPLINE_CURVE_WITH_KNOTS('',3,(#41846,#41847,#41848,#41849,#41850,
#41851,#41852,#41853,#41854,#41855),.UNSPECIFIED.,.F.,.F.,(4,1,1,1,1,1,
1,4),(65.9734457253858,66.8748739481489,67.8721553114081,68.8694366746674,
69.8667180379266,70.8639994011859,71.8612807644451,72.2566310325654),
 .UNSPECIFIED.);
#666=B_SPLINE_CURVE_WITH_KNOTS('',3,(#41860,#41861,#41862,#41863,#41864,
#41865,#41866,#41867,#41868,#41869),.UNSPECIFIED.,.F.,.F.,(4,1,1,1,1,1,
1,4),(59.6902604182062,60.2091621611327,61.206443524392,62.2037248876512,
63.2010062509104,64.1982876141697,65.1955689774289,65.9734457253857),
 .UNSPECIFIED.);
#667=B_SPLINE_CURVE_WITH_KNOTS('',3,(#41870,#41871,#41872,#41873,#41874,
#41875,#41876,#41877,#41878,#41879,#41880),.UNSPECIFIED.,.F.,.F.,(4,1,1,
1,1,1,1,1,4),(59.6902604182062,59.8939044053342,60.8911857685935,61.8884671318527,
62.8857484951119,63.8830298583712,64.8803112216304,65.8775925848897,65.9734457253858),
 .UNSPECIFIED.);
#668=B_SPLINE_CURVE_WITH_KNOTS('',3,(#41885,#41886,#41887,#41888,#41889,
#41890,#41891,#41892,#41893,#41894),.UNSPECIFIED.,.F.,.F.,(4,1,1,1,1,1,
1,4),(53.4070751110266,54.2254739815773,55.2227553448365,56.2200367080958,
57.217318071355,58.2145994346142,59.2118807978735,59.6902604182062),
 .UNSPECIFIED.);
#669=B_SPLINE_CURVE_WITH_KNOTS('',3,(#41895,#41896,#41897,#41898,#41899,
#41900,#41901,#41902,#41903,#41904),.UNSPECIFIED.,.F.,.F.,(4,1,1,1,1,1,
1,4),(53.4070751110266,53.9102162257788,54.907497589038,55.9047789522973,
56.9020603155565,57.8993416788158,58.896623042075,59.6902604182062),
 .UNSPECIFIED.);
#670=B_SPLINE_CURVE_WITH_KNOTS('',3,(#41909,#41910,#41911,#41912,#41913,
#41914,#41915,#41916,#41917,#41918,#41919),.UNSPECIFIED.,.F.,.F.,(4,1,1,
1,1,1,1,1,4),(47.123889803847,47.2445044387626,48.2417858020219,49.2390671652811,
50.2363485285403,51.2336298917996,52.2309112550588,53.2281926183181,53.4070751110266),
 .UNSPECIFIED.);
#671=B_SPLINE_CURVE_WITH_KNOTS('',3,(#41920,#41921,#41922,#41923,#41924,
#41925,#41926,#41927,#41928,#41929),.UNSPECIFIED.,.F.,.F.,(4,1,1,1,1,1,
1,4),(47.123889803847,47.9265280462234,48.9238094094826,49.9210907727419,
50.9183721360011,51.9156534992603,52.9129348625196,53.4070751110266),
 .UNSPECIFIED.);
#672=B_SPLINE_CURVE_WITH_KNOTS('',3,(#41934,#41935,#41936,#41937,#41938,
#41939,#41940,#41941,#41942,#41943),.UNSPECIFIED.,.F.,.F.,(4,1,1,1,1,1,
1,4),(40.8407044966674,41.2608162592072,42.2580976224665,43.2553789857257,
44.2526603489849,45.2499417122442,46.2472230755034,47.123889803847),
 .UNSPECIFIED.);
#673=B_SPLINE_CURVE_WITH_KNOTS('',3,(#41944,#41945,#41946,#41947,#41948,
#41949,#41950,#41951,#41952,#41953,#41954),.UNSPECIFIED.,.F.,.F.,(4,1,1,
1,1,1,1,1,4),(40.8407044966674,40.9455585034087,41.942839866668,42.9401212299272,
43.9374025931864,44.9346839564457,45.9319653197049,46.9292466829641,47.123889803847),
 .UNSPECIFIED.);
#674=B_SPLINE_CURVE_WITH_KNOTS('',3,(#41959,#41960,#41961,#41962,#41963,
#41964,#41965,#41966,#41967,#41968),.UNSPECIFIED.,.F.,.F.,(4,1,1,1,1,1,
1,4),(34.5575191894878,35.2771280796518,36.274409442911,37.2716908061703,
38.2689721694295,39.2662535326887,40.263534895948,40.8407044966674),
 .UNSPECIFIED.);
#675=B_SPLINE_CURVE_WITH_KNOTS('',3,(#41969,#41970,#41971,#41972,#41973,
#41974,#41975,#41976,#41977,#41978),.UNSPECIFIED.,.F.,.F.,(4,1,1,1,1,1,
1,4),(34.5575191894878,34.9618703238533,35.9591516871125,36.9564330503718,
37.953714413631,38.9509957768902,39.9482771401495,40.8407044966674),
 .UNSPECIFIED.);
#676=B_SPLINE_CURVE_WITH_KNOTS('',3,(#41983,#41984,#41985,#41986,#41987,
#41988,#41989,#41990,#41991,#41992,#41993),.UNSPECIFIED.,.F.,.F.,(4,1,1,
1,1,1,1,1,4),(28.2743338823082,28.2961585368371,29.2934399000964,30.2907212633556,
31.2880026266148,32.2852839898741,33.2825653531333,34.2798467163926,34.5575191894878),
 .UNSPECIFIED.);
#677=B_SPLINE_CURVE_WITH_KNOTS('',3,(#41994,#41995,#41996,#41997,#41998,
#41999,#42000,#42001,#42002,#42003),.UNSPECIFIED.,.F.,.F.,(4,1,1,1,1,1,
1,4),(28.2743338823083,28.9781821442979,29.9754635075571,30.9727448708163,
31.9700262340756,32.9673075973348,33.9645889605941,34.5575191894878),
 .UNSPECIFIED.);
#678=B_SPLINE_CURVE_WITH_KNOTS('',3,(#42008,#42009,#42010,#42011,#42012,
#42013,#42014,#42015,#42016,#42017),.UNSPECIFIED.,.F.,.F.,(4,1,1,1,1,1,
1,4),(21.9911485751286,22.3124703572817,23.3097517205409,24.3070330838002,
25.3043144470594,26.3015958103187,27.2988771735779,28.2743338823082),
 .UNSPECIFIED.);
#679=B_SPLINE_CURVE_WITH_KNOTS('',3,(#42018,#42019,#42020,#42021,#42022,
#42023,#42024,#42025,#42026,#42027,#42028),.UNSPECIFIED.,.F.,.F.,(4,1,1,
1,1,1,1,1,4),(21.9911485751287,21.9972126014832,22.9944939647424,23.9917753280017,
24.9890566912609,25.9863380545202,26.9836194177794,27.9809007810386,28.2743338823083),
 .UNSPECIFIED.);
#680=B_SPLINE_CURVE_WITH_KNOTS('',3,(#42035,#42036,#42037,#42038,#42039,
#42040,#42041,#42042,#42043),.UNSPECIFIED.,.F.,.F.,(4,1,1,1,1,1,4),(16.3287821777263,
17.3260635409855,18.3233449042448,19.320626267504,20.3179076307632,21.3151889940225,
21.9911485751286),.UNSPECIFIED.);
#681=B_SPLINE_CURVE_WITH_KNOTS('',3,(#42044,#42045,#42046,#42047,#42048,
#42049,#42050,#42051,#42052,#42053),.UNSPECIFIED.,.F.,.F.,(4,1,1,1,1,1,
1,4),(15.7079632679491,16.0135244219278,17.010805785187,18.0080871484463,
19.0053685117055,20.0026498749647,20.999931238224,21.9911485751287),
 .UNSPECIFIED.);
#682=B_SPLINE_CURVE_WITH_KNOTS('',3,(#42056,#42057,#42058,#42059,#42060,
#42061,#42062,#42063,#42064,#42065,#42066,#42067,#42068,#42069,#42070,#42071,
#42072,#42073,#42074,#42075,#42076,#42077,#42078,#42079,#42080,#42081,#42082,
#42083,#42084,#42085,#42086,#42087,#42088,#42089,#42090,#42091,#42092,#42093,
#42094,#42095,#42096,#42097,#42098,#42099,#42100,#42101),.UNSPECIFIED.,
 .F.,.F.,(4,3,3,3,3,3,3,3,3,3,3,3,3,3,3,4),(-0.178587760439498,-0.17323124397687,
-0.160983113245847,-0.152353885869142,-0.140321204623344,-0.131822429222877,
-0.111507763274134,-0.104192183870485,-0.0920062408537154,-0.0761220460318835,
-0.066495657095031,-0.0498717428212732,-0.0376847964718908,-0.0291012278395342,
-0.00653686159787477,0.),.UNSPECIFIED.);
#683=B_SPLINE_CURVE_WITH_KNOTS('',3,(#42106,#42107,#42108,#42109,#42110,
#42111,#42112,#42113,#42114,#42115,#42116,#42117,#42118,#42119,#42120,#42121,
#42122,#42123,#42124,#42125,#42126,#42127,#42128,#42129,#42130,#42131,#42132,
#42133,#42134,#42135,#42136,#42137,#42138,#42139,#42140,#42141,#42142,#42143,
#42144,#42145,#42146,#42147,#42148,#42149,#42150,#42151,#42152,#42153,#42154),
 .UNSPECIFIED.,.F.,.F.,(4,3,3,3,3,3,3,3,3,3,3,3,3,3,3,3,4),(-0.177567088092139,
-0.170723718372817,-0.155497180017511,-0.145825010567084,-0.12979337606496,
-0.121643046295364,-0.10085906030943,-0.0933124832844217,-0.0856434724597094,
-0.0800750743234962,-0.0675594968156845,-0.0595371790067273,-0.0397284982519809,
-0.030777491864391,-0.0244620215328627,-0.00609433026311949,0.),
 .UNSPECIFIED.);
#684=B_SPLINE_CURVE_WITH_KNOTS('',3,(#42891,#42892,#42893,#42894,#42895,
#42896,#42897,#42898,#42899,#42900,#42901,#42902,#42903,#42904,#42905,#42906,
#42907,#42908,#42909,#42910,#42911,#42912),.UNSPECIFIED.,.F.,.F.,(4,3,3,
3,3,3,3,4),(172.332286229648,172.529675843848,173.526957207107,174.524238570367,
175.521519933626,176.518801296885,177.516082660144,178.4424627239),
 .UNSPECIFIED.);
#685=B_SPLINE_CURVE_WITH_KNOTS('',3,(#42914,#42915,#42916,#42917,#42918,
#42919,#42920,#42921,#42922,#42923,#42924,#42925,#42926,#42927,#42928,#42929,
#42930,#42931,#42932,#42933,#42934,#42935,#42936,#42937,#42938,#42939,#42940,
#42941,#42942,#42943,#42944,#42945,#42946,#42947,#42948,#42949,#42950,#42951,
#42952,#42953,#42954,#42955,#42956,#42957,#42958,#42959),.UNSPECIFIED.,
 .F.,.F.,(4,3,3,3,3,3,3,3,3,3,3,3,3,3,3,4),(-0.178587760439495,-0.173231243976866,
-0.160983111934104,-0.15235388586526,-0.140321196401713,-0.131822429300813,
-0.111507763491313,-0.104192184639522,-0.0920062408537155,-0.0761220434809652,
-0.0664956565909429,-0.0498717424432072,-0.0376847913304863,-0.0291012266178207,
-0.006536858955891,0.),.UNSPECIFIED.);
#686=B_SPLINE_CURVE_WITH_KNOTS('',3,(#42960,#42961,#42962,#42963),
 .UNSPECIFIED.,.F.,.F.,(4,4),(15.0871443581718,15.7079632679491),
 .UNSPECIFIED.);
#687=B_SPLINE_CURVE_WITH_KNOTS('',3,(#42965,#42966,#42967,#42968,#42969,
#42970,#42971,#42972,#42973,#42974,#42975,#42976,#42977,#42978,#42979,#42980,
#42981,#42982,#42983,#42984,#42985,#42986,#42987,#42988,#42989,#42990,#42991,
#42992,#42993,#42994,#42995,#42996,#42997,#42998,#42999,#43000,#43001,#43002,
#43003,#43004,#43005,#43006,#43007,#43008,#43009,#43010,#43011,#43012,#43013),
 .UNSPECIFIED.,.F.,.F.,(4,3,3,3,3,3,3,3,3,3,3,3,3,3,3,3,4),(-0.177567088092158,
-0.170723718372832,-0.155497179061098,-0.145825009845381,-0.129793369296123,
-0.121643042061732,-0.100859058192623,-0.0933124790575794,-0.0856434713972359,
-0.0800750743235143,-0.0675595120764577,-0.0595372059277545,-0.0397285262789718,
-0.0307775036558628,-0.0244620394540028,-0.00609435183518047,0.),
 .UNSPECIFIED.);
#688=B_SPLINE_CURVE_WITH_KNOTS('',3,(#43752,#43753,#43754,#43755,#43756,
#43757,#43758,#43759,#43760,#43761,#43762,#43763,#43764,#43765,#43766,#43767,
#43768,#43769,#43770),.UNSPECIFIED.,.F.,.F.,(4,3,3,3,3,3,4),(-180.507926749922,
-179.510645386663,-178.513364023404,-177.516082660144,-176.518801296885,
-175.521519933626,-175.308369691251),.UNSPECIFIED.);
#971=SHAPE_REPRESENTATION_RELATIONSHIP('SRR','None',#55119,#991);
#991=ADVANCED_BREP_SHAPE_REPRESENTATION('',(#1031),#54997);
#1011=STYLED_ITEM('',(#55393),#1031);
#1031=MANIFOLD_SOLID_BREP('ISO_4762_M2x12_A2',#24544);
#1263=FACE_BOUND('',#4936,.T.);
#1264=FACE_BOUND('',#4942,.T.);
#1265=FACE_BOUND('',#4944,.T.);
#1558=PLANE('',#26315);
#1559=PLANE('',#26318);
#1560=PLANE('',#26321);
#1561=PLANE('',#26323);
#1562=PLANE('',#26324);
#1563=PLANE('',#26325);
#1564=PLANE('',#26327);
#1565=PLANE('',#26328);
#1566=PLANE('',#26329);
#1567=PLANE('',#26331);
#1568=PLANE('',#26332);
#1569=PLANE('',#26333);
#1570=PLANE('',#26335);
#1571=PLANE('',#26336);
#1572=PLANE('',#26337);
#1573=PLANE('',#26339);
#1574=PLANE('',#26340);
#1575=PLANE('',#26341);
#1576=PLANE('',#26343);
#1577=PLANE('',#26344);
#1578=PLANE('',#26345);
#1579=PLANE('',#26347);
#1580=PLANE('',#26348);
#1581=PLANE('',#26349);
#1582=PLANE('',#26351);
#1583=PLANE('',#26352);
#1584=PLANE('',#26353);
#1585=PLANE('',#26355);
#1586=PLANE('',#26356);
#1587=PLANE('',#26357);
#1588=PLANE('',#26359);
#1589=PLANE('',#26360);
#1590=PLANE('',#26361);
#1591=PLANE('',#26363);
#1592=PLANE('',#26364);
#1593=PLANE('',#26365);
#1594=PLANE('',#26367);
#1595=PLANE('',#26368);
#1596=PLANE('',#26369);
#1597=PLANE('',#26371);
#1598=PLANE('',#26372);
#1599=PLANE('',#26373);
#1600=PLANE('',#26375);
#1601=PLANE('',#26376);
#1602=PLANE('',#26377);
#1603=PLANE('',#26379);
#1604=PLANE('',#26380);
#1605=PLANE('',#26381);
#1606=PLANE('',#26383);
#1607=PLANE('',#26384);
#1608=PLANE('',#26385);
#1609=PLANE('',#26387);
#1610=PLANE('',#26388);
#1611=PLANE('',#26389);
#1612=PLANE('',#26392);
#1613=PLANE('',#26393);
#1614=PLANE('',#26394);
#1615=PLANE('',#26396);
#1616=PLANE('',#26397);
#1617=PLANE('',#26398);
#1618=PLANE('',#26400);
#1619=PLANE('',#26401);
#1620=PLANE('',#26402);
#1621=PLANE('',#26404);
#1622=PLANE('',#26405);
#1623=PLANE('',#26406);
#1624=PLANE('',#26408);
#1625=PLANE('',#26409);
#1626=PLANE('',#26410);
#1627=PLANE('',#26412);
#1628=PLANE('',#26413);
#1629=PLANE('',#26414);
#1630=PLANE('',#26416);
#1631=PLANE('',#26417);
#1632=PLANE('',#26418);
#1633=PLANE('',#26420);
#1634=PLANE('',#26421);
#1635=PLANE('',#26422);
#1636=PLANE('',#26424);
#1637=PLANE('',#26425);
#1638=PLANE('',#26426);
#1639=PLANE('',#26428);
#1640=PLANE('',#26429);
#1641=PLANE('',#26430);
#1642=PLANE('',#26432);
#1643=PLANE('',#26433);
#1644=PLANE('',#26434);
#1645=PLANE('',#26436);
#1646=PLANE('',#26437);
#1647=PLANE('',#26438);
#1648=PLANE('',#26440);
#1649=PLANE('',#26441);
#1650=PLANE('',#26442);
#1651=PLANE('',#26444);
#1652=PLANE('',#26445);
#1653=PLANE('',#26446);
#1654=PLANE('',#26448);
#1655=PLANE('',#26449);
#1656=PLANE('',#26450);
#1657=PLANE('',#26452);
#1658=PLANE('',#26453);
#1659=PLANE('',#26454);
#1660=PLANE('',#26456);
#1661=PLANE('',#26457);
#1662=PLANE('',#26458);
#1663=PLANE('',#26460);
#1664=PLANE('',#26461);
#1665=PLANE('',#26501);
#1666=PLANE('',#26502);
#1667=PLANE('',#26503);
#1668=PLANE('',#26508);
#1669=PLANE('',#26509);
#1670=PLANE('',#26510);
#1671=PLANE('',#26511);
#1672=PLANE('',#26512);
#1673=PLANE('',#26513);
#1674=PLANE('',#26514);
#1675=PLANE('',#26515);
#1676=PLANE('',#26522);
#1677=PLANE('',#26523);
#2221=CYLINDRICAL_SURFACE('',#26253,0.096675);
#2222=CYLINDRICAL_SURFACE('',#26257,0.096675);
#2223=CYLINDRICAL_SURFACE('',#26258,0.096675);
#2224=CYLINDRICAL_SURFACE('',#26259,0.096675);
#2225=CYLINDRICAL_SURFACE('',#26260,0.096675);
#2226=CYLINDRICAL_SURFACE('',#26261,0.096675);
#2227=CYLINDRICAL_SURFACE('',#26262,0.096675);
#2228=CYLINDRICAL_SURFACE('',#26263,0.096675);
#2229=CYLINDRICAL_SURFACE('',#26264,0.096675);
#2230=CYLINDRICAL_SURFACE('',#26265,0.096675);
#2231=CYLINDRICAL_SURFACE('',#26266,0.096675);
#2232=CYLINDRICAL_SURFACE('',#26267,0.096675);
#2233=CYLINDRICAL_SURFACE('',#26268,0.096675);
#2234=CYLINDRICAL_SURFACE('',#26269,0.096675);
#2235=CYLINDRICAL_SURFACE('',#26270,0.096675);
#2236=CYLINDRICAL_SURFACE('',#26271,0.096675);
#2237=CYLINDRICAL_SURFACE('',#26272,0.096675);
#2238=CYLINDRICAL_SURFACE('',#26273,0.096675);
#2239=CYLINDRICAL_SURFACE('',#26274,0.096675);
#2240=CYLINDRICAL_SURFACE('',#26275,0.096675);
#2241=CYLINDRICAL_SURFACE('',#26276,0.096675);
#2242=CYLINDRICAL_SURFACE('',#26277,0.096675);
#2243=CYLINDRICAL_SURFACE('',#26278,0.096675);
#2244=CYLINDRICAL_SURFACE('',#26279,0.096675);
#2245=CYLINDRICAL_SURFACE('',#26280,0.096675);
#2246=CYLINDRICAL_SURFACE('',#26281,0.096675);
#2247=CYLINDRICAL_SURFACE('',#26282,0.096675);
#2248=CYLINDRICAL_SURFACE('',#26283,0.096675);
#2249=CYLINDRICAL_SURFACE('',#26284,0.0739);
#2250=CYLINDRICAL_SURFACE('',#26286,0.0739);
#2251=CYLINDRICAL_SURFACE('',#26287,0.0739);
#2252=CYLINDRICAL_SURFACE('',#26288,0.0739);
#2253=CYLINDRICAL_SURFACE('',#26289,0.0739);
#2254=CYLINDRICAL_SURFACE('',#26290,0.0739);
#2255=CYLINDRICAL_SURFACE('',#26291,0.0739);
#2256=CYLINDRICAL_SURFACE('',#26292,0.0739);
#2257=CYLINDRICAL_SURFACE('',#26293,0.0739);
#2258=CYLINDRICAL_SURFACE('',#26294,0.0739);
#2259=CYLINDRICAL_SURFACE('',#26295,0.0739);
#2260=CYLINDRICAL_SURFACE('',#26296,0.0739);
#2261=CYLINDRICAL_SURFACE('',#26297,0.0739);
#2262=CYLINDRICAL_SURFACE('',#26298,0.0739);
#2263=CYLINDRICAL_SURFACE('',#26299,0.0739);
#2264=CYLINDRICAL_SURFACE('',#26300,0.0739);
#2265=CYLINDRICAL_SURFACE('',#26301,0.0739);
#2266=CYLINDRICAL_SURFACE('',#26302,0.0739);
#2267=CYLINDRICAL_SURFACE('',#26303,0.0739);
#2268=CYLINDRICAL_SURFACE('',#26304,0.0739);
#2269=CYLINDRICAL_SURFACE('',#26305,0.0739);
#2270=CYLINDRICAL_SURFACE('',#26306,0.0739);
#2271=CYLINDRICAL_SURFACE('',#26307,0.0739);
#2272=CYLINDRICAL_SURFACE('',#26308,0.0739);
#2273=CYLINDRICAL_SURFACE('',#26309,0.0739);
#2274=CYLINDRICAL_SURFACE('',#26310,0.0739);
#2275=CYLINDRICAL_SURFACE('',#26311,0.0739);
#2276=CYLINDRICAL_SURFACE('',#26312,0.0739);
#2277=CYLINDRICAL_SURFACE('',#26313,0.0739);
#2278=CYLINDRICAL_SURFACE('',#26320,0.0739);
#2279=CYLINDRICAL_SURFACE('',#26462,0.19);
#2280=CYLINDRICAL_SURFACE('',#26518,0.096675);
#3165=FACE_OUTER_BOUND('',#4756,.T.);
#3166=FACE_OUTER_BOUND('',#4757,.T.);
#3167=FACE_OUTER_BOUND('',#4758,.T.);
#3168=FACE_OUTER_BOUND('',#4759,.T.);
#3169=FACE_OUTER_BOUND('',#4760,.T.);
#3170=FACE_OUTER_BOUND('',#4761,.T.);
#3171=FACE_OUTER_BOUND('',#4762,.T.);
#3172=FACE_OUTER_BOUND('',#4763,.T.);
#3173=FACE_OUTER_BOUND('',#4764,.T.);
#3174=FACE_OUTER_BOUND('',#4765,.T.);
#3175=FACE_OUTER_BOUND('',#4766,.T.);
#3176=FACE_OUTER_BOUND('',#4767,.T.);
#3177=FACE_OUTER_BOUND('',#4768,.T.);
#3178=FACE_OUTER_BOUND('',#4769,.T.);
#3179=FACE_OUTER_BOUND('',#4770,.T.);
#3180=FACE_OUTER_BOUND('',#4771,.T.);
#3181=FACE_OUTER_BOUND('',#4772,.T.);
#3182=FACE_OUTER_BOUND('',#4773,.T.);
#3183=FACE_OUTER_BOUND('',#4774,.T.);
#3184=FACE_OUTER_BOUND('',#4775,.T.);
#3185=FACE_OUTER_BOUND('',#4776,.T.);
#3186=FACE_OUTER_BOUND('',#4777,.T.);
#3187=FACE_OUTER_BOUND('',#4778,.T.);
#3188=FACE_OUTER_BOUND('',#4779,.T.);
#3189=FACE_OUTER_BOUND('',#4780,.T.);
#3190=FACE_OUTER_BOUND('',#4781,.T.);
#3191=FACE_OUTER_BOUND('',#4782,.T.);
#3192=FACE_OUTER_BOUND('',#4783,.T.);
#3193=FACE_OUTER_BOUND('',#4784,.T.);
#3194=FACE_OUTER_BOUND('',#4785,.T.);
#3195=FACE_OUTER_BOUND('',#4786,.T.);
#3196=FACE_OUTER_BOUND('',#4787,.T.);
#3197=FACE_OUTER_BOUND('',#4788,.T.);
#3198=FACE_OUTER_BOUND('',#4789,.T.);
#3199=FACE_OUTER_BOUND('',#4790,.T.);
#3200=FACE_OUTER_BOUND('',#4791,.T.);
#3201=FACE_OUTER_BOUND('',#4792,.T.);
#3202=FACE_OUTER_BOUND('',#4793,.T.);
#3203=FACE_OUTER_BOUND('',#4794,.T.);
#3204=FACE_OUTER_BOUND('',#4795,.T.);
#3205=FACE_OUTER_BOUND('',#4796,.T.);
#3206=FACE_OUTER_BOUND('',#4797,.T.);
#3207=FACE_OUTER_BOUND('',#4798,.T.);
#3208=FACE_OUTER_BOUND('',#4799,.T.);
#3209=FACE_OUTER_BOUND('',#4800,.T.);
#3210=FACE_OUTER_BOUND('',#4801,.T.);
#3211=FACE_OUTER_BOUND('',#4802,.T.);
#3212=FACE_OUTER_BOUND('',#4803,.T.);
#3213=FACE_OUTER_BOUND('',#4804,.T.);
#3214=FACE_OUTER_BOUND('',#4805,.T.);
#3215=FACE_OUTER_BOUND('',#4806,.T.);
#3216=FACE_OUTER_BOUND('',#4807,.T.);
#3217=FACE_OUTER_BOUND('',#4808,.T.);
#3218=FACE_OUTER_BOUND('',#4809,.T.);
#3219=FACE_OUTER_BOUND('',#4810,.T.);
#3220=FACE_OUTER_BOUND('',#4811,.T.);
#3221=FACE_OUTER_BOUND('',#4812,.T.);
#3222=FACE_OUTER_BOUND('',#4813,.T.);
#3223=FACE_OUTER_BOUND('',#4814,.T.);
#3224=FACE_OUTER_BOUND('',#4815,.T.);
#3225=FACE_OUTER_BOUND('',#4816,.T.);
#3226=FACE_OUTER_BOUND('',#4817,.T.);
#3227=FACE_OUTER_BOUND('',#4818,.T.);
#3228=FACE_OUTER_BOUND('',#4819,.T.);
#3229=FACE_OUTER_BOUND('',#4820,.T.);
#3230=FACE_OUTER_BOUND('',#4821,.T.);
#3231=FACE_OUTER_BOUND('',#4822,.T.);
#3232=FACE_OUTER_BOUND('',#4823,.T.);
#3233=FACE_OUTER_BOUND('',#4824,.T.);
#3234=FACE_OUTER_BOUND('',#4825,.T.);
#3235=FACE_OUTER_BOUND('',#4826,.T.);
#3236=FACE_OUTER_BOUND('',#4827,.T.);
#3237=FACE_OUTER_BOUND('',#4828,.T.);
#3238=FACE_OUTER_BOUND('',#4829,.T.);
#3239=FACE_OUTER_BOUND('',#4830,.T.);
#3240=FACE_OUTER_BOUND('',#4831,.T.);
#3241=FACE_OUTER_BOUND('',#4832,.T.);
#3242=FACE_OUTER_BOUND('',#4833,.T.);
#3243=FACE_OUTER_BOUND('',#4834,.T.);
#3244=FACE_OUTER_BOUND('',#4835,.T.);
#3245=FACE_OUTER_BOUND('',#4836,.T.);
#3246=FACE_OUTER_BOUND('',#4837,.T.);
#3247=FACE_OUTER_BOUND('',#4838,.T.);
#3248=FACE_OUTER_BOUND('',#4839,.T.);
#3249=FACE_OUTER_BOUND('',#4840,.T.);
#3250=FACE_OUTER_BOUND('',#4841,.T.);
#3251=FACE_OUTER_BOUND('',#4842,.T.);
#3252=FACE_OUTER_BOUND('',#4843,.T.);
#3253=FACE_OUTER_BOUND('',#4844,.T.);
#3254=FACE_OUTER_BOUND('',#4845,.T.);
#3255=FACE_OUTER_BOUND('',#4846,.T.);
#3256=FACE_OUTER_BOUND('',#4847,.T.);
#3257=FACE_OUTER_BOUND('',#4848,.T.);
#3258=FACE_OUTER_BOUND('',#4849,.T.);
#3259=FACE_OUTER_BOUND('',#4850,.T.);
#3260=FACE_OUTER_BOUND('',#4851,.T.);
#3261=FACE_OUTER_BOUND('',#4852,.T.);
#3262=FACE_OUTER_BOUND('',#4853,.T.);
#3263=FACE_OUTER_BOUND('',#4854,.T.);
#3264=FACE_OUTER_BOUND('',#4855,.T.);
#3265=FACE_OUTER_BOUND('',#4856,.T.);
#3266=FACE_OUTER_BOUND('',#4857,.T.);
#3267=FACE_OUTER_BOUND('',#4858,.T.);
#3268=FACE_OUTER_BOUND('',#4859,.T.);
#3269=FACE_OUTER_BOUND('',#4860,.T.);
#3270=FACE_OUTER_BOUND('',#4861,.T.);
#3271=FACE_OUTER_BOUND('',#4862,.T.);
#3272=FACE_OUTER_BOUND('',#4863,.T.);
#3273=FACE_OUTER_BOUND('',#4864,.T.);
#3274=FACE_OUTER_BOUND('',#4865,.T.);
#3275=FACE_OUTER_BOUND('',#4866,.T.);
#3276=FACE_OUTER_BOUND('',#4867,.T.);
#3277=FACE_OUTER_BOUND('',#4868,.T.);
#3278=FACE_OUTER_BOUND('',#4869,.T.);
#3279=FACE_OUTER_BOUND('',#4870,.T.);
#3280=FACE_OUTER_BOUND('',#4871,.T.);
#3281=FACE_OUTER_BOUND('',#4872,.T.);
#3282=FACE_OUTER_BOUND('',#4873,.T.);
#3283=FACE_OUTER_BOUND('',#4874,.T.);
#3284=FACE_OUTER_BOUND('',#4875,.T.);
#3285=FACE_OUTER_BOUND('',#4876,.T.);
#3286=FACE_OUTER_BOUND('',#4877,.T.);
#3287=FACE_OUTER_BOUND('',#4878,.T.);
#3288=FACE_OUTER_BOUND('',#4879,.T.);
#3289=FACE_OUTER_BOUND('',#4880,.T.);
#3290=FACE_OUTER_BOUND('',#4881,.T.);
#3291=FACE_OUTER_BOUND('',#4882,.T.);
#3292=FACE_OUTER_BOUND('',#4883,.T.);
#3293=FACE_OUTER_BOUND('',#4884,.T.);
#3294=FACE_OUTER_BOUND('',#4885,.T.);
#3295=FACE_OUTER_BOUND('',#4886,.T.);
#3296=FACE_OUTER_BOUND('',#4887,.T.);
#3297=FACE_OUTER_BOUND('',#4888,.T.);
#3298=FACE_OUTER_BOUND('',#4889,.T.);
#3299=FACE_OUTER_BOUND('',#4890,.T.);
#3300=FACE_OUTER_BOUND('',#4891,.T.);
#3301=FACE_OUTER_BOUND('',#4892,.T.);
#3302=FACE_OUTER_BOUND('',#4893,.T.);
#3303=FACE_OUTER_BOUND('',#4894,.T.);
#3304=FACE_OUTER_BOUND('',#4895,.T.);
#3305=FACE_OUTER_BOUND('',#4896,.T.);
#3306=FACE_OUTER_BOUND('',#4897,.T.);
#3307=FACE_OUTER_BOUND('',#4898,.T.);
#3308=FACE_OUTER_BOUND('',#4899,.T.);
#3309=FACE_OUTER_BOUND('',#4900,.T.);
#3310=FACE_OUTER_BOUND('',#4901,.T.);
#3311=FACE_OUTER_BOUND('',#4902,.T.);
#3312=FACE_OUTER_BOUND('',#4903,.T.);
#3313=FACE_OUTER_BOUND('',#4904,.T.);
#3314=FACE_OUTER_BOUND('',#4905,.T.);
#3315=FACE_OUTER_BOUND('',#4906,.T.);
#3316=FACE_OUTER_BOUND('',#4907,.T.);
#3317=FACE_OUTER_BOUND('',#4908,.T.);
#3318=FACE_OUTER_BOUND('',#4909,.T.);
#3319=FACE_OUTER_BOUND('',#4910,.T.);
#3320=FACE_OUTER_BOUND('',#4911,.T.);
#3321=FACE_OUTER_BOUND('',#4912,.T.);
#3322=FACE_OUTER_BOUND('',#4913,.T.);
#3323=FACE_OUTER_BOUND('',#4914,.T.);
#3324=FACE_OUTER_BOUND('',#4915,.T.);
#3325=FACE_OUTER_BOUND('',#4916,.T.);
#3326=FACE_OUTER_BOUND('',#4917,.T.);
#3327=FACE_OUTER_BOUND('',#4918,.T.);
#3328=FACE_OUTER_BOUND('',#4919,.T.);
#3329=FACE_OUTER_BOUND('',#4920,.T.);
#3330=FACE_OUTER_BOUND('',#4921,.T.);
#3331=FACE_OUTER_BOUND('',#4922,.T.);
#3332=FACE_OUTER_BOUND('',#4923,.T.);
#3333=FACE_OUTER_BOUND('',#4924,.T.);
#3334=FACE_OUTER_BOUND('',#4925,.T.);
#3335=FACE_OUTER_BOUND('',#4926,.T.);
#3336=FACE_OUTER_BOUND('',#4927,.T.);
#3337=FACE_OUTER_BOUND('',#4928,.T.);
#3338=FACE_OUTER_BOUND('',#4929,.T.);
#3339=FACE_OUTER_BOUND('',#4930,.T.);
#3340=FACE_OUTER_BOUND('',#4931,.T.);
#3341=FACE_OUTER_BOUND('',#4932,.T.);
#3342=FACE_OUTER_BOUND('',#4933,.T.);
#3343=FACE_OUTER_BOUND('',#4934,.T.);
#3344=FACE_OUTER_BOUND('',#4935,.T.);
#3345=FACE_OUTER_BOUND('',#4937,.T.);
#3346=FACE_OUTER_BOUND('',#4938,.T.);
#3347=FACE_OUTER_BOUND('',#4939,.T.);
#3348=FACE_OUTER_BOUND('',#4940,.T.);
#3349=FACE_OUTER_BOUND('',#4941,.T.);
#3350=FACE_OUTER_BOUND('',#4943,.T.);
#4756=EDGE_LOOP('',(#19448,#19449,#19450,#19451,#19452,#19453,#19454,#19455));
#4757=EDGE_LOOP('',(#19456,#19457,#19458,#19459));
#4758=EDGE_LOOP('',(#19460,#19461,#19462,#19463));
#4759=EDGE_LOOP('',(#19464,#19465,#19466,#19467));
#4760=EDGE_LOOP('',(#19468,#19469,#19470,#19471));
#4761=EDGE_LOOP('',(#19472,#19473,#19474,#19475));
#4762=EDGE_LOOP('',(#19476,#19477,#19478,#19479));
#4763=EDGE_LOOP('',(#19480,#19481,#19482,#19483));
#4764=EDGE_LOOP('',(#19484,#19485,#19486,#19487));
#4765=EDGE_LOOP('',(#19488,#19489,#19490,#19491));
#4766=EDGE_LOOP('',(#19492,#19493,#19494,#19495));
#4767=EDGE_LOOP('',(#19496,#19497,#19498,#19499));
#4768=EDGE_LOOP('',(#19500,#19501,#19502,#19503));
#4769=EDGE_LOOP('',(#19504,#19505,#19506,#19507));
#4770=EDGE_LOOP('',(#19508,#19509,#19510,#19511));
#4771=EDGE_LOOP('',(#19512,#19513,#19514,#19515));
#4772=EDGE_LOOP('',(#19516,#19517,#19518,#19519));
#4773=EDGE_LOOP('',(#19520,#19521,#19522,#19523));
#4774=EDGE_LOOP('',(#19524,#19525,#19526,#19527));
#4775=EDGE_LOOP('',(#19528,#19529,#19530,#19531));
#4776=EDGE_LOOP('',(#19532,#19533,#19534,#19535));
#4777=EDGE_LOOP('',(#19536,#19537,#19538,#19539));
#4778=EDGE_LOOP('',(#19540,#19541,#19542,#19543));
#4779=EDGE_LOOP('',(#19544,#19545,#19546,#19547));
#4780=EDGE_LOOP('',(#19548,#19549,#19550,#19551));
#4781=EDGE_LOOP('',(#19552,#19553,#19554,#19555));
#4782=EDGE_LOOP('',(#19556,#19557,#19558,#19559));
#4783=EDGE_LOOP('',(#19560,#19561,#19562,#19563));
#4784=EDGE_LOOP('',(#19564,#19565,#19566,#19567));
#4785=EDGE_LOOP('',(#19568,#19569,#19570,#19571));
#4786=EDGE_LOOP('',(#19572,#19573,#19574,#19575));
#4787=EDGE_LOOP('',(#19576,#19577,#19578,#19579));
#4788=EDGE_LOOP('',(#19580,#19581,#19582,#19583));
#4789=EDGE_LOOP('',(#19584,#19585,#19586,#19587));
#4790=EDGE_LOOP('',(#19588,#19589,#19590,#19591));
#4791=EDGE_LOOP('',(#19592,#19593,#19594,#19595));
#4792=EDGE_LOOP('',(#19596,#19597,#19598,#19599));
#4793=EDGE_LOOP('',(#19600,#19601,#19602,#19603));
#4794=EDGE_LOOP('',(#19604,#19605,#19606,#19607));
#4795=EDGE_LOOP('',(#19608,#19609,#19610,#19611));
#4796=EDGE_LOOP('',(#19612,#19613,#19614,#19615));
#4797=EDGE_LOOP('',(#19616,#19617,#19618,#19619));
#4798=EDGE_LOOP('',(#19620,#19621,#19622,#19623));
#4799=EDGE_LOOP('',(#19624,#19625,#19626,#19627));
#4800=EDGE_LOOP('',(#19628,#19629,#19630,#19631));
#4801=EDGE_LOOP('',(#19632,#19633,#19634,#19635));
#4802=EDGE_LOOP('',(#19636,#19637,#19638,#19639));
#4803=EDGE_LOOP('',(#19640,#19641,#19642,#19643));
#4804=EDGE_LOOP('',(#19644,#19645,#19646,#19647));
#4805=EDGE_LOOP('',(#19648,#19649,#19650,#19651));
#4806=EDGE_LOOP('',(#19652,#19653,#19654,#19655));
#4807=EDGE_LOOP('',(#19656,#19657,#19658,#19659));
#4808=EDGE_LOOP('',(#19660,#19661,#19662,#19663));
#4809=EDGE_LOOP('',(#19664,#19665,#19666,#19667));
#4810=EDGE_LOOP('',(#19668,#19669,#19670,#19671));
#4811=EDGE_LOOP('',(#19672,#19673,#19674,#19675));
#4812=EDGE_LOOP('',(#19676,#19677,#19678,#19679,#19680));
#4813=EDGE_LOOP('',(#19681,#19682,#19683,#19684,#19685));
#4814=EDGE_LOOP('',(#19686,#19687,#19688,#19689,#19690,#19691,#19692,#19693,
#19694,#19695,#19696,#19697,#19698,#19699,#19700,#19701,#19702,#19703,#19704,
#19705,#19706,#19707,#19708,#19709,#19710,#19711,#19712,#19713,#19714,#19715,
#19716,#19717,#19718,#19719,#19720,#19721,#19722,#19723,#19724,#19725,#19726,
#19727,#19728,#19729,#19730,#19731,#19732,#19733,#19734,#19735,#19736,#19737,
#19738,#19739,#19740,#19741,#19742,#19743,#19744,#19745,#19746));
#4815=EDGE_LOOP('',(#19747,#19748,#19749,#19750,#19751,#19752));
#4816=EDGE_LOOP('',(#19753,#19754,#19755));
#4817=EDGE_LOOP('',(#19756,#19757,#19758,#19759,#19760,#19761,#19762,#19763,
#19764,#19765,#19766,#19767,#19768,#19769,#19770,#19771,#19772,#19773,#19774,
#19775,#19776,#19777,#19778,#19779,#19780,#19781,#19782,#19783,#19784,#19785,
#19786,#19787,#19788,#19789,#19790,#19791,#19792,#19793,#19794,#19795,#19796,
#19797,#19798,#19799,#19800,#19801,#19802,#19803,#19804,#19805,#19806,#19807,
#19808,#19809,#19810,#19811,#19812,#19813,#19814,#19815));
#4818=EDGE_LOOP('',(#19816,#19817,#19818));
#4819=EDGE_LOOP('',(#19819,#19820,#19821,#19822));
#4820=EDGE_LOOP('',(#19823,#19824,#19825,#19826));
#4821=EDGE_LOOP('',(#19827,#19828,#19829));
#4822=EDGE_LOOP('',(#19830,#19831,#19832,#19833));
#4823=EDGE_LOOP('',(#19834,#19835,#19836,#19837));
#4824=EDGE_LOOP('',(#19838,#19839,#19840));
#4825=EDGE_LOOP('',(#19841,#19842,#19843,#19844));
#4826=EDGE_LOOP('',(#19845,#19846,#19847,#19848));
#4827=EDGE_LOOP('',(#19849,#19850,#19851));
#4828=EDGE_LOOP('',(#19852,#19853,#19854,#19855));
#4829=EDGE_LOOP('',(#19856,#19857,#19858,#19859));
#4830=EDGE_LOOP('',(#19860,#19861,#19862));
#4831=EDGE_LOOP('',(#19863,#19864,#19865,#19866));
#4832=EDGE_LOOP('',(#19867,#19868,#19869,#19870));
#4833=EDGE_LOOP('',(#19871,#19872,#19873));
#4834=EDGE_LOOP('',(#19874,#19875,#19876,#19877));
#4835=EDGE_LOOP('',(#19878,#19879,#19880,#19881));
#4836=EDGE_LOOP('',(#19882,#19883,#19884));
#4837=EDGE_LOOP('',(#19885,#19886,#19887,#19888));
#4838=EDGE_LOOP('',(#19889,#19890,#19891,#19892));
#4839=EDGE_LOOP('',(#19893,#19894,#19895));
#4840=EDGE_LOOP('',(#19896,#19897,#19898,#19899));
#4841=EDGE_LOOP('',(#19900,#19901,#19902,#19903));
#4842=EDGE_LOOP('',(#19904,#19905,#19906));
#4843=EDGE_LOOP('',(#19907,#19908,#19909,#19910));
#4844=EDGE_LOOP('',(#19911,#19912,#19913,#19914));
#4845=EDGE_LOOP('',(#19915,#19916,#19917));
#4846=EDGE_LOOP('',(#19918,#19919,#19920,#19921));
#4847=EDGE_LOOP('',(#19922,#19923,#19924,#19925));
#4848=EDGE_LOOP('',(#19926,#19927,#19928));
#4849=EDGE_LOOP('',(#19929,#19930,#19931,#19932));
#4850=EDGE_LOOP('',(#19933,#19934,#19935,#19936));
#4851=EDGE_LOOP('',(#19937,#19938,#19939));
#4852=EDGE_LOOP('',(#19940,#19941,#19942,#19943));
#4853=EDGE_LOOP('',(#19944,#19945,#19946,#19947));
#4854=EDGE_LOOP('',(#19948,#19949,#19950));
#4855=EDGE_LOOP('',(#19951,#19952,#19953,#19954));
#4856=EDGE_LOOP('',(#19955,#19956,#19957,#19958));
#4857=EDGE_LOOP('',(#19959,#19960,#19961));
#4858=EDGE_LOOP('',(#19962,#19963,#19964,#19965));
#4859=EDGE_LOOP('',(#19966,#19967,#19968,#19969));
#4860=EDGE_LOOP('',(#19970,#19971,#19972));
#4861=EDGE_LOOP('',(#19973,#19974,#19975,#19976));
#4862=EDGE_LOOP('',(#19977,#19978,#19979,#19980));
#4863=EDGE_LOOP('',(#19981,#19982,#19983));
#4864=EDGE_LOOP('',(#19984,#19985,#19986,#19987));
#4865=EDGE_LOOP('',(#19988,#19989,#19990,#19991));
#4866=EDGE_LOOP('',(#19992,#19993,#19994));
#4867=EDGE_LOOP('',(#19995,#19996,#19997,#19998));
#4868=EDGE_LOOP('',(#19999,#20000,#20001,#20002));
#4869=EDGE_LOOP('',(#20003,#20004,#20005,#20006));
#4870=EDGE_LOOP('',(#20007,#20008,#20009,#20010));
#4871=EDGE_LOOP('',(#20011,#20012,#20013,#20014));
#4872=EDGE_LOOP('',(#20015,#20016,#20017));
#4873=EDGE_LOOP('',(#20018,#20019,#20020,#20021));
#4874=EDGE_LOOP('',(#20022,#20023,#20024,#20025));
#4875=EDGE_LOOP('',(#20026,#20027,#20028));
#4876=EDGE_LOOP('',(#20029,#20030,#20031,#20032));
#4877=EDGE_LOOP('',(#20033,#20034,#20035,#20036));
#4878=EDGE_LOOP('',(#20037,#20038,#20039));
#4879=EDGE_LOOP('',(#20040,#20041,#20042,#20043));
#4880=EDGE_LOOP('',(#20044,#20045,#20046,#20047));
#4881=EDGE_LOOP('',(#20048,#20049,#20050));
#4882=EDGE_LOOP('',(#20051,#20052,#20053,#20054));
#4883=EDGE_LOOP('',(#20055,#20056,#20057,#20058));
#4884=EDGE_LOOP('',(#20059,#20060,#20061));
#4885=EDGE_LOOP('',(#20062,#20063,#20064,#20065));
#4886=EDGE_LOOP('',(#20066,#20067,#20068,#20069));
#4887=EDGE_LOOP('',(#20070,#20071,#20072));
#4888=EDGE_LOOP('',(#20073,#20074,#20075,#20076));
#4889=EDGE_LOOP('',(#20077,#20078,#20079,#20080));
#4890=EDGE_LOOP('',(#20081,#20082,#20083));
#4891=EDGE_LOOP('',(#20084,#20085,#20086,#20087));
#4892=EDGE_LOOP('',(#20088,#20089,#20090,#20091));
#4893=EDGE_LOOP('',(#20092,#20093,#20094));
#4894=EDGE_LOOP('',(#20095,#20096,#20097,#20098));
#4895=EDGE_LOOP('',(#20099,#20100,#20101,#20102));
#4896=EDGE_LOOP('',(#20103,#20104,#20105));
#4897=EDGE_LOOP('',(#20106,#20107,#20108,#20109));
#4898=EDGE_LOOP('',(#20110,#20111,#20112,#20113));
#4899=EDGE_LOOP('',(#20114,#20115,#20116));
#4900=EDGE_LOOP('',(#20117,#20118,#20119,#20120));
#4901=EDGE_LOOP('',(#20121,#20122,#20123,#20124));
#4902=EDGE_LOOP('',(#20125,#20126,#20127));
#4903=EDGE_LOOP('',(#20128,#20129,#20130,#20131));
#4904=EDGE_LOOP('',(#20132,#20133,#20134,#20135));
#4905=EDGE_LOOP('',(#20136,#20137,#20138));
#4906=EDGE_LOOP('',(#20139,#20140,#20141,#20142));
#4907=EDGE_LOOP('',(#20143,#20144,#20145,#20146));
#4908=EDGE_LOOP('',(#20147,#20148,#20149));
#4909=EDGE_LOOP('',(#20150,#20151,#20152,#20153));
#4910=EDGE_LOOP('',(#20154,#20155,#20156,#20157));
#4911=EDGE_LOOP('',(#20158,#20159,#20160));
#4912=EDGE_LOOP('',(#20161,#20162,#20163,#20164));
#4913=EDGE_LOOP('',(#20165,#20166,#20167,#20168));
#4914=EDGE_LOOP('',(#20169,#20170,#20171));
#4915=EDGE_LOOP('',(#20172,#20173,#20174,#20175));
#4916=EDGE_LOOP('',(#20176,#20177,#20178,#20179));
#4917=EDGE_LOOP('',(#20180,#20181,#20182));
#4918=EDGE_LOOP('',(#20183,#20184,#20185,#20186));
#4919=EDGE_LOOP('',(#20187,#20188,#20189,#20190));
#4920=EDGE_LOOP('',(#20191,#20192,#20193));
#4921=EDGE_LOOP('',(#20194,#20195,#20196,#20197));
#4922=EDGE_LOOP('',(#20198,#20199,#20200,#20201));
#4923=EDGE_LOOP('',(#20202,#20203,#20204,#20205,#20206,#20207,#20208,#20209,
#20210,#20211,#20212,#20213,#20214,#20215,#20216,#20217,#20218,#20219,#20220,
#20221,#20222,#20223,#20224,#20225,#20226,#20227,#20228,#20229,#20230,#20231,
#20232,#20233,#20234,#20235,#20236,#20237,#20238,#20239,#20240,#20241,#20242,
#20243,#20244,#20245,#20246,#20247,#20248,#20249,#20250,#20251,#20252,#20253,
#20254,#20255,#20256,#20257,#20258,#20259,#20260,#20261,#20262,#20263,#20264,
#20265,#20266,#20267,#20268,#20269,#20270,#20271,#20272,#20273,#20274,#20275,
#20276,#20277,#20278,#20279,#20280,#20281,#20282,#20283,#20284,#20285,#20286,
#20287,#20288,#20289,#20290,#20291,#20292,#20293,#20294,#20295,#20296,#20297,
#20298,#20299,#20300,#20301,#20302,#20303,#20304,#20305,#20306,#20307,#20308,
#20309,#20310,#20311,#20312,#20313,#20314,#20315,#20316,#20317,#20318,#20319,
#20320,#20321,#20322,#20323,#20324,#20325,#20326,#20327,#20328,#20329,#20330,
#20331,#20332,#20333,#20334,#20335,#20336,#20337,#20338,#20339,#20340,#20341,
#20342,#20343,#20344,#20345,#20346,#20347,#20348,#20349));
#4924=EDGE_LOOP('',(#20350,#20351,#20352,#20353));
#4925=EDGE_LOOP('',(#20354,#20355,#20356,#20357));
#4926=EDGE_LOOP('',(#20358,#20359,#20360));
#4927=EDGE_LOOP('',(#20361,#20362,#20363,#20364,#20365,#20366,#20367,#20368,
#20369,#20370,#20371,#20372,#20373,#20374,#20375,#20376,#20377,#20378,#20379,
#20380,#20381,#20382,#20383,#20384,#20385,#20386,#20387,#20388,#20389,#20390,
#20391,#20392,#20393,#20394,#20395,#20396,#20397,#20398,#20399,#20400,#20401,
#20402,#20403,#20404,#20405,#20406,#20407,#20408,#20409,#20410,#20411,#20412,
#20413,#20414,#20415,#20416,#20417,#20418,#20419,#20420,#20421,#20422,#20423,
#20424,#20425,#20426,#20427,#20428,#20429,#20430,#20431,#20432,#20433,#20434,
#20435,#20436,#20437,#20438,#20439,#20440,#20441,#20442,#20443,#20444,#20445,
#20446,#20447,#20448,#20449,#20450,#20451,#20452,#20453,#20454,#20455,#20456,
#20457,#20458,#20459,#20460,#20461,#20462,#20463,#20464,#20465,#20466,#20467,
#20468,#20469,#20470,#20471));
#4928=EDGE_LOOP('',(#20472,#20473,#20474));
#4929=EDGE_LOOP('',(#20475,#20476,#20477,#20478));
#4930=EDGE_LOOP('',(#20479,#20480,#20481,#20482));
#4931=EDGE_LOOP('',(#20483,#20484,#20485,#20486));
#4932=EDGE_LOOP('',(#20487,#20488,#20489,#20490));
#4933=EDGE_LOOP('',(#20491,#20492,#20493,#20494));
#4934=EDGE_LOOP('',(#20495,#20496,#20497,#20498));
#4935=EDGE_LOOP('',(#20499,#20500,#20501,#20502,#20503,#20504));
#4936=EDGE_LOOP('',(#20505));
#4937=EDGE_LOOP('',(#20506));
#4938=EDGE_LOOP('',(#20507,#20508,#20509,#20510));
#4939=EDGE_LOOP('',(#20511,#20512,#20513,#20514));
#4940=EDGE_LOOP('',(#20515,#20516,#20517,#20518,#20519,#20520));
#4941=EDGE_LOOP('',(#20521));
#4942=EDGE_LOOP('',(#20522));
#4943=EDGE_LOOP('',(#20523));
#4944=EDGE_LOOP('',(#20524,#20525,#20526,#20527,#20528,#20529));
#6333=LINE('',#39978,#8154);
#6334=LINE('',#39996,#8155);
#6335=LINE('',#40013,#8156);
#6336=LINE('',#40061,#8157);
#6337=LINE('',#40112,#8158);
#6338=LINE('',#40160,#8159);
#6339=LINE('',#40208,#8160);
#6340=LINE('',#40262,#8161);
#6341=LINE('',#40310,#8162);
#6342=LINE('',#40358,#8163);
#6343=LINE('',#40412,#8164);
#6344=LINE('',#40460,#8165);
#6345=LINE('',#40508,#8166);
#6346=LINE('',#40556,#8167);
#6347=LINE('',#40607,#8168);
#6348=LINE('',#40655,#8169);
#6349=LINE('',#40703,#8170);
#6350=LINE('',#40757,#8171);
#6351=LINE('',#40805,#8172);
#6352=LINE('',#40853,#8173);
#6353=LINE('',#40907,#8174);
#6354=LINE('',#40955,#8175);
#6355=LINE('',#41003,#8176);
#6356=LINE('',#41051,#8177);
#6357=LINE('',#41102,#8178);
#6358=LINE('',#41150,#8179);
#6359=LINE('',#41198,#8180);
#6360=LINE('',#41252,#8181);
#6361=LINE('',#41300,#8182);
#6362=LINE('',#41348,#8183);
#6363=LINE('',#41367,#8184);
#6364=LINE('',#41392,#8185);
#6365=LINE('',#41416,#8186);
#6366=LINE('',#41441,#8187);
#6367=LINE('',#41466,#8188);
#6368=LINE('',#41490,#8189);
#6369=LINE('',#41515,#8190);
#6370=LINE('',#41539,#8191);
#6371=LINE('',#41564,#8192);
#6372=LINE('',#41588,#8193);
#6373=LINE('',#41613,#8194);
#6374=LINE('',#41638,#8195);
#6375=LINE('',#41662,#8196);
#6376=LINE('',#41687,#8197);
#6377=LINE('',#41712,#8198);
#6378=LINE('',#41736,#8199);
#6379=LINE('',#41761,#8200);
#6380=LINE('',#41786,#8201);
#6381=LINE('',#41810,#8202);
#6382=LINE('',#41834,#8203);
#6383=LINE('',#41859,#8204);
#6384=LINE('',#41884,#8205);
#6385=LINE('',#41908,#8206);
#6386=LINE('',#41933,#8207);
#6387=LINE('',#41958,#8208);
#6388=LINE('',#41982,#8209);
#6389=LINE('',#42007,#8210);
#6390=LINE('',#42032,#8211);
#6391=LINE('',#43776,#8212);
#6392=LINE('',#43777,#8213);
#6393=LINE('',#43780,#8214);
#6394=LINE('',#43782,#8215);
#6395=LINE('',#43788,#8216);
#6396=LINE('',#43797,#8217);
#6397=LINE('',#43798,#8218);
#6398=LINE('',#43801,#8219);
#6399=LINE('',#43803,#8220);
#6400=LINE('',#43809,#8221);
#6401=LINE('',#43818,#8222);
#6402=LINE('',#43819,#8223);
#6403=LINE('',#43822,#8224);
#6404=LINE('',#43824,#8225);
#6405=LINE('',#43830,#8226);
#6406=LINE('',#43839,#8227);
#6407=LINE('',#43840,#8228);
#6408=LINE('',#43843,#8229);
#6409=LINE('',#43845,#8230);
#6410=LINE('',#43851,#8231);
#6411=LINE('',#43860,#8232);
#6412=LINE('',#43861,#8233);
#6413=LINE('',#43864,#8234);
#6414=LINE('',#43866,#8235);
#6415=LINE('',#43872,#8236);
#6416=LINE('',#43881,#8237);
#6417=LINE('',#43882,#8238);
#6418=LINE('',#43885,#8239);
#6419=LINE('',#43887,#8240);
#6420=LINE('',#43893,#8241);
#6421=LINE('',#43902,#8242);
#6422=LINE('',#43903,#8243);
#6423=LINE('',#43906,#8244);
#6424=LINE('',#43908,#8245);
#6425=LINE('',#43914,#8246);
#6426=LINE('',#43923,#8247);
#6427=LINE('',#43924,#8248);
#6428=LINE('',#43927,#8249);
#6429=LINE('',#43929,#8250);
#6430=LINE('',#43935,#8251);
#6431=LINE('',#43944,#8252);
#6432=LINE('',#43945,#8253);
#6433=LINE('',#43948,#8254);
#6434=LINE('',#43950,#8255);
#6435=LINE('',#43956,#8256);
#6436=LINE('',#43965,#8257);
#6437=LINE('',#43966,#8258);
#6438=LINE('',#43969,#8259);
#6439=LINE('',#43971,#8260);
#6440=LINE('',#43977,#8261);
#6441=LINE('',#43986,#8262);
#6442=LINE('',#43987,#8263);
#6443=LINE('',#43990,#8264);
#6444=LINE('',#43992,#8265);
#6445=LINE('',#43998,#8266);
#6446=LINE('',#44007,#8267);
#6447=LINE('',#44008,#8268);
#6448=LINE('',#44011,#8269);
#6449=LINE('',#44013,#8270);
#6450=LINE('',#44019,#8271);
#6451=LINE('',#44028,#8272);
#6452=LINE('',#44029,#8273);
#6453=LINE('',#44032,#8274);
#6454=LINE('',#44034,#8275);
#6455=LINE('',#44040,#8276);
#6456=LINE('',#44049,#8277);
#6457=LINE('',#44050,#8278);
#6458=LINE('',#44053,#8279);
#6459=LINE('',#44055,#8280);
#6460=LINE('',#44061,#8281);
#6461=LINE('',#44070,#8282);
#6462=LINE('',#44071,#8283);
#6463=LINE('',#44074,#8284);
#6464=LINE('',#44076,#8285);
#6465=LINE('',#44082,#8286);
#6466=LINE('',#44091,#8287);
#6467=LINE('',#44092,#8288);
#6468=LINE('',#44095,#8289);
#6469=LINE('',#44097,#8290);
#6470=LINE('',#44103,#8291);
#6471=LINE('',#44112,#8292);
#6472=LINE('',#44113,#8293);
#6473=LINE('',#44116,#8294);
#6474=LINE('',#44118,#8295);
#6475=LINE('',#44124,#8296);
#6476=LINE('',#44133,#8297);
#6477=LINE('',#44135,#8298);
#6478=LINE('',#44139,#8299);
#6479=LINE('',#44141,#8300);
#6480=LINE('',#44147,#8301);
#6481=LINE('',#44156,#8302);
#6482=LINE('',#44157,#8303);
#6483=LINE('',#44160,#8304);
#6484=LINE('',#44162,#8305);
#6485=LINE('',#44168,#8306);
#6486=LINE('',#44177,#8307);
#6487=LINE('',#44178,#8308);
#6488=LINE('',#44181,#8309);
#6489=LINE('',#44183,#8310);
#6490=LINE('',#44189,#8311);
#6491=LINE('',#44198,#8312);
#6492=LINE('',#44199,#8313);
#6493=LINE('',#44202,#8314);
#6494=LINE('',#44204,#8315);
#6495=LINE('',#44210,#8316);
#6496=LINE('',#44219,#8317);
#6497=LINE('',#44220,#8318);
#6498=LINE('',#44223,#8319);
#6499=LINE('',#44225,#8320);
#6500=LINE('',#44231,#8321);
#6501=LINE('',#44240,#8322);
#6502=LINE('',#44241,#8323);
#6503=LINE('',#44244,#8324);
#6504=LINE('',#44246,#8325);
#6505=LINE('',#44252,#8326);
#6506=LINE('',#44261,#8327);
#6507=LINE('',#44262,#8328);
#6508=LINE('',#44265,#8329);
#6509=LINE('',#44267,#8330);
#6510=LINE('',#44273,#8331);
#6511=LINE('',#44282,#8332);
#6512=LINE('',#44283,#8333);
#6513=LINE('',#44286,#8334);
#6514=LINE('',#44288,#8335);
#6515=LINE('',#44294,#8336);
#6516=LINE('',#44303,#8337);
#6517=LINE('',#44304,#8338);
#6518=LINE('',#44307,#8339);
#6519=LINE('',#44309,#8340);
#6520=LINE('',#44315,#8341);
#6521=LINE('',#44324,#8342);
#6522=LINE('',#44325,#8343);
#6523=LINE('',#44328,#8344);
#6524=LINE('',#44330,#8345);
#6525=LINE('',#44336,#8346);
#6526=LINE('',#44345,#8347);
#6527=LINE('',#44346,#8348);
#6528=LINE('',#44349,#8349);
#6529=LINE('',#44351,#8350);
#6530=LINE('',#44357,#8351);
#6531=LINE('',#44366,#8352);
#6532=LINE('',#44367,#8353);
#6533=LINE('',#44370,#8354);
#6534=LINE('',#44372,#8355);
#6535=LINE('',#44378,#8356);
#6536=LINE('',#44387,#8357);
#6537=LINE('',#44388,#8358);
#6538=LINE('',#44391,#8359);
#6539=LINE('',#44393,#8360);
#6540=LINE('',#44399,#8361);
#6541=LINE('',#44408,#8362);
#6542=LINE('',#44409,#8363);
#6543=LINE('',#44412,#8364);
#6544=LINE('',#44414,#8365);
#6545=LINE('',#44420,#8366);
#6546=LINE('',#44429,#8367);
#6547=LINE('',#44430,#8368);
#6548=LINE('',#44433,#8369);
#6549=LINE('',#44435,#8370);
#6550=LINE('',#44441,#8371);
#6551=LINE('',#44450,#8372);
#6552=LINE('',#44451,#8373);
#6553=LINE('',#44454,#8374);
#6554=LINE('',#44456,#8375);
#6555=LINE('',#44462,#8376);
#6556=LINE('',#44471,#8377);
#6557=LINE('',#44472,#8378);
#6558=LINE('',#44475,#8379);
#6559=LINE('',#44477,#8380);
#6560=LINE('',#44483,#8381);
#6561=LINE('',#44492,#8382);
#6562=LINE('',#44493,#8383);
#6563=LINE('',#44496,#8384);
#6564=LINE('',#44498,#8385);
#6565=LINE('',#44504,#8386);
#6566=LINE('',#44527,#8387);
#6567=LINE('',#44549,#8388);
#6568=LINE('',#44553,#8389);
#6569=LINE('',#44557,#8390);
#6570=LINE('',#44559,#8391);
#6571=LINE('',#44567,#8392);
#6572=LINE('',#44572,#8393);
#6573=LINE('',#44576,#8394);
#6574=LINE('',#44581,#8395);
#6575=LINE('',#44583,#8396);
#6576=LINE('',#44585,#8397);
#6577=LINE('',#44586,#8398);
#6578=LINE('',#44589,#8399);
#6579=LINE('',#44591,#8400);
#6580=LINE('',#44592,#8401);
#6581=LINE('',#44595,#8402);
#6582=LINE('',#44597,#8403);
#6583=LINE('',#44598,#8404);
#6584=LINE('',#44601,#8405);
#6585=LINE('',#44603,#8406);
#6586=LINE('',#44604,#8407);
#6587=LINE('',#44607,#8408);
#6588=LINE('',#44609,#8409);
#6589=LINE('',#44610,#8410);
#6590=LINE('',#44612,#8411);
#6591=LINE('',#44613,#8412);
#6592=LINE('',#44619,#8413);
#6593=LINE('',#44625,#8414);
#8154=VECTOR('',#31117,0.1);
#8155=VECTOR('',#31120,0.1);
#8156=VECTOR('',#31127,0.1);
#8157=VECTOR('',#31130,0.1);
#8158=VECTOR('',#31133,0.1);
#8159=VECTOR('',#31136,0.1);
#8160=VECTOR('',#31139,0.1);
#8161=VECTOR('',#31142,0.1);
#8162=VECTOR('',#31145,0.1);
#8163=VECTOR('',#31148,0.1);
#8164=VECTOR('',#31151,0.1);
#8165=VECTOR('',#31154,0.1);
#8166=VECTOR('',#31157,0.1);
#8167=VECTOR('',#31160,0.1);
#8168=VECTOR('',#31163,0.1);
#8169=VECTOR('',#31166,0.1);
#8170=VECTOR('',#31169,0.1);
#8171=VECTOR('',#31172,0.1);
#8172=VECTOR('',#31175,0.1);
#8173=VECTOR('',#31178,0.1);
#8174=VECTOR('',#31181,0.1);
#8175=VECTOR('',#31184,0.1);
#8176=VECTOR('',#31187,0.1);
#8177=VECTOR('',#31190,0.1);
#8178=VECTOR('',#31193,0.1);
#8179=VECTOR('',#31196,0.1);
#8180=VECTOR('',#31199,0.1);
#8181=VECTOR('',#31202,0.1);
#8182=VECTOR('',#31205,0.1);
#8183=VECTOR('',#31208,0.0739);
#8184=VECTOR('',#31213,0.0739);
#8185=VECTOR('',#31216,0.0739);
#8186=VECTOR('',#31219,0.0739);
#8187=VECTOR('',#31222,0.0739);
#8188=VECTOR('',#31225,0.0739);
#8189=VECTOR('',#31228,0.0739);
#8190=VECTOR('',#31231,0.0739);
#8191=VECTOR('',#31234,0.0739);
#8192=VECTOR('',#31237,0.0739);
#8193=VECTOR('',#31240,0.0739);
#8194=VECTOR('',#31243,0.0739);
#8195=VECTOR('',#31246,0.0739);
#8196=VECTOR('',#31249,0.0739);
#8197=VECTOR('',#31252,0.0739);
#8198=VECTOR('',#31255,0.0739);
#8199=VECTOR('',#31258,0.0739);
#8200=VECTOR('',#31261,0.0739);
#8201=VECTOR('',#31264,0.0739);
#8202=VECTOR('',#31267,0.0739);
#8203=VECTOR('',#31270,0.0739);
#8204=VECTOR('',#31273,0.0739);
#8205=VECTOR('',#31276,0.0739);
#8206=VECTOR('',#31279,0.0739);
#8207=VECTOR('',#31282,0.0739);
#8208=VECTOR('',#31285,0.0739);
#8209=VECTOR('',#31288,0.0739);
#8210=VECTOR('',#31291,0.0739);
#8211=VECTOR('',#31294,0.0739);
#8212=VECTOR('',#31313,1.);
#8213=VECTOR('',#31314,1.);
#8214=VECTOR('',#31317,1.);
#8215=VECTOR('',#31318,1.);
#8216=VECTOR('',#31321,1.);
#8217=VECTOR('',#31326,1.);
#8218=VECTOR('',#31327,1.);
#8219=VECTOR('',#31330,1.);
#8220=VECTOR('',#31331,1.);
#8221=VECTOR('',#31334,1.);
#8222=VECTOR('',#31339,1.);
#8223=VECTOR('',#31340,1.);
#8224=VECTOR('',#31343,1.);
#8225=VECTOR('',#31344,1.);
#8226=VECTOR('',#31347,1.);
#8227=VECTOR('',#31352,1.);
#8228=VECTOR('',#31353,1.);
#8229=VECTOR('',#31356,1.);
#8230=VECTOR('',#31357,1.);
#8231=VECTOR('',#31360,1.);
#8232=VECTOR('',#31365,1.);
#8233=VECTOR('',#31366,1.);
#8234=VECTOR('',#31369,1.);
#8235=VECTOR('',#31370,1.);
#8236=VECTOR('',#31373,1.);
#8237=VECTOR('',#31378,1.);
#8238=VECTOR('',#31379,1.);
#8239=VECTOR('',#31382,1.);
#8240=VECTOR('',#31383,1.);
#8241=VECTOR('',#31386,1.);
#8242=VECTOR('',#31391,1.);
#8243=VECTOR('',#31392,1.);
#8244=VECTOR('',#31395,1.);
#8245=VECTOR('',#31396,1.);
#8246=VECTOR('',#31399,1.);
#8247=VECTOR('',#31404,1.);
#8248=VECTOR('',#31405,1.);
#8249=VECTOR('',#31408,1.);
#8250=VECTOR('',#31409,1.);
#8251=VECTOR('',#31412,1.);
#8252=VECTOR('',#31417,1.);
#8253=VECTOR('',#31418,1.);
#8254=VECTOR('',#31421,1.);
#8255=VECTOR('',#31422,1.);
#8256=VECTOR('',#31425,1.);
#8257=VECTOR('',#31430,1.);
#8258=VECTOR('',#31431,1.);
#8259=VECTOR('',#31434,1.);
#8260=VECTOR('',#31435,1.);
#8261=VECTOR('',#31438,1.);
#8262=VECTOR('',#31443,1.);
#8263=VECTOR('',#31444,1.);
#8264=VECTOR('',#31447,1.);
#8265=VECTOR('',#31448,1.);
#8266=VECTOR('',#31451,1.);
#8267=VECTOR('',#31456,1.);
#8268=VECTOR('',#31457,1.);
#8269=VECTOR('',#31460,1.);
#8270=VECTOR('',#31461,1.);
#8271=VECTOR('',#31464,1.);
#8272=VECTOR('',#31469,1.);
#8273=VECTOR('',#31470,1.);
#8274=VECTOR('',#31473,1.);
#8275=VECTOR('',#31474,1.);
#8276=VECTOR('',#31477,1.);
#8277=VECTOR('',#31482,1.);
#8278=VECTOR('',#31483,1.);
#8279=VECTOR('',#31486,1.);
#8280=VECTOR('',#31487,1.);
#8281=VECTOR('',#31490,1.);
#8282=VECTOR('',#31495,1.);
#8283=VECTOR('',#31496,1.);
#8284=VECTOR('',#31499,1.);
#8285=VECTOR('',#31500,1.);
#8286=VECTOR('',#31503,1.);
#8287=VECTOR('',#31508,1.);
#8288=VECTOR('',#31509,1.);
#8289=VECTOR('',#31512,1.);
#8290=VECTOR('',#31513,1.);
#8291=VECTOR('',#31516,1.);
#8292=VECTOR('',#31521,1.);
#8293=VECTOR('',#31522,1.);
#8294=VECTOR('',#31525,1.);
#8295=VECTOR('',#31526,1.);
#8296=VECTOR('',#31529,1.);
#8297=VECTOR('',#31534,1.);
#8298=VECTOR('',#31535,1.);
#8299=VECTOR('',#31540,1.);
#8300=VECTOR('',#31541,1.);
#8301=VECTOR('',#31544,1.);
#8302=VECTOR('',#31549,1.);
#8303=VECTOR('',#31550,1.);
#8304=VECTOR('',#31553,1.);
#8305=VECTOR('',#31554,1.);
#8306=VECTOR('',#31557,1.);
#8307=VECTOR('',#31562,1.);
#8308=VECTOR('',#31563,1.);
#8309=VECTOR('',#31566,1.);
#8310=VECTOR('',#31567,1.);
#8311=VECTOR('',#31570,1.);
#8312=VECTOR('',#31575,1.);
#8313=VECTOR('',#31576,1.);
#8314=VECTOR('',#31579,1.);
#8315=VECTOR('',#31580,1.);
#8316=VECTOR('',#31583,1.);
#8317=VECTOR('',#31588,1.);
#8318=VECTOR('',#31589,1.);
#8319=VECTOR('',#31592,1.);
#8320=VECTOR('',#31593,1.);
#8321=VECTOR('',#31596,1.);
#8322=VECTOR('',#31601,1.);
#8323=VECTOR('',#31602,1.);
#8324=VECTOR('',#31605,1.);
#8325=VECTOR('',#31606,1.);
#8326=VECTOR('',#31609,1.);
#8327=VECTOR('',#31614,1.);
#8328=VECTOR('',#31615,1.);
#8329=VECTOR('',#31618,1.);
#8330=VECTOR('',#31619,1.);
#8331=VECTOR('',#31622,1.);
#8332=VECTOR('',#31627,1.);
#8333=VECTOR('',#31628,1.);
#8334=VECTOR('',#31631,1.);
#8335=VECTOR('',#31632,1.);
#8336=VECTOR('',#31635,1.);
#8337=VECTOR('',#31640,1.);
#8338=VECTOR('',#31641,1.);
#8339=VECTOR('',#31644,1.);
#8340=VECTOR('',#31645,1.);
#8341=VECTOR('',#31648,1.);
#8342=VECTOR('',#31653,1.);
#8343=VECTOR('',#31654,1.);
#8344=VECTOR('',#31657,1.);
#8345=VECTOR('',#31658,1.);
#8346=VECTOR('',#31661,1.);
#8347=VECTOR('',#31666,1.);
#8348=VECTOR('',#31667,1.);
#8349=VECTOR('',#31670,1.);
#8350=VECTOR('',#31671,1.);
#8351=VECTOR('',#31674,1.);
#8352=VECTOR('',#31679,1.);
#8353=VECTOR('',#31680,1.);
#8354=VECTOR('',#31683,1.);
#8355=VECTOR('',#31684,1.);
#8356=VECTOR('',#31687,1.);
#8357=VECTOR('',#31692,1.);
#8358=VECTOR('',#31693,1.);
#8359=VECTOR('',#31696,1.);
#8360=VECTOR('',#31697,1.);
#8361=VECTOR('',#31700,1.);
#8362=VECTOR('',#31705,1.);
#8363=VECTOR('',#31706,1.);
#8364=VECTOR('',#31709,1.);
#8365=VECTOR('',#31710,1.);
#8366=VECTOR('',#31713,1.);
#8367=VECTOR('',#31718,1.);
#8368=VECTOR('',#31719,1.);
#8369=VECTOR('',#31722,1.);
#8370=VECTOR('',#31723,1.);
#8371=VECTOR('',#31726,1.);
#8372=VECTOR('',#31731,1.);
#8373=VECTOR('',#31732,1.);
#8374=VECTOR('',#31735,1.);
#8375=VECTOR('',#31736,1.);
#8376=VECTOR('',#31739,1.);
#8377=VECTOR('',#31744,1.);
#8378=VECTOR('',#31745,1.);
#8379=VECTOR('',#31748,1.);
#8380=VECTOR('',#31749,1.);
#8381=VECTOR('',#31752,1.);
#8382=VECTOR('',#31757,1.);
#8383=VECTOR('',#31758,1.);
#8384=VECTOR('',#31761,1.);
#8385=VECTOR('',#31762,1.);
#8386=VECTOR('',#31765,1.);
#8387=VECTOR('',#31802,0.19);
#8388=VECTOR('',#31841,1.);
#8389=VECTOR('',#31844,1.);
#8390=VECTOR('',#31849,1.);
#8391=VECTOR('',#31850,1.);
#8392=VECTOR('',#31853,1.);
#8393=VECTOR('',#31860,0.1825);
#8394=VECTOR('',#31863,0.0346410161513776);
#8395=VECTOR('',#31868,1.);
#8396=VECTOR('',#31869,1.);
#8397=VECTOR('',#31870,1.);
#8398=VECTOR('',#31871,1.);
#8399=VECTOR('',#31874,1.);
#8400=VECTOR('',#31875,1.);
#8401=VECTOR('',#31876,1.);
#8402=VECTOR('',#31879,1.);
#8403=VECTOR('',#31880,1.);
#8404=VECTOR('',#31881,1.);
#8405=VECTOR('',#31884,1.);
#8406=VECTOR('',#31885,1.);
#8407=VECTOR('',#31886,1.);
#8408=VECTOR('',#31889,1.);
#8409=VECTOR('',#31890,1.);
#8410=VECTOR('',#31891,1.);
#8411=VECTOR('',#31894,1.);
#8412=VECTOR('',#31895,1.);
#8413=VECTOR('',#31904,0.088);
#8414=VECTOR('',#31913,0.105);
#9742=CIRCLE('',#26254,0.096675);
#9743=CIRCLE('',#26255,0.096675);
#9744=CIRCLE('',#26256,0.096675);
#9745=CIRCLE('',#26285,0.0739);
#9746=CIRCLE('',#26314,0.0739);
#9747=CIRCLE('',#26316,0.096675);
#9748=CIRCLE('',#26317,0.096675);
#9749=CIRCLE('',#26319,0.0739);
#9750=CIRCLE('',#26322,0.19);
#9751=CIRCLE('',#26326,0.19);
#9752=CIRCLE('',#26330,0.19);
#9753=CIRCLE('',#26334,0.19);
#9754=CIRCLE('',#26338,0.19);
#9755=CIRCLE('',#26342,0.19);
#9756=CIRCLE('',#26346,0.19);
#9757=CIRCLE('',#26350,0.19);
#9758=CIRCLE('',#26354,0.19);
#9759=CIRCLE('',#26358,0.19);
#9760=CIRCLE('',#26362,0.19);
#9761=CIRCLE('',#26366,0.19);
#9762=CIRCLE('',#26370,0.19);
#9763=CIRCLE('',#26374,0.19);
#9764=CIRCLE('',#26378,0.19);
#9765=CIRCLE('',#26382,0.19);
#9766=CIRCLE('',#26386,0.19);
#9767=CIRCLE('',#26390,0.19);
#9768=CIRCLE('',#26391,0.19);
#9769=CIRCLE('',#26395,0.19);
#9770=CIRCLE('',#26399,0.19);
#9771=CIRCLE('',#26403,0.19);
#9772=CIRCLE('',#26407,0.19);
#9773=CIRCLE('',#26411,0.19);
#9774=CIRCLE('',#26415,0.19);
#9775=CIRCLE('',#26419,0.19);
#9776=CIRCLE('',#26423,0.19);
#9777=CIRCLE('',#26427,0.19);
#9778=CIRCLE('',#26431,0.19);
#9779=CIRCLE('',#26435,0.19);
#9780=CIRCLE('',#26439,0.19);
#9781=CIRCLE('',#26443,0.19);
#9782=CIRCLE('',#26447,0.19);
#9783=CIRCLE('',#26451,0.19);
#9784=CIRCLE('',#26455,0.19);
#9785=CIRCLE('',#26459,0.19);
#9786=CIRCLE('',#26463,0.19);
#9787=CIRCLE('',#26464,0.19);
#9788=CIRCLE('',#26465,0.19);
#9789=CIRCLE('',#26466,0.19);
#9790=CIRCLE('',#26467,0.19);
#9791=CIRCLE('',#26468,0.19);
#9792=CIRCLE('',#26469,0.19);
#9793=CIRCLE('',#26470,0.19);
#9794=CIRCLE('',#26471,0.19);
#9795=CIRCLE('',#26472,0.19);
#9796=CIRCLE('',#26473,0.19);
#9797=CIRCLE('',#26474,0.19);
#9798=CIRCLE('',#26475,0.19);
#9799=CIRCLE('',#26476,0.19);
#9800=CIRCLE('',#26477,0.19);
#9801=CIRCLE('',#26478,0.19);
#9802=CIRCLE('',#26479,0.19);
#9803=CIRCLE('',#26480,0.19);
#9804=CIRCLE('',#26481,0.19);
#9805=CIRCLE('',#26482,0.19);
#9806=CIRCLE('',#26483,0.19);
#9807=CIRCLE('',#26484,0.19);
#9808=CIRCLE('',#26485,0.19);
#9809=CIRCLE('',#26486,0.19);
#9810=CIRCLE('',#26487,0.19);
#9811=CIRCLE('',#26488,0.19);
#9812=CIRCLE('',#26489,0.19);
#9813=CIRCLE('',#26490,0.19);
#9814=CIRCLE('',#26491,0.19);
#9815=CIRCLE('',#26492,0.19);
#9816=CIRCLE('',#26493,0.19);
#9817=CIRCLE('',#26494,0.19);
#9818=CIRCLE('',#26495,0.19);
#9819=CIRCLE('',#26496,0.19);
#9820=CIRCLE('',#26497,0.19);
#9821=CIRCLE('',#26498,0.19);
#9822=CIRCLE('',#26499,0.19);
#9823=CIRCLE('',#26500,0.19);
#9824=CIRCLE('',#26505,0.175);
#9825=CIRCLE('',#26507,0.0677181486487011);
#9826=CIRCLE('',#26516,0.076);
#9827=CIRCLE('',#26519,0.096675);
#9828=CIRCLE('',#26521,0.11);
#11185=VERTEX_POINT('',#39976);
#11186=VERTEX_POINT('',#39977);
#11187=VERTEX_POINT('',#39979);
#11188=VERTEX_POINT('',#39993);
#11189=VERTEX_POINT('',#39995);
#11190=VERTEX_POINT('',#39998);
#11191=VERTEX_POINT('',#40011);
#11192=VERTEX_POINT('',#40012);
#11193=VERTEX_POINT('',#40059);
#11194=VERTEX_POINT('',#40060);
#11195=VERTEX_POINT('',#40110);
#11196=VERTEX_POINT('',#40111);
#11197=VERTEX_POINT('',#40158);
#11198=VERTEX_POINT('',#40159);
#11199=VERTEX_POINT('',#40206);
#11200=VERTEX_POINT('',#40207);
#11201=VERTEX_POINT('',#40260);
#11202=VERTEX_POINT('',#40261);
#11203=VERTEX_POINT('',#40308);
#11204=VERTEX_POINT('',#40309);
#11205=VERTEX_POINT('',#40356);
#11206=VERTEX_POINT('',#40357);
#11207=VERTEX_POINT('',#40410);
#11208=VERTEX_POINT('',#40411);
#11209=VERTEX_POINT('',#40458);
#11210=VERTEX_POINT('',#40459);
#11211=VERTEX_POINT('',#40506);
#11212=VERTEX_POINT('',#40507);
#11213=VERTEX_POINT('',#40554);
#11214=VERTEX_POINT('',#40555);
#11215=VERTEX_POINT('',#40605);
#11216=VERTEX_POINT('',#40606);
#11217=VERTEX_POINT('',#40653);
#11218=VERTEX_POINT('',#40654);
#11219=VERTEX_POINT('',#40701);
#11220=VERTEX_POINT('',#40702);
#11221=VERTEX_POINT('',#40755);
#11222=VERTEX_POINT('',#40756);
#11223=VERTEX_POINT('',#40803);
#11224=VERTEX_POINT('',#40804);
#11225=VERTEX_POINT('',#40851);
#11226=VERTEX_POINT('',#40852);
#11227=VERTEX_POINT('',#40905);
#11228=VERTEX_POINT('',#40906);
#11229=VERTEX_POINT('',#40953);
#11230=VERTEX_POINT('',#40954);
#11231=VERTEX_POINT('',#41001);
#11232=VERTEX_POINT('',#41002);
#11233=VERTEX_POINT('',#41049);
#11234=VERTEX_POINT('',#41050);
#11235=VERTEX_POINT('',#41100);
#11236=VERTEX_POINT('',#41101);
#11237=VERTEX_POINT('',#41148);
#11238=VERTEX_POINT('',#41149);
#11239=VERTEX_POINT('',#41196);
#11240=VERTEX_POINT('',#41197);
#11241=VERTEX_POINT('',#41250);
#11242=VERTEX_POINT('',#41251);
#11243=VERTEX_POINT('',#41298);
#11244=VERTEX_POINT('',#41299);
#11245=VERTEX_POINT('',#41346);
#11246=VERTEX_POINT('',#41347);
#11247=VERTEX_POINT('',#41349);
#11248=VERTEX_POINT('',#41357);
#11249=VERTEX_POINT('',#41365);
#11250=VERTEX_POINT('',#41366);
#11251=VERTEX_POINT('',#41390);
#11252=VERTEX_POINT('',#41391);
#11253=VERTEX_POINT('',#41414);
#11254=VERTEX_POINT('',#41415);
#11255=VERTEX_POINT('',#41439);
#11256=VERTEX_POINT('',#41440);
#11257=VERTEX_POINT('',#41464);
#11258=VERTEX_POINT('',#41465);
#11259=VERTEX_POINT('',#41488);
#11260=VERTEX_POINT('',#41489);
#11261=VERTEX_POINT('',#41513);
#11262=VERTEX_POINT('',#41514);
#11263=VERTEX_POINT('',#41537);
#11264=VERTEX_POINT('',#41538);
#11265=VERTEX_POINT('',#41562);
#11266=VERTEX_POINT('',#41563);
#11267=VERTEX_POINT('',#41586);
#11268=VERTEX_POINT('',#41587);
#11269=VERTEX_POINT('',#41611);
#11270=VERTEX_POINT('',#41612);
#11271=VERTEX_POINT('',#41636);
#11272=VERTEX_POINT('',#41637);
#11273=VERTEX_POINT('',#41660);
#11274=VERTEX_POINT('',#41661);
#11275=VERTEX_POINT('',#41685);
#11276=VERTEX_POINT('',#41686);
#11277=VERTEX_POINT('',#41710);
#11278=VERTEX_POINT('',#41711);
#11279=VERTEX_POINT('',#41734);
#11280=VERTEX_POINT('',#41735);
#11281=VERTEX_POINT('',#41759);
#11282=VERTEX_POINT('',#41760);
#11283=VERTEX_POINT('',#41784);
#11284=VERTEX_POINT('',#41785);
#11285=VERTEX_POINT('',#41808);
#11286=VERTEX_POINT('',#41809);
#11287=VERTEX_POINT('',#41832);
#11288=VERTEX_POINT('',#41833);
#11289=VERTEX_POINT('',#41857);
#11290=VERTEX_POINT('',#41858);
#11291=VERTEX_POINT('',#41882);
#11292=VERTEX_POINT('',#41883);
#11293=VERTEX_POINT('',#41906);
#11294=VERTEX_POINT('',#41907);
#11295=VERTEX_POINT('',#41931);
#11296=VERTEX_POINT('',#41932);
#11297=VERTEX_POINT('',#41956);
#11298=VERTEX_POINT('',#41957);
#11299=VERTEX_POINT('',#41980);
#11300=VERTEX_POINT('',#41981);
#11301=VERTEX_POINT('',#42005);
#11302=VERTEX_POINT('',#42006);
#11303=VERTEX_POINT('',#42030);
#11304=VERTEX_POINT('',#42031);
#11305=VERTEX_POINT('',#42033);
#11306=VERTEX_POINT('',#42055);
#11307=VERTEX_POINT('',#42102);
#11308=VERTEX_POINT('',#42104);
#11309=VERTEX_POINT('',#42913);
#11310=VERTEX_POINT('',#43772);
#11311=VERTEX_POINT('',#43773);
#11312=VERTEX_POINT('',#43775);
#11313=VERTEX_POINT('',#43779);
#11314=VERTEX_POINT('',#43781);
#11315=VERTEX_POINT('',#43787);
#11316=VERTEX_POINT('',#43793);
#11317=VERTEX_POINT('',#43794);
#11318=VERTEX_POINT('',#43796);
#11319=VERTEX_POINT('',#43800);
#11320=VERTEX_POINT('',#43802);
#11321=VERTEX_POINT('',#43808);
#11322=VERTEX_POINT('',#43814);
#11323=VERTEX_POINT('',#43815);
#11324=VERTEX_POINT('',#43817);
#11325=VERTEX_POINT('',#43821);
#11326=VERTEX_POINT('',#43823);
#11327=VERTEX_POINT('',#43829);
#11328=VERTEX_POINT('',#43835);
#11329=VERTEX_POINT('',#43836);
#11330=VERTEX_POINT('',#43838);
#11331=VERTEX_POINT('',#43842);
#11332=VERTEX_POINT('',#43844);
#11333=VERTEX_POINT('',#43850);
#11334=VERTEX_POINT('',#43856);
#11335=VERTEX_POINT('',#43857);
#11336=VERTEX_POINT('',#43859);
#11337=VERTEX_POINT('',#43863);
#11338=VERTEX_POINT('',#43865);
#11339=VERTEX_POINT('',#43871);
#11340=VERTEX_POINT('',#43877);
#11341=VERTEX_POINT('',#43878);
#11342=VERTEX_POINT('',#43880);
#11343=VERTEX_POINT('',#43884);
#11344=VERTEX_POINT('',#43886);
#11345=VERTEX_POINT('',#43892);
#11346=VERTEX_POINT('',#43898);
#11347=VERTEX_POINT('',#43899);
#11348=VERTEX_POINT('',#43901);
#11349=VERTEX_POINT('',#43905);
#11350=VERTEX_POINT('',#43907);
#11351=VERTEX_POINT('',#43913);
#11352=VERTEX_POINT('',#43919);
#11353=VERTEX_POINT('',#43920);
#11354=VERTEX_POINT('',#43922);
#11355=VERTEX_POINT('',#43926);
#11356=VERTEX_POINT('',#43928);
#11357=VERTEX_POINT('',#43934);
#11358=VERTEX_POINT('',#43940);
#11359=VERTEX_POINT('',#43941);
#11360=VERTEX_POINT('',#43943);
#11361=VERTEX_POINT('',#43947);
#11362=VERTEX_POINT('',#43949);
#11363=VERTEX_POINT('',#43955);
#11364=VERTEX_POINT('',#43961);
#11365=VERTEX_POINT('',#43962);
#11366=VERTEX_POINT('',#43964);
#11367=VERTEX_POINT('',#43968);
#11368=VERTEX_POINT('',#43970);
#11369=VERTEX_POINT('',#43976);
#11370=VERTEX_POINT('',#43982);
#11371=VERTEX_POINT('',#43983);
#11372=VERTEX_POINT('',#43985);
#11373=VERTEX_POINT('',#43989);
#11374=VERTEX_POINT('',#43991);
#11375=VERTEX_POINT('',#43997);
#11376=VERTEX_POINT('',#44003);
#11377=VERTEX_POINT('',#44004);
#11378=VERTEX_POINT('',#44006);
#11379=VERTEX_POINT('',#44010);
#11380=VERTEX_POINT('',#44012);
#11381=VERTEX_POINT('',#44018);
#11382=VERTEX_POINT('',#44024);
#11383=VERTEX_POINT('',#44025);
#11384=VERTEX_POINT('',#44027);
#11385=VERTEX_POINT('',#44031);
#11386=VERTEX_POINT('',#44033);
#11387=VERTEX_POINT('',#44039);
#11388=VERTEX_POINT('',#44045);
#11389=VERTEX_POINT('',#44046);
#11390=VERTEX_POINT('',#44048);
#11391=VERTEX_POINT('',#44052);
#11392=VERTEX_POINT('',#44054);
#11393=VERTEX_POINT('',#44060);
#11394=VERTEX_POINT('',#44066);
#11395=VERTEX_POINT('',#44067);
#11396=VERTEX_POINT('',#44069);
#11397=VERTEX_POINT('',#44073);
#11398=VERTEX_POINT('',#44075);
#11399=VERTEX_POINT('',#44081);
#11400=VERTEX_POINT('',#44087);
#11401=VERTEX_POINT('',#44088);
#11402=VERTEX_POINT('',#44090);
#11403=VERTEX_POINT('',#44094);
#11404=VERTEX_POINT('',#44096);
#11405=VERTEX_POINT('',#44102);
#11406=VERTEX_POINT('',#44108);
#11407=VERTEX_POINT('',#44109);
#11408=VERTEX_POINT('',#44111);
#11409=VERTEX_POINT('',#44115);
#11410=VERTEX_POINT('',#44117);
#11411=VERTEX_POINT('',#44123);
#11412=VERTEX_POINT('',#44129);
#11413=VERTEX_POINT('',#44130);
#11414=VERTEX_POINT('',#44132);
#11415=VERTEX_POINT('',#44134);
#11416=VERTEX_POINT('',#44138);
#11417=VERTEX_POINT('',#44140);
#11418=VERTEX_POINT('',#44146);
#11419=VERTEX_POINT('',#44152);
#11420=VERTEX_POINT('',#44153);
#11421=VERTEX_POINT('',#44155);
#11422=VERTEX_POINT('',#44159);
#11423=VERTEX_POINT('',#44161);
#11424=VERTEX_POINT('',#44167);
#11425=VERTEX_POINT('',#44173);
#11426=VERTEX_POINT('',#44174);
#11427=VERTEX_POINT('',#44176);
#11428=VERTEX_POINT('',#44180);
#11429=VERTEX_POINT('',#44182);
#11430=VERTEX_POINT('',#44188);
#11431=VERTEX_POINT('',#44194);
#11432=VERTEX_POINT('',#44195);
#11433=VERTEX_POINT('',#44197);
#11434=VERTEX_POINT('',#44201);
#11435=VERTEX_POINT('',#44203);
#11436=VERTEX_POINT('',#44209);
#11437=VERTEX_POINT('',#44215);
#11438=VERTEX_POINT('',#44216);
#11439=VERTEX_POINT('',#44218);
#11440=VERTEX_POINT('',#44222);
#11441=VERTEX_POINT('',#44224);
#11442=VERTEX_POINT('',#44230);
#11443=VERTEX_POINT('',#44236);
#11444=VERTEX_POINT('',#44237);
#11445=VERTEX_POINT('',#44239);
#11446=VERTEX_POINT('',#44243);
#11447=VERTEX_POINT('',#44245);
#11448=VERTEX_POINT('',#44251);
#11449=VERTEX_POINT('',#44257);
#11450=VERTEX_POINT('',#44258);
#11451=VERTEX_POINT('',#44260);
#11452=VERTEX_POINT('',#44264);
#11453=VERTEX_POINT('',#44266);
#11454=VERTEX_POINT('',#44272);
#11455=VERTEX_POINT('',#44278);
#11456=VERTEX_POINT('',#44279);
#11457=VERTEX_POINT('',#44281);
#11458=VERTEX_POINT('',#44285);
#11459=VERTEX_POINT('',#44287);
#11460=VERTEX_POINT('',#44293);
#11461=VERTEX_POINT('',#44299);
#11462=VERTEX_POINT('',#44300);
#11463=VERTEX_POINT('',#44302);
#11464=VERTEX_POINT('',#44306);
#11465=VERTEX_POINT('',#44308);
#11466=VERTEX_POINT('',#44314);
#11467=VERTEX_POINT('',#44320);
#11468=VERTEX_POINT('',#44321);
#11469=VERTEX_POINT('',#44323);
#11470=VERTEX_POINT('',#44327);
#11471=VERTEX_POINT('',#44329);
#11472=VERTEX_POINT('',#44335);
#11473=VERTEX_POINT('',#44341);
#11474=VERTEX_POINT('',#44342);
#11475=VERTEX_POINT('',#44344);
#11476=VERTEX_POINT('',#44348);
#11477=VERTEX_POINT('',#44350);
#11478=VERTEX_POINT('',#44356);
#11479=VERTEX_POINT('',#44362);
#11480=VERTEX_POINT('',#44363);
#11481=VERTEX_POINT('',#44365);
#11482=VERTEX_POINT('',#44369);
#11483=VERTEX_POINT('',#44371);
#11484=VERTEX_POINT('',#44377);
#11485=VERTEX_POINT('',#44383);
#11486=VERTEX_POINT('',#44384);
#11487=VERTEX_POINT('',#44386);
#11488=VERTEX_POINT('',#44390);
#11489=VERTEX_POINT('',#44392);
#11490=VERTEX_POINT('',#44398);
#11491=VERTEX_POINT('',#44404);
#11492=VERTEX_POINT('',#44405);
#11493=VERTEX_POINT('',#44407);
#11494=VERTEX_POINT('',#44411);
#11495=VERTEX_POINT('',#44413);
#11496=VERTEX_POINT('',#44419);
#11497=VERTEX_POINT('',#44425);
#11498=VERTEX_POINT('',#44426);
#11499=VERTEX_POINT('',#44428);
#11500=VERTEX_POINT('',#44432);
#11501=VERTEX_POINT('',#44434);
#11502=VERTEX_POINT('',#44440);
#11503=VERTEX_POINT('',#44446);
#11504=VERTEX_POINT('',#44447);
#11505=VERTEX_POINT('',#44449);
#11506=VERTEX_POINT('',#44453);
#11507=VERTEX_POINT('',#44455);
#11508=VERTEX_POINT('',#44461);
#11509=VERTEX_POINT('',#44467);
#11510=VERTEX_POINT('',#44468);
#11511=VERTEX_POINT('',#44470);
#11512=VERTEX_POINT('',#44474);
#11513=VERTEX_POINT('',#44476);
#11514=VERTEX_POINT('',#44482);
#11515=VERTEX_POINT('',#44488);
#11516=VERTEX_POINT('',#44489);
#11517=VERTEX_POINT('',#44491);
#11518=VERTEX_POINT('',#44495);
#11519=VERTEX_POINT('',#44497);
#11520=VERTEX_POINT('',#44503);
#11521=VERTEX_POINT('',#44526);
#11522=VERTEX_POINT('',#44546);
#11523=VERTEX_POINT('',#44548);
#11524=VERTEX_POINT('',#44550);
#11525=VERTEX_POINT('',#44552);
#11526=VERTEX_POINT('',#44556);
#11527=VERTEX_POINT('',#44558);
#11528=VERTEX_POINT('',#44570);
#11529=VERTEX_POINT('',#44574);
#11530=VERTEX_POINT('',#44575);
#11531=VERTEX_POINT('',#44579);
#11532=VERTEX_POINT('',#44580);
#11533=VERTEX_POINT('',#44582);
#11534=VERTEX_POINT('',#44584);
#11535=VERTEX_POINT('',#44588);
#11536=VERTEX_POINT('',#44590);
#11537=VERTEX_POINT('',#44594);
#11538=VERTEX_POINT('',#44596);
#11539=VERTEX_POINT('',#44600);
#11540=VERTEX_POINT('',#44602);
#11541=VERTEX_POINT('',#44606);
#11542=VERTEX_POINT('',#44608);
#11543=VERTEX_POINT('',#44616);
#11544=VERTEX_POINT('',#44623);
#14132=EDGE_CURVE('',#11185,#11186,#6333,.T.);
#14133=EDGE_CURVE('',#11185,#11187,#568,.T.);
#14134=EDGE_CURVE('',#11187,#11188,#9742,.T.);
#14135=EDGE_CURVE('',#11188,#11189,#6334,.T.);
#14136=EDGE_CURVE('',#11189,#11189,#9743,.T.);
#14137=EDGE_CURVE('',#11188,#11190,#9744,.T.);
#14138=EDGE_CURVE('',#11190,#11186,#569,.T.);
#14139=EDGE_CURVE('',#11191,#11192,#6335,.T.);
#14140=EDGE_CURVE('',#11191,#11185,#570,.T.);
#14141=EDGE_CURVE('',#11186,#11192,#571,.T.);
#14142=EDGE_CURVE('',#11193,#11194,#6336,.T.);
#14143=EDGE_CURVE('',#11193,#11191,#572,.T.);
#14144=EDGE_CURVE('',#11192,#11194,#573,.T.);
#14145=EDGE_CURVE('',#11195,#11196,#6337,.T.);
#14146=EDGE_CURVE('',#11195,#11193,#574,.T.);
#14147=EDGE_CURVE('',#11194,#11196,#575,.T.);
#14148=EDGE_CURVE('',#11197,#11198,#6338,.T.);
#14149=EDGE_CURVE('',#11197,#11195,#576,.T.);
#14150=EDGE_CURVE('',#11196,#11198,#577,.T.);
#14151=EDGE_CURVE('',#11199,#11200,#6339,.T.);
#14152=EDGE_CURVE('',#11199,#11197,#578,.T.);
#14153=EDGE_CURVE('',#11198,#11200,#579,.T.);
#14154=EDGE_CURVE('',#11201,#11202,#6340,.T.);
#14155=EDGE_CURVE('',#11201,#11199,#580,.T.);
#14156=EDGE_CURVE('',#11200,#11202,#581,.T.);
#14157=EDGE_CURVE('',#11203,#11204,#6341,.T.);
#14158=EDGE_CURVE('',#11203,#11201,#582,.T.);
#14159=EDGE_CURVE('',#11202,#11204,#583,.T.);
#14160=EDGE_CURVE('',#11205,#11206,#6342,.T.);
#14161=EDGE_CURVE('',#11205,#11203,#584,.T.);
#14162=EDGE_CURVE('',#11204,#11206,#585,.T.);
#14163=EDGE_CURVE('',#11207,#11208,#6343,.T.);
#14164=EDGE_CURVE('',#11207,#11205,#586,.T.);
#14165=EDGE_CURVE('',#11206,#11208,#587,.T.);
#14166=EDGE_CURVE('',#11209,#11210,#6344,.T.);
#14167=EDGE_CURVE('',#11209,#11207,#588,.T.);
#14168=EDGE_CURVE('',#11208,#11210,#589,.T.);
#14169=EDGE_CURVE('',#11211,#11212,#6345,.T.);
#14170=EDGE_CURVE('',#11211,#11209,#590,.T.);
#14171=EDGE_CURVE('',#11210,#11212,#591,.T.);
#14172=EDGE_CURVE('',#11213,#11214,#6346,.T.);
#14173=EDGE_CURVE('',#11213,#11211,#592,.T.);
#14174=EDGE_CURVE('',#11212,#11214,#593,.T.);
#14175=EDGE_CURVE('',#11215,#11216,#6347,.T.);
#14176=EDGE_CURVE('',#11215,#11213,#594,.T.);
#14177=EDGE_CURVE('',#11214,#11216,#595,.T.);
#14178=EDGE_CURVE('',#11217,#11218,#6348,.T.);
#14179=EDGE_CURVE('',#11217,#11215,#596,.T.);
#14180=EDGE_CURVE('',#11216,#11218,#597,.T.);
#14181=EDGE_CURVE('',#11219,#11220,#6349,.T.);
#14182=EDGE_CURVE('',#11219,#11217,#598,.T.);
#14183=EDGE_CURVE('',#11218,#11220,#599,.T.);
#14184=EDGE_CURVE('',#11221,#11222,#6350,.T.);
#14185=EDGE_CURVE('',#11221,#11219,#600,.T.);
#14186=EDGE_CURVE('',#11220,#11222,#601,.T.);
#14187=EDGE_CURVE('',#11223,#11224,#6351,.T.);
#14188=EDGE_CURVE('',#11223,#11221,#602,.T.);
#14189=EDGE_CURVE('',#11222,#11224,#603,.T.);
#14190=EDGE_CURVE('',#11225,#11226,#6352,.T.);
#14191=EDGE_CURVE('',#11225,#11223,#604,.T.);
#14192=EDGE_CURVE('',#11224,#11226,#605,.T.);
#14193=EDGE_CURVE('',#11227,#11228,#6353,.T.);
#14194=EDGE_CURVE('',#11227,#11225,#606,.T.);
#14195=EDGE_CURVE('',#11226,#11228,#607,.T.);
#14196=EDGE_CURVE('',#11229,#11230,#6354,.T.);
#14197=EDGE_CURVE('',#11229,#11227,#608,.T.);
#14198=EDGE_CURVE('',#11228,#11230,#609,.T.);
#14199=EDGE_CURVE('',#11231,#11232,#6355,.T.);
#14200=EDGE_CURVE('',#11231,#11229,#610,.T.);
#14201=EDGE_CURVE('',#11230,#11232,#611,.T.);
#14202=EDGE_CURVE('',#11233,#11234,#6356,.T.);
#14203=EDGE_CURVE('',#11233,#11231,#612,.T.);
#14204=EDGE_CURVE('',#11232,#11234,#613,.T.);
#14205=EDGE_CURVE('',#11235,#11236,#6357,.T.);
#14206=EDGE_CURVE('',#11235,#11233,#614,.T.);
#14207=EDGE_CURVE('',#11234,#11236,#615,.T.);
#14208=EDGE_CURVE('',#11237,#11238,#6358,.T.);
#14209=EDGE_CURVE('',#11237,#11235,#616,.T.);
#14210=EDGE_CURVE('',#11236,#11238,#617,.T.);
#14211=EDGE_CURVE('',#11239,#11240,#6359,.T.);
#14212=EDGE_CURVE('',#11239,#11237,#618,.T.);
#14213=EDGE_CURVE('',#11238,#11240,#619,.T.);
#14214=EDGE_CURVE('',#11241,#11242,#6360,.T.);
#14215=EDGE_CURVE('',#11241,#11239,#620,.T.);
#14216=EDGE_CURVE('',#11240,#11242,#621,.T.);
#14217=EDGE_CURVE('',#11243,#11244,#6361,.T.);
#14218=EDGE_CURVE('',#11243,#11241,#622,.T.);
#14219=EDGE_CURVE('',#11242,#11244,#623,.T.);
#14220=EDGE_CURVE('',#11245,#11246,#6362,.T.);
#14221=EDGE_CURVE('',#11245,#11247,#624,.T.);
#14222=EDGE_CURVE('',#11248,#11247,#9745,.T.);
#14223=EDGE_CURVE('',#11246,#11248,#625,.T.);
#14224=EDGE_CURVE('',#11249,#11250,#6363,.T.);
#14225=EDGE_CURVE('',#11249,#11245,#626,.T.);
#14226=EDGE_CURVE('',#11250,#11246,#627,.T.);
#14227=EDGE_CURVE('',#11251,#11252,#6364,.T.);
#14228=EDGE_CURVE('',#11251,#11249,#628,.T.);
#14229=EDGE_CURVE('',#11252,#11250,#629,.T.);
#14230=EDGE_CURVE('',#11253,#11254,#6365,.T.);
#14231=EDGE_CURVE('',#11253,#11251,#630,.T.);
#14232=EDGE_CURVE('',#11254,#11252,#631,.T.);
#14233=EDGE_CURVE('',#11255,#11256,#6366,.T.);
#14234=EDGE_CURVE('',#11255,#11253,#632,.T.);
#14235=EDGE_CURVE('',#11256,#11254,#633,.T.);
#14236=EDGE_CURVE('',#11257,#11258,#6367,.T.);
#14237=EDGE_CURVE('',#11257,#11255,#634,.T.);
#14238=EDGE_CURVE('',#11258,#11256,#635,.T.);
#14239=EDGE_CURVE('',#11259,#11260,#6368,.T.);
#14240=EDGE_CURVE('',#11259,#11257,#636,.T.);
#14241=EDGE_CURVE('',#11260,#11258,#637,.T.);
#14242=EDGE_CURVE('',#11261,#11262,#6369,.T.);
#14243=EDGE_CURVE('',#11261,#11259,#638,.T.);
#14244=EDGE_CURVE('',#11262,#11260,#639,.T.);
#14245=EDGE_CURVE('',#11263,#11264,#6370,.T.);
#14246=EDGE_CURVE('',#11263,#11261,#640,.T.);
#14247=EDGE_CURVE('',#11264,#11262,#641,.T.);
#14248=EDGE_CURVE('',#11265,#11266,#6371,.T.);
#14249=EDGE_CURVE('',#11265,#11263,#642,.T.);
#14250=EDGE_CURVE('',#11266,#11264,#643,.T.);
#14251=EDGE_CURVE('',#11267,#11268,#6372,.T.);
#14252=EDGE_CURVE('',#11267,#11265,#644,.T.);
#14253=EDGE_CURVE('',#11268,#11266,#645,.T.);
#14254=EDGE_CURVE('',#11269,#11270,#6373,.T.);
#14255=EDGE_CURVE('',#11269,#11267,#646,.T.);
#14256=EDGE_CURVE('',#11270,#11268,#647,.T.);
#14257=EDGE_CURVE('',#11271,#11272,#6374,.T.);
#14258=EDGE_CURVE('',#11271,#11269,#648,.T.);
#14259=EDGE_CURVE('',#11272,#11270,#649,.T.);
#14260=EDGE_CURVE('',#11273,#11274,#6375,.T.);
#14261=EDGE_CURVE('',#11273,#11271,#650,.T.);
#14262=EDGE_CURVE('',#11274,#11272,#651,.T.);
#14263=EDGE_CURVE('',#11275,#11276,#6376,.T.);
#14264=EDGE_CURVE('',#11275,#11273,#652,.T.);
#14265=EDGE_CURVE('',#11276,#11274,#653,.T.);
#14266=EDGE_CURVE('',#11277,#11278,#6377,.T.);
#14267=EDGE_CURVE('',#11277,#11275,#654,.T.);
#14268=EDGE_CURVE('',#11278,#11276,#655,.T.);
#14269=EDGE_CURVE('',#11279,#11280,#6378,.T.);
#14270=EDGE_CURVE('',#11279,#11277,#656,.T.);
#14271=EDGE_CURVE('',#11280,#11278,#657,.T.);
#14272=EDGE_CURVE('',#11281,#11282,#6379,.T.);
#14273=EDGE_CURVE('',#11281,#11279,#658,.T.);
#14274=EDGE_CURVE('',#11282,#11280,#659,.T.);
#14275=EDGE_CURVE('',#11283,#11284,#6380,.T.);
#14276=EDGE_CURVE('',#11283,#11281,#660,.T.);
#14277=EDGE_CURVE('',#11284,#11282,#661,.T.);
#14278=EDGE_CURVE('',#11285,#11286,#6381,.T.);
#14279=EDGE_CURVE('',#11285,#11283,#662,.T.);
#14280=EDGE_CURVE('',#11286,#11284,#663,.T.);
#14281=EDGE_CURVE('',#11287,#11288,#6382,.T.);
#14282=EDGE_CURVE('',#11287,#11285,#664,.T.);
#14283=EDGE_CURVE('',#11288,#11286,#665,.T.);
#14284=EDGE_CURVE('',#11289,#11290,#6383,.T.);
#14285=EDGE_CURVE('',#11289,#11287,#666,.T.);
#14286=EDGE_CURVE('',#11290,#11288,#667,.T.);
#14287=EDGE_CURVE('',#11291,#11292,#6384,.T.);
#14288=EDGE_CURVE('',#11291,#11289,#668,.T.);
#14289=EDGE_CURVE('',#11292,#11290,#669,.T.);
#14290=EDGE_CURVE('',#11293,#11294,#6385,.T.);
#14291=EDGE_CURVE('',#11293,#11291,#670,.T.);
#14292=EDGE_CURVE('',#11294,#11292,#671,.T.);
#14293=EDGE_CURVE('',#11295,#11296,#6386,.T.);
#14294=EDGE_CURVE('',#11295,#11293,#672,.T.);
#14295=EDGE_CURVE('',#11296,#11294,#673,.T.);
#14296=EDGE_CURVE('',#11297,#11298,#6387,.T.);
#14297=EDGE_CURVE('',#11297,#11295,#674,.T.);
#14298=EDGE_CURVE('',#11298,#11296,#675,.T.);
#14299=EDGE_CURVE('',#11299,#11300,#6388,.T.);
#14300=EDGE_CURVE('',#11299,#11297,#676,.T.);
#14301=EDGE_CURVE('',#11300,#11298,#677,.T.);
#14302=EDGE_CURVE('',#11301,#11302,#6389,.T.);
#14303=EDGE_CURVE('',#11301,#11299,#678,.T.);
#14304=EDGE_CURVE('',#11302,#11300,#679,.T.);
#14305=EDGE_CURVE('',#11303,#11304,#6390,.T.);
#14306=EDGE_CURVE('',#11305,#11303,#9746,.T.);
#14307=EDGE_CURVE('',#11305,#11301,#680,.T.);
#14308=EDGE_CURVE('',#11304,#11302,#681,.T.);
#14309=EDGE_CURVE('',#11247,#11306,#682,.T.);
#14310=EDGE_CURVE('',#11307,#11306,#9747,.T.);
#14311=EDGE_CURVE('',#11308,#11307,#9748,.T.);
#14312=EDGE_CURVE('',#11308,#11248,#683,.T.);
#14313=EDGE_CURVE('',#11244,#11308,#684,.T.);
#14314=EDGE_CURVE('',#11309,#11190,#685,.T.);
#14315=EDGE_CURVE('',#11309,#11304,#686,.T.);
#14316=EDGE_CURVE('',#11187,#11305,#687,.T.);
#14317=EDGE_CURVE('',#11303,#11309,#9749,.T.);
#14318=EDGE_CURVE('',#11306,#11243,#688,.T.);
#14319=EDGE_CURVE('',#11310,#11311,#9750,.T.);
#14320=EDGE_CURVE('',#11310,#11312,#6391,.T.);
#14321=EDGE_CURVE('',#11312,#11311,#6392,.T.);
#14322=EDGE_CURVE('',#11311,#11313,#6393,.T.);
#14323=EDGE_CURVE('',#11312,#11314,#6394,.T.);
#14324=EDGE_CURVE('',#11313,#11314,#251,.T.);
#14325=EDGE_CURVE('',#11315,#11310,#6395,.T.);
#14326=EDGE_CURVE('',#11314,#11315,#252,.T.);
#14327=EDGE_CURVE('',#11316,#11317,#9751,.T.);
#14328=EDGE_CURVE('',#11316,#11318,#6396,.T.);
#14329=EDGE_CURVE('',#11318,#11317,#6397,.T.);
#14330=EDGE_CURVE('',#11317,#11319,#6398,.T.);
#14331=EDGE_CURVE('',#11318,#11320,#6399,.T.);
#14332=EDGE_CURVE('',#11319,#11320,#253,.T.);
#14333=EDGE_CURVE('',#11321,#11316,#6400,.T.);
#14334=EDGE_CURVE('',#11320,#11321,#254,.T.);
#14335=EDGE_CURVE('',#11322,#11323,#9752,.T.);
#14336=EDGE_CURVE('',#11322,#11324,#6401,.T.);
#14337=EDGE_CURVE('',#11324,#11323,#6402,.T.);
#14338=EDGE_CURVE('',#11323,#11325,#6403,.T.);
#14339=EDGE_CURVE('',#11324,#11326,#6404,.T.);
#14340=EDGE_CURVE('',#11325,#11326,#255,.T.);
#14341=EDGE_CURVE('',#11327,#11322,#6405,.T.);
#14342=EDGE_CURVE('',#11326,#11327,#256,.T.);
#14343=EDGE_CURVE('',#11328,#11329,#9753,.T.);
#14344=EDGE_CURVE('',#11328,#11330,#6406,.T.);
#14345=EDGE_CURVE('',#11330,#11329,#6407,.T.);
#14346=EDGE_CURVE('',#11329,#11331,#6408,.T.);
#14347=EDGE_CURVE('',#11330,#11332,#6409,.T.);
#14348=EDGE_CURVE('',#11331,#11332,#257,.T.);
#14349=EDGE_CURVE('',#11333,#11328,#6410,.T.);
#14350=EDGE_CURVE('',#11332,#11333,#258,.T.);
#14351=EDGE_CURVE('',#11334,#11335,#9754,.T.);
#14352=EDGE_CURVE('',#11334,#11336,#6411,.T.);
#14353=EDGE_CURVE('',#11336,#11335,#6412,.T.);
#14354=EDGE_CURVE('',#11335,#11337,#6413,.T.);
#14355=EDGE_CURVE('',#11336,#11338,#6414,.T.);
#14356=EDGE_CURVE('',#11337,#11338,#259,.T.);
#14357=EDGE_CURVE('',#11339,#11334,#6415,.T.);
#14358=EDGE_CURVE('',#11338,#11339,#260,.T.);
#14359=EDGE_CURVE('',#11340,#11341,#9755,.T.);
#14360=EDGE_CURVE('',#11340,#11342,#6416,.T.);
#14361=EDGE_CURVE('',#11342,#11341,#6417,.T.);
#14362=EDGE_CURVE('',#11341,#11343,#6418,.T.);
#14363=EDGE_CURVE('',#11342,#11344,#6419,.T.);
#14364=EDGE_CURVE('',#11343,#11344,#261,.T.);
#14365=EDGE_CURVE('',#11345,#11340,#6420,.T.);
#14366=EDGE_CURVE('',#11344,#11345,#262,.T.);
#14367=EDGE_CURVE('',#11346,#11347,#9756,.T.);
#14368=EDGE_CURVE('',#11346,#11348,#6421,.T.);
#14369=EDGE_CURVE('',#11348,#11347,#6422,.T.);
#14370=EDGE_CURVE('',#11347,#11349,#6423,.T.);
#14371=EDGE_CURVE('',#11348,#11350,#6424,.T.);
#14372=EDGE_CURVE('',#11349,#11350,#263,.T.);
#14373=EDGE_CURVE('',#11351,#11346,#6425,.T.);
#14374=EDGE_CURVE('',#11350,#11351,#264,.T.);
#14375=EDGE_CURVE('',#11352,#11353,#9757,.T.);
#14376=EDGE_CURVE('',#11352,#11354,#6426,.T.);
#14377=EDGE_CURVE('',#11354,#11353,#6427,.T.);
#14378=EDGE_CURVE('',#11353,#11355,#6428,.T.);
#14379=EDGE_CURVE('',#11354,#11356,#6429,.T.);
#14380=EDGE_CURVE('',#11355,#11356,#265,.T.);
#14381=EDGE_CURVE('',#11357,#11352,#6430,.T.);
#14382=EDGE_CURVE('',#11356,#11357,#266,.T.);
#14383=EDGE_CURVE('',#11358,#11359,#9758,.T.);
#14384=EDGE_CURVE('',#11358,#11360,#6431,.T.);
#14385=EDGE_CURVE('',#11360,#11359,#6432,.T.);
#14386=EDGE_CURVE('',#11359,#11361,#6433,.T.);
#14387=EDGE_CURVE('',#11360,#11362,#6434,.T.);
#14388=EDGE_CURVE('',#11361,#11362,#267,.T.);
#14389=EDGE_CURVE('',#11363,#11358,#6435,.T.);
#14390=EDGE_CURVE('',#11362,#11363,#268,.T.);
#14391=EDGE_CURVE('',#11364,#11365,#9759,.T.);
#14392=EDGE_CURVE('',#11364,#11366,#6436,.T.);
#14393=EDGE_CURVE('',#11366,#11365,#6437,.T.);
#14394=EDGE_CURVE('',#11365,#11367,#6438,.T.);
#14395=EDGE_CURVE('',#11366,#11368,#6439,.T.);
#14396=EDGE_CURVE('',#11367,#11368,#269,.T.);
#14397=EDGE_CURVE('',#11369,#11364,#6440,.T.);
#14398=EDGE_CURVE('',#11368,#11369,#270,.T.);
#14399=EDGE_CURVE('',#11370,#11371,#9760,.T.);
#14400=EDGE_CURVE('',#11370,#11372,#6441,.T.);
#14401=EDGE_CURVE('',#11372,#11371,#6442,.T.);
#14402=EDGE_CURVE('',#11371,#11373,#6443,.T.);
#14403=EDGE_CURVE('',#11372,#11374,#6444,.T.);
#14404=EDGE_CURVE('',#11373,#11374,#271,.T.);
#14405=EDGE_CURVE('',#11375,#11370,#6445,.T.);
#14406=EDGE_CURVE('',#11374,#11375,#272,.T.);
#14407=EDGE_CURVE('',#11376,#11377,#9761,.T.);
#14408=EDGE_CURVE('',#11376,#11378,#6446,.T.);
#14409=EDGE_CURVE('',#11378,#11377,#6447,.T.);
#14410=EDGE_CURVE('',#11377,#11379,#6448,.T.);
#14411=EDGE_CURVE('',#11378,#11380,#6449,.T.);
#14412=EDGE_CURVE('',#11379,#11380,#273,.T.);
#14413=EDGE_CURVE('',#11381,#11376,#6450,.T.);
#14414=EDGE_CURVE('',#11380,#11381,#274,.T.);
#14415=EDGE_CURVE('',#11382,#11383,#9762,.T.);
#14416=EDGE_CURVE('',#11382,#11384,#6451,.T.);
#14417=EDGE_CURVE('',#11384,#11383,#6452,.T.);
#14418=EDGE_CURVE('',#11383,#11385,#6453,.T.);
#14419=EDGE_CURVE('',#11384,#11386,#6454,.T.);
#14420=EDGE_CURVE('',#11385,#11386,#275,.T.);
#14421=EDGE_CURVE('',#11387,#11382,#6455,.T.);
#14422=EDGE_CURVE('',#11386,#11387,#276,.T.);
#14423=EDGE_CURVE('',#11388,#11389,#9763,.T.);
#14424=EDGE_CURVE('',#11388,#11390,#6456,.T.);
#14425=EDGE_CURVE('',#11390,#11389,#6457,.T.);
#14426=EDGE_CURVE('',#11389,#11391,#6458,.T.);
#14427=EDGE_CURVE('',#11390,#11392,#6459,.T.);
#14428=EDGE_CURVE('',#11391,#11392,#277,.T.);
#14429=EDGE_CURVE('',#11393,#11388,#6460,.T.);
#14430=EDGE_CURVE('',#11392,#11393,#278,.T.);
#14431=EDGE_CURVE('',#11394,#11395,#9764,.T.);
#14432=EDGE_CURVE('',#11394,#11396,#6461,.T.);
#14433=EDGE_CURVE('',#11396,#11395,#6462,.T.);
#14434=EDGE_CURVE('',#11395,#11397,#6463,.T.);
#14435=EDGE_CURVE('',#11396,#11398,#6464,.T.);
#14436=EDGE_CURVE('',#11397,#11398,#279,.T.);
#14437=EDGE_CURVE('',#11399,#11394,#6465,.T.);
#14438=EDGE_CURVE('',#11398,#11399,#280,.T.);
#14439=EDGE_CURVE('',#11400,#11401,#9765,.T.);
#14440=EDGE_CURVE('',#11400,#11402,#6466,.T.);
#14441=EDGE_CURVE('',#11402,#11401,#6467,.T.);
#14442=EDGE_CURVE('',#11401,#11403,#6468,.T.);
#14443=EDGE_CURVE('',#11402,#11404,#6469,.T.);
#14444=EDGE_CURVE('',#11403,#11404,#281,.T.);
#14445=EDGE_CURVE('',#11405,#11400,#6470,.T.);
#14446=EDGE_CURVE('',#11404,#11405,#282,.T.);
#14447=EDGE_CURVE('',#11406,#11407,#9766,.T.);
#14448=EDGE_CURVE('',#11406,#11408,#6471,.T.);
#14449=EDGE_CURVE('',#11408,#11407,#6472,.T.);
#14450=EDGE_CURVE('',#11407,#11409,#6473,.T.);
#14451=EDGE_CURVE('',#11408,#11410,#6474,.T.);
#14452=EDGE_CURVE('',#11409,#11410,#283,.T.);
#14453=EDGE_CURVE('',#11411,#11406,#6475,.T.);
#14454=EDGE_CURVE('',#11410,#11411,#284,.T.);
#14455=EDGE_CURVE('',#11412,#11413,#9767,.T.);
#14456=EDGE_CURVE('',#11412,#11414,#6476,.T.);
#14457=EDGE_CURVE('',#11414,#11415,#6477,.T.);
#14458=EDGE_CURVE('',#11413,#11415,#9768,.T.);
#14459=EDGE_CURVE('',#11415,#11416,#6478,.T.);
#14460=EDGE_CURVE('',#11414,#11417,#6479,.T.);
#14461=EDGE_CURVE('',#11416,#11417,#285,.T.);
#14462=EDGE_CURVE('',#11418,#11412,#6480,.T.);
#14463=EDGE_CURVE('',#11417,#11418,#286,.T.);
#14464=EDGE_CURVE('',#11419,#11420,#9769,.T.);
#14465=EDGE_CURVE('',#11419,#11421,#6481,.T.);
#14466=EDGE_CURVE('',#11421,#11420,#6482,.T.);
#14467=EDGE_CURVE('',#11420,#11422,#6483,.T.);
#14468=EDGE_CURVE('',#11421,#11423,#6484,.T.);
#14469=EDGE_CURVE('',#11422,#11423,#287,.T.);
#14470=EDGE_CURVE('',#11424,#11419,#6485,.T.);
#14471=EDGE_CURVE('',#11423,#11424,#288,.T.);
#14472=EDGE_CURVE('',#11425,#11426,#9770,.T.);
#14473=EDGE_CURVE('',#11425,#11427,#6486,.T.);
#14474=EDGE_CURVE('',#11427,#11426,#6487,.T.);
#14475=EDGE_CURVE('',#11426,#11428,#6488,.T.);
#14476=EDGE_CURVE('',#11427,#11429,#6489,.T.);
#14477=EDGE_CURVE('',#11428,#11429,#289,.T.);
#14478=EDGE_CURVE('',#11430,#11425,#6490,.T.);
#14479=EDGE_CURVE('',#11429,#11430,#290,.T.);
#14480=EDGE_CURVE('',#11431,#11432,#9771,.T.);
#14481=EDGE_CURVE('',#11431,#11433,#6491,.T.);
#14482=EDGE_CURVE('',#11433,#11432,#6492,.T.);
#14483=EDGE_CURVE('',#11432,#11434,#6493,.T.);
#14484=EDGE_CURVE('',#11433,#11435,#6494,.T.);
#14485=EDGE_CURVE('',#11434,#11435,#291,.T.);
#14486=EDGE_CURVE('',#11436,#11431,#6495,.T.);
#14487=EDGE_CURVE('',#11435,#11436,#292,.T.);
#14488=EDGE_CURVE('',#11437,#11438,#9772,.T.);
#14489=EDGE_CURVE('',#11437,#11439,#6496,.T.);
#14490=EDGE_CURVE('',#11439,#11438,#6497,.T.);
#14491=EDGE_CURVE('',#11438,#11440,#6498,.T.);
#14492=EDGE_CURVE('',#11439,#11441,#6499,.T.);
#14493=EDGE_CURVE('',#11440,#11441,#293,.T.);
#14494=EDGE_CURVE('',#11442,#11437,#6500,.T.);
#14495=EDGE_CURVE('',#11441,#11442,#294,.T.);
#14496=EDGE_CURVE('',#11443,#11444,#9773,.T.);
#14497=EDGE_CURVE('',#11443,#11445,#6501,.T.);
#14498=EDGE_CURVE('',#11445,#11444,#6502,.T.);
#14499=EDGE_CURVE('',#11444,#11446,#6503,.T.);
#14500=EDGE_CURVE('',#11445,#11447,#6504,.T.);
#14501=EDGE_CURVE('',#11446,#11447,#295,.T.);
#14502=EDGE_CURVE('',#11448,#11443,#6505,.T.);
#14503=EDGE_CURVE('',#11447,#11448,#296,.T.);
#14504=EDGE_CURVE('',#11449,#11450,#9774,.T.);
#14505=EDGE_CURVE('',#11449,#11451,#6506,.T.);
#14506=EDGE_CURVE('',#11451,#11450,#6507,.T.);
#14507=EDGE_CURVE('',#11450,#11452,#6508,.T.);
#14508=EDGE_CURVE('',#11451,#11453,#6509,.T.);
#14509=EDGE_CURVE('',#11452,#11453,#297,.T.);
#14510=EDGE_CURVE('',#11454,#11449,#6510,.T.);
#14511=EDGE_CURVE('',#11453,#11454,#298,.T.);
#14512=EDGE_CURVE('',#11455,#11456,#9775,.T.);
#14513=EDGE_CURVE('',#11455,#11457,#6511,.T.);
#14514=EDGE_CURVE('',#11457,#11456,#6512,.T.);
#14515=EDGE_CURVE('',#11456,#11458,#6513,.T.);
#14516=EDGE_CURVE('',#11457,#11459,#6514,.T.);
#14517=EDGE_CURVE('',#11458,#11459,#299,.T.);
#14518=EDGE_CURVE('',#11460,#11455,#6515,.T.);
#14519=EDGE_CURVE('',#11459,#11460,#300,.T.);
#14520=EDGE_CURVE('',#11461,#11462,#9776,.T.);
#14521=EDGE_CURVE('',#11461,#11463,#6516,.T.);
#14522=EDGE_CURVE('',#11463,#11462,#6517,.T.);
#14523=EDGE_CURVE('',#11462,#11464,#6518,.T.);
#14524=EDGE_CURVE('',#11463,#11465,#6519,.T.);
#14525=EDGE_CURVE('',#11464,#11465,#301,.T.);
#14526=EDGE_CURVE('',#11466,#11461,#6520,.T.);
#14527=EDGE_CURVE('',#11465,#11466,#302,.T.);
#14528=EDGE_CURVE('',#11467,#11468,#9777,.T.);
#14529=EDGE_CURVE('',#11467,#11469,#6521,.T.);
#14530=EDGE_CURVE('',#11469,#11468,#6522,.T.);
#14531=EDGE_CURVE('',#11468,#11470,#6523,.T.);
#14532=EDGE_CURVE('',#11469,#11471,#6524,.T.);
#14533=EDGE_CURVE('',#11470,#11471,#303,.T.);
#14534=EDGE_CURVE('',#11472,#11467,#6525,.T.);
#14535=EDGE_CURVE('',#11471,#11472,#304,.T.);
#14536=EDGE_CURVE('',#11473,#11474,#9778,.T.);
#14537=EDGE_CURVE('',#11473,#11475,#6526,.T.);
#14538=EDGE_CURVE('',#11475,#11474,#6527,.T.);
#14539=EDGE_CURVE('',#11474,#11476,#6528,.T.);
#14540=EDGE_CURVE('',#11475,#11477,#6529,.T.);
#14541=EDGE_CURVE('',#11476,#11477,#305,.T.);
#14542=EDGE_CURVE('',#11478,#11473,#6530,.T.);
#14543=EDGE_CURVE('',#11477,#11478,#306,.T.);
#14544=EDGE_CURVE('',#11479,#11480,#9779,.T.);
#14545=EDGE_CURVE('',#11479,#11481,#6531,.T.);
#14546=EDGE_CURVE('',#11481,#11480,#6532,.T.);
#14547=EDGE_CURVE('',#11480,#11482,#6533,.T.);
#14548=EDGE_CURVE('',#11481,#11483,#6534,.T.);
#14549=EDGE_CURVE('',#11482,#11483,#307,.T.);
#14550=EDGE_CURVE('',#11484,#11479,#6535,.T.);
#14551=EDGE_CURVE('',#11483,#11484,#308,.T.);
#14552=EDGE_CURVE('',#11485,#11486,#9780,.T.);
#14553=EDGE_CURVE('',#11485,#11487,#6536,.T.);
#14554=EDGE_CURVE('',#11487,#11486,#6537,.T.);
#14555=EDGE_CURVE('',#11486,#11488,#6538,.T.);
#14556=EDGE_CURVE('',#11487,#11489,#6539,.T.);
#14557=EDGE_CURVE('',#11488,#11489,#309,.T.);
#14558=EDGE_CURVE('',#11490,#11485,#6540,.T.);
#14559=EDGE_CURVE('',#11489,#11490,#310,.T.);
#14560=EDGE_CURVE('',#11491,#11492,#9781,.T.);
#14561=EDGE_CURVE('',#11491,#11493,#6541,.T.);
#14562=EDGE_CURVE('',#11493,#11492,#6542,.T.);
#14563=EDGE_CURVE('',#11492,#11494,#6543,.T.);
#14564=EDGE_CURVE('',#11493,#11495,#6544,.T.);
#14565=EDGE_CURVE('',#11494,#11495,#311,.T.);
#14566=EDGE_CURVE('',#11496,#11491,#6545,.T.);
#14567=EDGE_CURVE('',#11495,#11496,#312,.T.);
#14568=EDGE_CURVE('',#11497,#11498,#9782,.T.);
#14569=EDGE_CURVE('',#11497,#11499,#6546,.T.);
#14570=EDGE_CURVE('',#11499,#11498,#6547,.T.);
#14571=EDGE_CURVE('',#11498,#11500,#6548,.T.);
#14572=EDGE_CURVE('',#11499,#11501,#6549,.T.);
#14573=EDGE_CURVE('',#11500,#11501,#313,.T.);
#14574=EDGE_CURVE('',#11502,#11497,#6550,.T.);
#14575=EDGE_CURVE('',#11501,#11502,#314,.T.);
#14576=EDGE_CURVE('',#11503,#11504,#9783,.T.);
#14577=EDGE_CURVE('',#11503,#11505,#6551,.T.);
#14578=EDGE_CURVE('',#11505,#11504,#6552,.T.);
#14579=EDGE_CURVE('',#11504,#11506,#6553,.T.);
#14580=EDGE_CURVE('',#11505,#11507,#6554,.T.);
#14581=EDGE_CURVE('',#11506,#11507,#315,.T.);
#14582=EDGE_CURVE('',#11508,#11503,#6555,.T.);
#14583=EDGE_CURVE('',#11507,#11508,#316,.T.);
#14584=EDGE_CURVE('',#11509,#11510,#9784,.T.);
#14585=EDGE_CURVE('',#11509,#11511,#6556,.T.);
#14586=EDGE_CURVE('',#11511,#11510,#6557,.T.);
#14587=EDGE_CURVE('',#11510,#11512,#6558,.T.);
#14588=EDGE_CURVE('',#11511,#11513,#6559,.T.);
#14589=EDGE_CURVE('',#11512,#11513,#317,.T.);
#14590=EDGE_CURVE('',#11514,#11509,#6560,.T.);
#14591=EDGE_CURVE('',#11513,#11514,#318,.T.);
#14592=EDGE_CURVE('',#11515,#11516,#9785,.T.);
#14593=EDGE_CURVE('',#11515,#11517,#6561,.T.);
#14594=EDGE_CURVE('',#11517,#11516,#6562,.T.);
#14595=EDGE_CURVE('',#11516,#11518,#6563,.T.);
#14596=EDGE_CURVE('',#11517,#11519,#6564,.T.);
#14597=EDGE_CURVE('',#11518,#11519,#319,.T.);
#14598=EDGE_CURVE('',#11520,#11515,#6565,.T.);
#14599=EDGE_CURVE('',#11519,#11520,#320,.T.);
#14600=EDGE_CURVE('',#11321,#11313,#9786,.T.);
#14601=EDGE_CURVE('',#11327,#11319,#9787,.T.);
#14602=EDGE_CURVE('',#11333,#11325,#9788,.T.);
#14603=EDGE_CURVE('',#11339,#11331,#9789,.T.);
#14604=EDGE_CURVE('',#11345,#11337,#9790,.T.);
#14605=EDGE_CURVE('',#11351,#11343,#9791,.T.);
#14606=EDGE_CURVE('',#11357,#11349,#9792,.T.);
#14607=EDGE_CURVE('',#11363,#11355,#9793,.T.);
#14608=EDGE_CURVE('',#11369,#11361,#9794,.T.);
#14609=EDGE_CURVE('',#11375,#11367,#9795,.T.);
#14610=EDGE_CURVE('',#11381,#11373,#9796,.T.);
#14611=EDGE_CURVE('',#11387,#11379,#9797,.T.);
#14612=EDGE_CURVE('',#11393,#11385,#9798,.T.);
#14613=EDGE_CURVE('',#11399,#11391,#9799,.T.);
#14614=EDGE_CURVE('',#11405,#11397,#9800,.T.);
#14615=EDGE_CURVE('',#11411,#11403,#9801,.T.);
#14616=EDGE_CURVE('',#11418,#11409,#9802,.T.);
#14617=EDGE_CURVE('',#11413,#11521,#6566,.T.);
#14618=EDGE_CURVE('',#11521,#11521,#9803,.T.);
#14619=EDGE_CURVE('',#11424,#11416,#9804,.T.);
#14620=EDGE_CURVE('',#11430,#11422,#9805,.T.);
#14621=EDGE_CURVE('',#11436,#11428,#9806,.T.);
#14622=EDGE_CURVE('',#11442,#11434,#9807,.T.);
#14623=EDGE_CURVE('',#11448,#11440,#9808,.T.);
#14624=EDGE_CURVE('',#11454,#11446,#9809,.T.);
#14625=EDGE_CURVE('',#11460,#11452,#9810,.T.);
#14626=EDGE_CURVE('',#11466,#11458,#9811,.T.);
#14627=EDGE_CURVE('',#11472,#11464,#9812,.T.);
#14628=EDGE_CURVE('',#11478,#11470,#9813,.T.);
#14629=EDGE_CURVE('',#11484,#11476,#9814,.T.);
#14630=EDGE_CURVE('',#11490,#11482,#9815,.T.);
#14631=EDGE_CURVE('',#11496,#11488,#9816,.T.);
#14632=EDGE_CURVE('',#11502,#11494,#9817,.T.);
#14633=EDGE_CURVE('',#11508,#11500,#9818,.T.);
#14634=EDGE_CURVE('',#11514,#11506,#9819,.T.);
#14635=EDGE_CURVE('',#11520,#11512,#9820,.T.);
#14636=EDGE_CURVE('',#11522,#11518,#9821,.T.);
#14637=EDGE_CURVE('',#11522,#11523,#6567,.T.);
#14638=EDGE_CURVE('',#11523,#11524,#9822,.T.);
#14639=EDGE_CURVE('',#11524,#11525,#6568,.T.);
#14640=EDGE_CURVE('',#11315,#11525,#9823,.T.);
#14641=EDGE_CURVE('',#11526,#11524,#6569,.T.);
#14642=EDGE_CURVE('',#11526,#11527,#6570,.T.);
#14643=EDGE_CURVE('',#11525,#11527,#321,.T.);
#14644=EDGE_CURVE('',#11527,#11522,#322,.T.);
#14645=EDGE_CURVE('',#11523,#11526,#6571,.T.);
#14646=EDGE_CURVE('',#11528,#11528,#9824,.T.);
#14647=EDGE_CURVE('',#11528,#11417,#6572,.T.);
#14648=EDGE_CURVE('',#11529,#11530,#6573,.T.);
#14649=EDGE_CURVE('',#11530,#11530,#9825,.T.);
#14650=EDGE_CURVE('',#11531,#11532,#6574,.T.);
#14651=EDGE_CURVE('',#11531,#11533,#6575,.T.);
#14652=EDGE_CURVE('',#11533,#11534,#6576,.T.);
#14653=EDGE_CURVE('',#11532,#11534,#6577,.T.);
#14654=EDGE_CURVE('',#11535,#11531,#6578,.T.);
#14655=EDGE_CURVE('',#11535,#11536,#6579,.T.);
#14656=EDGE_CURVE('',#11536,#11533,#6580,.T.);
#14657=EDGE_CURVE('',#11537,#11535,#6581,.T.);
#14658=EDGE_CURVE('',#11537,#11538,#6582,.T.);
#14659=EDGE_CURVE('',#11538,#11536,#6583,.T.);
#14660=EDGE_CURVE('',#11539,#11537,#6584,.T.);
#14661=EDGE_CURVE('',#11539,#11540,#6585,.T.);
#14662=EDGE_CURVE('',#11540,#11538,#6586,.T.);
#14663=EDGE_CURVE('',#11541,#11539,#6587,.T.);
#14664=EDGE_CURVE('',#11541,#11542,#6588,.T.);
#14665=EDGE_CURVE('',#11542,#11540,#6589,.T.);
#14666=EDGE_CURVE('',#11532,#11541,#6590,.T.);
#14667=EDGE_CURVE('',#11534,#11542,#6591,.T.);
#14668=EDGE_CURVE('',#11543,#11543,#9826,.T.);
#14669=EDGE_CURVE('',#11189,#11543,#6592,.T.);
#14670=EDGE_CURVE('',#11306,#11308,#9827,.T.);
#14671=EDGE_CURVE('',#11544,#11544,#9828,.T.);
#14672=EDGE_CURVE('',#11544,#11307,#6593,.T.);
#19448=ORIENTED_EDGE('',*,*,#14132,.F.);
#19449=ORIENTED_EDGE('',*,*,#14133,.T.);
#19450=ORIENTED_EDGE('',*,*,#14134,.T.);
#19451=ORIENTED_EDGE('',*,*,#14135,.T.);
#19452=ORIENTED_EDGE('',*,*,#14136,.T.);
#19453=ORIENTED_EDGE('',*,*,#14135,.F.);
#19454=ORIENTED_EDGE('',*,*,#14137,.T.);
#19455=ORIENTED_EDGE('',*,*,#14138,.T.);
#19456=ORIENTED_EDGE('',*,*,#14139,.F.);
#19457=ORIENTED_EDGE('',*,*,#14140,.T.);
#19458=ORIENTED_EDGE('',*,*,#14132,.T.);
#19459=ORIENTED_EDGE('',*,*,#14141,.T.);
#19460=ORIENTED_EDGE('',*,*,#14142,.F.);
#19461=ORIENTED_EDGE('',*,*,#14143,.T.);
#19462=ORIENTED_EDGE('',*,*,#14139,.T.);
#19463=ORIENTED_EDGE('',*,*,#14144,.T.);
#19464=ORIENTED_EDGE('',*,*,#14145,.F.);
#19465=ORIENTED_EDGE('',*,*,#14146,.T.);
#19466=ORIENTED_EDGE('',*,*,#14142,.T.);
#19467=ORIENTED_EDGE('',*,*,#14147,.T.);
#19468=ORIENTED_EDGE('',*,*,#14148,.F.);
#19469=ORIENTED_EDGE('',*,*,#14149,.T.);
#19470=ORIENTED_EDGE('',*,*,#14145,.T.);
#19471=ORIENTED_EDGE('',*,*,#14150,.T.);
#19472=ORIENTED_EDGE('',*,*,#14151,.F.);
#19473=ORIENTED_EDGE('',*,*,#14152,.T.);
#19474=ORIENTED_EDGE('',*,*,#14148,.T.);
#19475=ORIENTED_EDGE('',*,*,#14153,.T.);
#19476=ORIENTED_EDGE('',*,*,#14154,.F.);
#19477=ORIENTED_EDGE('',*,*,#14155,.T.);
#19478=ORIENTED_EDGE('',*,*,#14151,.T.);
#19479=ORIENTED_EDGE('',*,*,#14156,.T.);
#19480=ORIENTED_EDGE('',*,*,#14157,.F.);
#19481=ORIENTED_EDGE('',*,*,#14158,.T.);
#19482=ORIENTED_EDGE('',*,*,#14154,.T.);
#19483=ORIENTED_EDGE('',*,*,#14159,.T.);
#19484=ORIENTED_EDGE('',*,*,#14160,.F.);
#19485=ORIENTED_EDGE('',*,*,#14161,.T.);
#19486=ORIENTED_EDGE('',*,*,#14157,.T.);
#19487=ORIENTED_EDGE('',*,*,#14162,.T.);
#19488=ORIENTED_EDGE('',*,*,#14163,.F.);
#19489=ORIENTED_EDGE('',*,*,#14164,.T.);
#19490=ORIENTED_EDGE('',*,*,#14160,.T.);
#19491=ORIENTED_EDGE('',*,*,#14165,.T.);
#19492=ORIENTED_EDGE('',*,*,#14166,.F.);
#19493=ORIENTED_EDGE('',*,*,#14167,.T.);
#19494=ORIENTED_EDGE('',*,*,#14163,.T.);
#19495=ORIENTED_EDGE('',*,*,#14168,.T.);
#19496=ORIENTED_EDGE('',*,*,#14169,.F.);
#19497=ORIENTED_EDGE('',*,*,#14170,.T.);
#19498=ORIENTED_EDGE('',*,*,#14166,.T.);
#19499=ORIENTED_EDGE('',*,*,#14171,.T.);
#19500=ORIENTED_EDGE('',*,*,#14172,.F.);
#19501=ORIENTED_EDGE('',*,*,#14173,.T.);
#19502=ORIENTED_EDGE('',*,*,#14169,.T.);
#19503=ORIENTED_EDGE('',*,*,#14174,.T.);
#19504=ORIENTED_EDGE('',*,*,#14175,.F.);
#19505=ORIENTED_EDGE('',*,*,#14176,.T.);
#19506=ORIENTED_EDGE('',*,*,#14172,.T.);
#19507=ORIENTED_EDGE('',*,*,#14177,.T.);
#19508=ORIENTED_EDGE('',*,*,#14178,.F.);
#19509=ORIENTED_EDGE('',*,*,#14179,.T.);
#19510=ORIENTED_EDGE('',*,*,#14175,.T.);
#19511=ORIENTED_EDGE('',*,*,#14180,.T.);
#19512=ORIENTED_EDGE('',*,*,#14181,.F.);
#19513=ORIENTED_EDGE('',*,*,#14182,.T.);
#19514=ORIENTED_EDGE('',*,*,#14178,.T.);
#19515=ORIENTED_EDGE('',*,*,#14183,.T.);
#19516=ORIENTED_EDGE('',*,*,#14184,.F.);
#19517=ORIENTED_EDGE('',*,*,#14185,.T.);
#19518=ORIENTED_EDGE('',*,*,#14181,.T.);
#19519=ORIENTED_EDGE('',*,*,#14186,.T.);
#19520=ORIENTED_EDGE('',*,*,#14187,.F.);
#19521=ORIENTED_EDGE('',*,*,#14188,.T.);
#19522=ORIENTED_EDGE('',*,*,#14184,.T.);
#19523=ORIENTED_EDGE('',*,*,#14189,.T.);
#19524=ORIENTED_EDGE('',*,*,#14190,.F.);
#19525=ORIENTED_EDGE('',*,*,#14191,.T.);
#19526=ORIENTED_EDGE('',*,*,#14187,.T.);
#19527=ORIENTED_EDGE('',*,*,#14192,.T.);
#19528=ORIENTED_EDGE('',*,*,#14193,.F.);
#19529=ORIENTED_EDGE('',*,*,#14194,.T.);
#19530=ORIENTED_EDGE('',*,*,#14190,.T.);
#19531=ORIENTED_EDGE('',*,*,#14195,.T.);
#19532=ORIENTED_EDGE('',*,*,#14196,.F.);
#19533=ORIENTED_EDGE('',*,*,#14197,.T.);
#19534=ORIENTED_EDGE('',*,*,#14193,.T.);
#19535=ORIENTED_EDGE('',*,*,#14198,.T.);
#19536=ORIENTED_EDGE('',*,*,#14199,.F.);
#19537=ORIENTED_EDGE('',*,*,#14200,.T.);
#19538=ORIENTED_EDGE('',*,*,#14196,.T.);
#19539=ORIENTED_EDGE('',*,*,#14201,.T.);
#19540=ORIENTED_EDGE('',*,*,#14202,.F.);
#19541=ORIENTED_EDGE('',*,*,#14203,.T.);
#19542=ORIENTED_EDGE('',*,*,#14199,.T.);
#19543=ORIENTED_EDGE('',*,*,#14204,.T.);
#19544=ORIENTED_EDGE('',*,*,#14205,.F.);
#19545=ORIENTED_EDGE('',*,*,#14206,.T.);
#19546=ORIENTED_EDGE('',*,*,#14202,.T.);
#19547=ORIENTED_EDGE('',*,*,#14207,.T.);
#19548=ORIENTED_EDGE('',*,*,#14208,.F.);
#19549=ORIENTED_EDGE('',*,*,#14209,.T.);
#19550=ORIENTED_EDGE('',*,*,#14205,.T.);
#19551=ORIENTED_EDGE('',*,*,#14210,.T.);
#19552=ORIENTED_EDGE('',*,*,#14211,.F.);
#19553=ORIENTED_EDGE('',*,*,#14212,.T.);
#19554=ORIENTED_EDGE('',*,*,#14208,.T.);
#19555=ORIENTED_EDGE('',*,*,#14213,.T.);
#19556=ORIENTED_EDGE('',*,*,#14214,.F.);
#19557=ORIENTED_EDGE('',*,*,#14215,.T.);
#19558=ORIENTED_EDGE('',*,*,#14211,.T.);
#19559=ORIENTED_EDGE('',*,*,#14216,.T.);
#19560=ORIENTED_EDGE('',*,*,#14217,.F.);
#19561=ORIENTED_EDGE('',*,*,#14218,.T.);
#19562=ORIENTED_EDGE('',*,*,#14214,.T.);
#19563=ORIENTED_EDGE('',*,*,#14219,.T.);
#19564=ORIENTED_EDGE('',*,*,#14220,.F.);
#19565=ORIENTED_EDGE('',*,*,#14221,.T.);
#19566=ORIENTED_EDGE('',*,*,#14222,.F.);
#19567=ORIENTED_EDGE('',*,*,#14223,.F.);
#19568=ORIENTED_EDGE('',*,*,#14224,.F.);
#19569=ORIENTED_EDGE('',*,*,#14225,.T.);
#19570=ORIENTED_EDGE('',*,*,#14220,.T.);
#19571=ORIENTED_EDGE('',*,*,#14226,.F.);
#19572=ORIENTED_EDGE('',*,*,#14227,.F.);
#19573=ORIENTED_EDGE('',*,*,#14228,.T.);
#19574=ORIENTED_EDGE('',*,*,#14224,.T.);
#19575=ORIENTED_EDGE('',*,*,#14229,.F.);
#19576=ORIENTED_EDGE('',*,*,#14230,.F.);
#19577=ORIENTED_EDGE('',*,*,#14231,.T.);
#19578=ORIENTED_EDGE('',*,*,#14227,.T.);
#19579=ORIENTED_EDGE('',*,*,#14232,.F.);
#19580=ORIENTED_EDGE('',*,*,#14233,.F.);
#19581=ORIENTED_EDGE('',*,*,#14234,.T.);
#19582=ORIENTED_EDGE('',*,*,#14230,.T.);
#19583=ORIENTED_EDGE('',*,*,#14235,.F.);
#19584=ORIENTED_EDGE('',*,*,#14236,.F.);
#19585=ORIENTED_EDGE('',*,*,#14237,.T.);
#19586=ORIENTED_EDGE('',*,*,#14233,.T.);
#19587=ORIENTED_EDGE('',*,*,#14238,.F.);
#19588=ORIENTED_EDGE('',*,*,#14239,.F.);
#19589=ORIENTED_EDGE('',*,*,#14240,.T.);
#19590=ORIENTED_EDGE('',*,*,#14236,.T.);
#19591=ORIENTED_EDGE('',*,*,#14241,.F.);
#19592=ORIENTED_EDGE('',*,*,#14242,.F.);
#19593=ORIENTED_EDGE('',*,*,#14243,.T.);
#19594=ORIENTED_EDGE('',*,*,#14239,.T.);
#19595=ORIENTED_EDGE('',*,*,#14244,.F.);
#19596=ORIENTED_EDGE('',*,*,#14245,.F.);
#19597=ORIENTED_EDGE('',*,*,#14246,.T.);
#19598=ORIENTED_EDGE('',*,*,#14242,.T.);
#19599=ORIENTED_EDGE('',*,*,#14247,.F.);
#19600=ORIENTED_EDGE('',*,*,#14248,.F.);
#19601=ORIENTED_EDGE('',*,*,#14249,.T.);
#19602=ORIENTED_EDGE('',*,*,#14245,.T.);
#19603=ORIENTED_EDGE('',*,*,#14250,.F.);
#19604=ORIENTED_EDGE('',*,*,#14251,.F.);
#19605=ORIENTED_EDGE('',*,*,#14252,.T.);
#19606=ORIENTED_EDGE('',*,*,#14248,.T.);
#19607=ORIENTED_EDGE('',*,*,#14253,.F.);
#19608=ORIENTED_EDGE('',*,*,#14254,.F.);
#19609=ORIENTED_EDGE('',*,*,#14255,.T.);
#19610=ORIENTED_EDGE('',*,*,#14251,.T.);
#19611=ORIENTED_EDGE('',*,*,#14256,.F.);
#19612=ORIENTED_EDGE('',*,*,#14257,.F.);
#19613=ORIENTED_EDGE('',*,*,#14258,.T.);
#19614=ORIENTED_EDGE('',*,*,#14254,.T.);
#19615=ORIENTED_EDGE('',*,*,#14259,.F.);
#19616=ORIENTED_EDGE('',*,*,#14260,.F.);
#19617=ORIENTED_EDGE('',*,*,#14261,.T.);
#19618=ORIENTED_EDGE('',*,*,#14257,.T.);
#19619=ORIENTED_EDGE('',*,*,#14262,.F.);
#19620=ORIENTED_EDGE('',*,*,#14263,.F.);
#19621=ORIENTED_EDGE('',*,*,#14264,.T.);
#19622=ORIENTED_EDGE('',*,*,#14260,.T.);
#19623=ORIENTED_EDGE('',*,*,#14265,.F.);
#19624=ORIENTED_EDGE('',*,*,#14266,.F.);
#19625=ORIENTED_EDGE('',*,*,#14267,.T.);
#19626=ORIENTED_EDGE('',*,*,#14263,.T.);
#19627=ORIENTED_EDGE('',*,*,#14268,.F.);
#19628=ORIENTED_EDGE('',*,*,#14269,.F.);
#19629=ORIENTED_EDGE('',*,*,#14270,.T.);
#19630=ORIENTED_EDGE('',*,*,#14266,.T.);
#19631=ORIENTED_EDGE('',*,*,#14271,.F.);
#19632=ORIENTED_EDGE('',*,*,#14272,.F.);
#19633=ORIENTED_EDGE('',*,*,#14273,.T.);
#19634=ORIENTED_EDGE('',*,*,#14269,.T.);
#19635=ORIENTED_EDGE('',*,*,#14274,.F.);
#19636=ORIENTED_EDGE('',*,*,#14275,.F.);
#19637=ORIENTED_EDGE('',*,*,#14276,.T.);
#19638=ORIENTED_EDGE('',*,*,#14272,.T.);
#19639=ORIENTED_EDGE('',*,*,#14277,.F.);
#19640=ORIENTED_EDGE('',*,*,#14278,.F.);
#19641=ORIENTED_EDGE('',*,*,#14279,.T.);
#19642=ORIENTED_EDGE('',*,*,#14275,.T.);
#19643=ORIENTED_EDGE('',*,*,#14280,.F.);
#19644=ORIENTED_EDGE('',*,*,#14281,.F.);
#19645=ORIENTED_EDGE('',*,*,#14282,.T.);
#19646=ORIENTED_EDGE('',*,*,#14278,.T.);
#19647=ORIENTED_EDGE('',*,*,#14283,.F.);
#19648=ORIENTED_EDGE('',*,*,#14284,.F.);
#19649=ORIENTED_EDGE('',*,*,#14285,.T.);
#19650=ORIENTED_EDGE('',*,*,#14281,.T.);
#19651=ORIENTED_EDGE('',*,*,#14286,.F.);
#19652=ORIENTED_EDGE('',*,*,#14287,.F.);
#19653=ORIENTED_EDGE('',*,*,#14288,.T.);
#19654=ORIENTED_EDGE('',*,*,#14284,.T.);
#19655=ORIENTED_EDGE('',*,*,#14289,.F.);
#19656=ORIENTED_EDGE('',*,*,#14290,.F.);
#19657=ORIENTED_EDGE('',*,*,#14291,.T.);
#19658=ORIENTED_EDGE('',*,*,#14287,.T.);
#19659=ORIENTED_EDGE('',*,*,#14292,.F.);
#19660=ORIENTED_EDGE('',*,*,#14293,.F.);
#19661=ORIENTED_EDGE('',*,*,#14294,.T.);
#19662=ORIENTED_EDGE('',*,*,#14290,.T.);
#19663=ORIENTED_EDGE('',*,*,#14295,.F.);
#19664=ORIENTED_EDGE('',*,*,#14296,.F.);
#19665=ORIENTED_EDGE('',*,*,#14297,.T.);
#19666=ORIENTED_EDGE('',*,*,#14293,.T.);
#19667=ORIENTED_EDGE('',*,*,#14298,.F.);
#19668=ORIENTED_EDGE('',*,*,#14299,.F.);
#19669=ORIENTED_EDGE('',*,*,#14300,.T.);
#19670=ORIENTED_EDGE('',*,*,#14296,.T.);
#19671=ORIENTED_EDGE('',*,*,#14301,.F.);
#19672=ORIENTED_EDGE('',*,*,#14302,.F.);
#19673=ORIENTED_EDGE('',*,*,#14303,.T.);
#19674=ORIENTED_EDGE('',*,*,#14299,.T.);
#19675=ORIENTED_EDGE('',*,*,#14304,.F.);
#19676=ORIENTED_EDGE('',*,*,#14305,.F.);
#19677=ORIENTED_EDGE('',*,*,#14306,.F.);
#19678=ORIENTED_EDGE('',*,*,#14307,.T.);
#19679=ORIENTED_EDGE('',*,*,#14302,.T.);
#19680=ORIENTED_EDGE('',*,*,#14308,.F.);
#19681=ORIENTED_EDGE('',*,*,#14222,.T.);
#19682=ORIENTED_EDGE('',*,*,#14309,.T.);
#19683=ORIENTED_EDGE('',*,*,#14310,.F.);
#19684=ORIENTED_EDGE('',*,*,#14311,.F.);
#19685=ORIENTED_EDGE('',*,*,#14312,.T.);
#19686=ORIENTED_EDGE('',*,*,#14312,.F.);
#19687=ORIENTED_EDGE('',*,*,#14313,.F.);
#19688=ORIENTED_EDGE('',*,*,#14219,.F.);
#19689=ORIENTED_EDGE('',*,*,#14216,.F.);
#19690=ORIENTED_EDGE('',*,*,#14213,.F.);
#19691=ORIENTED_EDGE('',*,*,#14210,.F.);
#19692=ORIENTED_EDGE('',*,*,#14207,.F.);
#19693=ORIENTED_EDGE('',*,*,#14204,.F.);
#19694=ORIENTED_EDGE('',*,*,#14201,.F.);
#19695=ORIENTED_EDGE('',*,*,#14198,.F.);
#19696=ORIENTED_EDGE('',*,*,#14195,.F.);
#19697=ORIENTED_EDGE('',*,*,#14192,.F.);
#19698=ORIENTED_EDGE('',*,*,#14189,.F.);
#19699=ORIENTED_EDGE('',*,*,#14186,.F.);
#19700=ORIENTED_EDGE('',*,*,#14183,.F.);
#19701=ORIENTED_EDGE('',*,*,#14180,.F.);
#19702=ORIENTED_EDGE('',*,*,#14177,.F.);
#19703=ORIENTED_EDGE('',*,*,#14174,.F.);
#19704=ORIENTED_EDGE('',*,*,#14171,.F.);
#19705=ORIENTED_EDGE('',*,*,#14168,.F.);
#19706=ORIENTED_EDGE('',*,*,#14165,.F.);
#19707=ORIENTED_EDGE('',*,*,#14162,.F.);
#19708=ORIENTED_EDGE('',*,*,#14159,.F.);
#19709=ORIENTED_EDGE('',*,*,#14156,.F.);
#19710=ORIENTED_EDGE('',*,*,#14153,.F.);
#19711=ORIENTED_EDGE('',*,*,#14150,.F.);
#19712=ORIENTED_EDGE('',*,*,#14147,.F.);
#19713=ORIENTED_EDGE('',*,*,#14144,.F.);
#19714=ORIENTED_EDGE('',*,*,#14141,.F.);
#19715=ORIENTED_EDGE('',*,*,#14138,.F.);
#19716=ORIENTED_EDGE('',*,*,#14314,.F.);
#19717=ORIENTED_EDGE('',*,*,#14315,.T.);
#19718=ORIENTED_EDGE('',*,*,#14308,.T.);
#19719=ORIENTED_EDGE('',*,*,#14304,.T.);
#19720=ORIENTED_EDGE('',*,*,#14301,.T.);
#19721=ORIENTED_EDGE('',*,*,#14298,.T.);
#19722=ORIENTED_EDGE('',*,*,#14295,.T.);
#19723=ORIENTED_EDGE('',*,*,#14292,.T.);
#19724=ORIENTED_EDGE('',*,*,#14289,.T.);
#19725=ORIENTED_EDGE('',*,*,#14286,.T.);
#19726=ORIENTED_EDGE('',*,*,#14283,.T.);
#19727=ORIENTED_EDGE('',*,*,#14280,.T.);
#19728=ORIENTED_EDGE('',*,*,#14277,.T.);
#19729=ORIENTED_EDGE('',*,*,#14274,.T.);
#19730=ORIENTED_EDGE('',*,*,#14271,.T.);
#19731=ORIENTED_EDGE('',*,*,#14268,.T.);
#19732=ORIENTED_EDGE('',*,*,#14265,.T.);
#19733=ORIENTED_EDGE('',*,*,#14262,.T.);
#19734=ORIENTED_EDGE('',*,*,#14259,.T.);
#19735=ORIENTED_EDGE('',*,*,#14256,.T.);
#19736=ORIENTED_EDGE('',*,*,#14253,.T.);
#19737=ORIENTED_EDGE('',*,*,#14250,.T.);
#19738=ORIENTED_EDGE('',*,*,#14247,.T.);
#19739=ORIENTED_EDGE('',*,*,#14244,.T.);
#19740=ORIENTED_EDGE('',*,*,#14241,.T.);
#19741=ORIENTED_EDGE('',*,*,#14238,.T.);
#19742=ORIENTED_EDGE('',*,*,#14235,.T.);
#19743=ORIENTED_EDGE('',*,*,#14232,.T.);
#19744=ORIENTED_EDGE('',*,*,#14229,.T.);
#19745=ORIENTED_EDGE('',*,*,#14226,.T.);
#19746=ORIENTED_EDGE('',*,*,#14223,.T.);
#19747=ORIENTED_EDGE('',*,*,#14134,.F.);
#19748=ORIENTED_EDGE('',*,*,#14316,.T.);
#19749=ORIENTED_EDGE('',*,*,#14306,.T.);
#19750=ORIENTED_EDGE('',*,*,#14317,.T.);
#19751=ORIENTED_EDGE('',*,*,#14314,.T.);
#19752=ORIENTED_EDGE('',*,*,#14137,.F.);
#19753=ORIENTED_EDGE('',*,*,#14305,.T.);
#19754=ORIENTED_EDGE('',*,*,#14315,.F.);
#19755=ORIENTED_EDGE('',*,*,#14317,.F.);
#19756=ORIENTED_EDGE('',*,*,#14309,.F.);
#19757=ORIENTED_EDGE('',*,*,#14221,.F.);
#19758=ORIENTED_EDGE('',*,*,#14225,.F.);
#19759=ORIENTED_EDGE('',*,*,#14228,.F.);
#19760=ORIENTED_EDGE('',*,*,#14231,.F.);
#19761=ORIENTED_EDGE('',*,*,#14234,.F.);
#19762=ORIENTED_EDGE('',*,*,#14237,.F.);
#19763=ORIENTED_EDGE('',*,*,#14240,.F.);
#19764=ORIENTED_EDGE('',*,*,#14243,.F.);
#19765=ORIENTED_EDGE('',*,*,#14246,.F.);
#19766=ORIENTED_EDGE('',*,*,#14249,.F.);
#19767=ORIENTED_EDGE('',*,*,#14252,.F.);
#19768=ORIENTED_EDGE('',*,*,#14255,.F.);
#19769=ORIENTED_EDGE('',*,*,#14258,.F.);
#19770=ORIENTED_EDGE('',*,*,#14261,.F.);
#19771=ORIENTED_EDGE('',*,*,#14264,.F.);
#19772=ORIENTED_EDGE('',*,*,#14267,.F.);
#19773=ORIENTED_EDGE('',*,*,#14270,.F.);
#19774=ORIENTED_EDGE('',*,*,#14273,.F.);
#19775=ORIENTED_EDGE('',*,*,#14276,.F.);
#19776=ORIENTED_EDGE('',*,*,#14279,.F.);
#19777=ORIENTED_EDGE('',*,*,#14282,.F.);
#19778=ORIENTED_EDGE('',*,*,#14285,.F.);
#19779=ORIENTED_EDGE('',*,*,#14288,.F.);
#19780=ORIENTED_EDGE('',*,*,#14291,.F.);
#19781=ORIENTED_EDGE('',*,*,#14294,.F.);
#19782=ORIENTED_EDGE('',*,*,#14297,.F.);
#19783=ORIENTED_EDGE('',*,*,#14300,.F.);
#19784=ORIENTED_EDGE('',*,*,#14303,.F.);
#19785=ORIENTED_EDGE('',*,*,#14307,.F.);
#19786=ORIENTED_EDGE('',*,*,#14316,.F.);
#19787=ORIENTED_EDGE('',*,*,#14133,.F.);
#19788=ORIENTED_EDGE('',*,*,#14140,.F.);
#19789=ORIENTED_EDGE('',*,*,#14143,.F.);
#19790=ORIENTED_EDGE('',*,*,#14146,.F.);
#19791=ORIENTED_EDGE('',*,*,#14149,.F.);
#19792=ORIENTED_EDGE('',*,*,#14152,.F.);
#19793=ORIENTED_EDGE('',*,*,#14155,.F.);
#19794=ORIENTED_EDGE('',*,*,#14158,.F.);
#19795=ORIENTED_EDGE('',*,*,#14161,.F.);
#19796=ORIENTED_EDGE('',*,*,#14164,.F.);
#19797=ORIENTED_EDGE('',*,*,#14167,.F.);
#19798=ORIENTED_EDGE('',*,*,#14170,.F.);
#19799=ORIENTED_EDGE('',*,*,#14173,.F.);
#19800=ORIENTED_EDGE('',*,*,#14176,.F.);
#19801=ORIENTED_EDGE('',*,*,#14179,.F.);
#19802=ORIENTED_EDGE('',*,*,#14182,.F.);
#19803=ORIENTED_EDGE('',*,*,#14185,.F.);
#19804=ORIENTED_EDGE('',*,*,#14188,.F.);
#19805=ORIENTED_EDGE('',*,*,#14191,.F.);
#19806=ORIENTED_EDGE('',*,*,#14194,.F.);
#19807=ORIENTED_EDGE('',*,*,#14197,.F.);
#19808=ORIENTED_EDGE('',*,*,#14200,.F.);
#19809=ORIENTED_EDGE('',*,*,#14203,.F.);
#19810=ORIENTED_EDGE('',*,*,#14206,.F.);
#19811=ORIENTED_EDGE('',*,*,#14209,.F.);
#19812=ORIENTED_EDGE('',*,*,#14212,.F.);
#19813=ORIENTED_EDGE('',*,*,#14215,.F.);
#19814=ORIENTED_EDGE('',*,*,#14218,.F.);
#19815=ORIENTED_EDGE('',*,*,#14318,.F.);
#19816=ORIENTED_EDGE('',*,*,#14319,.F.);
#19817=ORIENTED_EDGE('',*,*,#14320,.T.);
#19818=ORIENTED_EDGE('',*,*,#14321,.T.);
#19819=ORIENTED_EDGE('',*,*,#14322,.F.);
#19820=ORIENTED_EDGE('',*,*,#14321,.F.);
#19821=ORIENTED_EDGE('',*,*,#14323,.T.);
#19822=ORIENTED_EDGE('',*,*,#14324,.F.);
#19823=ORIENTED_EDGE('',*,*,#14325,.F.);
#19824=ORIENTED_EDGE('',*,*,#14326,.F.);
#19825=ORIENTED_EDGE('',*,*,#14323,.F.);
#19826=ORIENTED_EDGE('',*,*,#14320,.F.);
#19827=ORIENTED_EDGE('',*,*,#14327,.F.);
#19828=ORIENTED_EDGE('',*,*,#14328,.T.);
#19829=ORIENTED_EDGE('',*,*,#14329,.T.);
#19830=ORIENTED_EDGE('',*,*,#14330,.F.);
#19831=ORIENTED_EDGE('',*,*,#14329,.F.);
#19832=ORIENTED_EDGE('',*,*,#14331,.T.);
#19833=ORIENTED_EDGE('',*,*,#14332,.F.);
#19834=ORIENTED_EDGE('',*,*,#14333,.F.);
#19835=ORIENTED_EDGE('',*,*,#14334,.F.);
#19836=ORIENTED_EDGE('',*,*,#14331,.F.);
#19837=ORIENTED_EDGE('',*,*,#14328,.F.);
#19838=ORIENTED_EDGE('',*,*,#14335,.F.);
#19839=ORIENTED_EDGE('',*,*,#14336,.T.);
#19840=ORIENTED_EDGE('',*,*,#14337,.T.);
#19841=ORIENTED_EDGE('',*,*,#14338,.F.);
#19842=ORIENTED_EDGE('',*,*,#14337,.F.);
#19843=ORIENTED_EDGE('',*,*,#14339,.T.);
#19844=ORIENTED_EDGE('',*,*,#14340,.F.);
#19845=ORIENTED_EDGE('',*,*,#14341,.F.);
#19846=ORIENTED_EDGE('',*,*,#14342,.F.);
#19847=ORIENTED_EDGE('',*,*,#14339,.F.);
#19848=ORIENTED_EDGE('',*,*,#14336,.F.);
#19849=ORIENTED_EDGE('',*,*,#14343,.F.);
#19850=ORIENTED_EDGE('',*,*,#14344,.T.);
#19851=ORIENTED_EDGE('',*,*,#14345,.T.);
#19852=ORIENTED_EDGE('',*,*,#14346,.F.);
#19853=ORIENTED_EDGE('',*,*,#14345,.F.);
#19854=ORIENTED_EDGE('',*,*,#14347,.T.);
#19855=ORIENTED_EDGE('',*,*,#14348,.F.);
#19856=ORIENTED_EDGE('',*,*,#14349,.F.);
#19857=ORIENTED_EDGE('',*,*,#14350,.F.);
#19858=ORIENTED_EDGE('',*,*,#14347,.F.);
#19859=ORIENTED_EDGE('',*,*,#14344,.F.);
#19860=ORIENTED_EDGE('',*,*,#14351,.F.);
#19861=ORIENTED_EDGE('',*,*,#14352,.T.);
#19862=ORIENTED_EDGE('',*,*,#14353,.T.);
#19863=ORIENTED_EDGE('',*,*,#14354,.F.);
#19864=ORIENTED_EDGE('',*,*,#14353,.F.);
#19865=ORIENTED_EDGE('',*,*,#14355,.T.);
#19866=ORIENTED_EDGE('',*,*,#14356,.F.);
#19867=ORIENTED_EDGE('',*,*,#14357,.F.);
#19868=ORIENTED_EDGE('',*,*,#14358,.F.);
#19869=ORIENTED_EDGE('',*,*,#14355,.F.);
#19870=ORIENTED_EDGE('',*,*,#14352,.F.);
#19871=ORIENTED_EDGE('',*,*,#14359,.F.);
#19872=ORIENTED_EDGE('',*,*,#14360,.T.);
#19873=ORIENTED_EDGE('',*,*,#14361,.T.);
#19874=ORIENTED_EDGE('',*,*,#14362,.F.);
#19875=ORIENTED_EDGE('',*,*,#14361,.F.);
#19876=ORIENTED_EDGE('',*,*,#14363,.T.);
#19877=ORIENTED_EDGE('',*,*,#14364,.F.);
#19878=ORIENTED_EDGE('',*,*,#14365,.F.);
#19879=ORIENTED_EDGE('',*,*,#14366,.F.);
#19880=ORIENTED_EDGE('',*,*,#14363,.F.);
#19881=ORIENTED_EDGE('',*,*,#14360,.F.);
#19882=ORIENTED_EDGE('',*,*,#14367,.F.);
#19883=ORIENTED_EDGE('',*,*,#14368,.T.);
#19884=ORIENTED_EDGE('',*,*,#14369,.T.);
#19885=ORIENTED_EDGE('',*,*,#14370,.F.);
#19886=ORIENTED_EDGE('',*,*,#14369,.F.);
#19887=ORIENTED_EDGE('',*,*,#14371,.T.);
#19888=ORIENTED_EDGE('',*,*,#14372,.F.);
#19889=ORIENTED_EDGE('',*,*,#14373,.F.);
#19890=ORIENTED_EDGE('',*,*,#14374,.F.);
#19891=ORIENTED_EDGE('',*,*,#14371,.F.);
#19892=ORIENTED_EDGE('',*,*,#14368,.F.);
#19893=ORIENTED_EDGE('',*,*,#14375,.F.);
#19894=ORIENTED_EDGE('',*,*,#14376,.T.);
#19895=ORIENTED_EDGE('',*,*,#14377,.T.);
#19896=ORIENTED_EDGE('',*,*,#14378,.F.);
#19897=ORIENTED_EDGE('',*,*,#14377,.F.);
#19898=ORIENTED_EDGE('',*,*,#14379,.T.);
#19899=ORIENTED_EDGE('',*,*,#14380,.F.);
#19900=ORIENTED_EDGE('',*,*,#14381,.F.);
#19901=ORIENTED_EDGE('',*,*,#14382,.F.);
#19902=ORIENTED_EDGE('',*,*,#14379,.F.);
#19903=ORIENTED_EDGE('',*,*,#14376,.F.);
#19904=ORIENTED_EDGE('',*,*,#14383,.F.);
#19905=ORIENTED_EDGE('',*,*,#14384,.T.);
#19906=ORIENTED_EDGE('',*,*,#14385,.T.);
#19907=ORIENTED_EDGE('',*,*,#14386,.F.);
#19908=ORIENTED_EDGE('',*,*,#14385,.F.);
#19909=ORIENTED_EDGE('',*,*,#14387,.T.);
#19910=ORIENTED_EDGE('',*,*,#14388,.F.);
#19911=ORIENTED_EDGE('',*,*,#14389,.F.);
#19912=ORIENTED_EDGE('',*,*,#14390,.F.);
#19913=ORIENTED_EDGE('',*,*,#14387,.F.);
#19914=ORIENTED_EDGE('',*,*,#14384,.F.);
#19915=ORIENTED_EDGE('',*,*,#14391,.F.);
#19916=ORIENTED_EDGE('',*,*,#14392,.T.);
#19917=ORIENTED_EDGE('',*,*,#14393,.T.);
#19918=ORIENTED_EDGE('',*,*,#14394,.F.);
#19919=ORIENTED_EDGE('',*,*,#14393,.F.);
#19920=ORIENTED_EDGE('',*,*,#14395,.T.);
#19921=ORIENTED_EDGE('',*,*,#14396,.F.);
#19922=ORIENTED_EDGE('',*,*,#14397,.F.);
#19923=ORIENTED_EDGE('',*,*,#14398,.F.);
#19924=ORIENTED_EDGE('',*,*,#14395,.F.);
#19925=ORIENTED_EDGE('',*,*,#14392,.F.);
#19926=ORIENTED_EDGE('',*,*,#14399,.F.);
#19927=ORIENTED_EDGE('',*,*,#14400,.T.);
#19928=ORIENTED_EDGE('',*,*,#14401,.T.);
#19929=ORIENTED_EDGE('',*,*,#14402,.F.);
#19930=ORIENTED_EDGE('',*,*,#14401,.F.);
#19931=ORIENTED_EDGE('',*,*,#14403,.T.);
#19932=ORIENTED_EDGE('',*,*,#14404,.F.);
#19933=ORIENTED_EDGE('',*,*,#14405,.F.);
#19934=ORIENTED_EDGE('',*,*,#14406,.F.);
#19935=ORIENTED_EDGE('',*,*,#14403,.F.);
#19936=ORIENTED_EDGE('',*,*,#14400,.F.);
#19937=ORIENTED_EDGE('',*,*,#14407,.F.);
#19938=ORIENTED_EDGE('',*,*,#14408,.T.);
#19939=ORIENTED_EDGE('',*,*,#14409,.T.);
#19940=ORIENTED_EDGE('',*,*,#14410,.F.);
#19941=ORIENTED_EDGE('',*,*,#14409,.F.);
#19942=ORIENTED_EDGE('',*,*,#14411,.T.);
#19943=ORIENTED_EDGE('',*,*,#14412,.F.);
#19944=ORIENTED_EDGE('',*,*,#14413,.F.);
#19945=ORIENTED_EDGE('',*,*,#14414,.F.);
#19946=ORIENTED_EDGE('',*,*,#14411,.F.);
#19947=ORIENTED_EDGE('',*,*,#14408,.F.);
#19948=ORIENTED_EDGE('',*,*,#14415,.F.);
#19949=ORIENTED_EDGE('',*,*,#14416,.T.);
#19950=ORIENTED_EDGE('',*,*,#14417,.T.);
#19951=ORIENTED_EDGE('',*,*,#14418,.F.);
#19952=ORIENTED_EDGE('',*,*,#14417,.F.);
#19953=ORIENTED_EDGE('',*,*,#14419,.T.);
#19954=ORIENTED_EDGE('',*,*,#14420,.F.);
#19955=ORIENTED_EDGE('',*,*,#14421,.F.);
#19956=ORIENTED_EDGE('',*,*,#14422,.F.);
#19957=ORIENTED_EDGE('',*,*,#14419,.F.);
#19958=ORIENTED_EDGE('',*,*,#14416,.F.);
#19959=ORIENTED_EDGE('',*,*,#14423,.F.);
#19960=ORIENTED_EDGE('',*,*,#14424,.T.);
#19961=ORIENTED_EDGE('',*,*,#14425,.T.);
#19962=ORIENTED_EDGE('',*,*,#14426,.F.);
#19963=ORIENTED_EDGE('',*,*,#14425,.F.);
#19964=ORIENTED_EDGE('',*,*,#14427,.T.);
#19965=ORIENTED_EDGE('',*,*,#14428,.F.);
#19966=ORIENTED_EDGE('',*,*,#14429,.F.);
#19967=ORIENTED_EDGE('',*,*,#14430,.F.);
#19968=ORIENTED_EDGE('',*,*,#14427,.F.);
#19969=ORIENTED_EDGE('',*,*,#14424,.F.);
#19970=ORIENTED_EDGE('',*,*,#14431,.F.);
#19971=ORIENTED_EDGE('',*,*,#14432,.T.);
#19972=ORIENTED_EDGE('',*,*,#14433,.T.);
#19973=ORIENTED_EDGE('',*,*,#14434,.F.);
#19974=ORIENTED_EDGE('',*,*,#14433,.F.);
#19975=ORIENTED_EDGE('',*,*,#14435,.T.);
#19976=ORIENTED_EDGE('',*,*,#14436,.F.);
#19977=ORIENTED_EDGE('',*,*,#14437,.F.);
#19978=ORIENTED_EDGE('',*,*,#14438,.F.);
#19979=ORIENTED_EDGE('',*,*,#14435,.F.);
#19980=ORIENTED_EDGE('',*,*,#14432,.F.);
#19981=ORIENTED_EDGE('',*,*,#14439,.F.);
#19982=ORIENTED_EDGE('',*,*,#14440,.T.);
#19983=ORIENTED_EDGE('',*,*,#14441,.T.);
#19984=ORIENTED_EDGE('',*,*,#14442,.F.);
#19985=ORIENTED_EDGE('',*,*,#14441,.F.);
#19986=ORIENTED_EDGE('',*,*,#14443,.T.);
#19987=ORIENTED_EDGE('',*,*,#14444,.F.);
#19988=ORIENTED_EDGE('',*,*,#14445,.F.);
#19989=ORIENTED_EDGE('',*,*,#14446,.F.);
#19990=ORIENTED_EDGE('',*,*,#14443,.F.);
#19991=ORIENTED_EDGE('',*,*,#14440,.F.);
#19992=ORIENTED_EDGE('',*,*,#14447,.F.);
#19993=ORIENTED_EDGE('',*,*,#14448,.T.);
#19994=ORIENTED_EDGE('',*,*,#14449,.T.);
#19995=ORIENTED_EDGE('',*,*,#14450,.F.);
#19996=ORIENTED_EDGE('',*,*,#14449,.F.);
#19997=ORIENTED_EDGE('',*,*,#14451,.T.);
#19998=ORIENTED_EDGE('',*,*,#14452,.F.);
#19999=ORIENTED_EDGE('',*,*,#14453,.F.);
#20000=ORIENTED_EDGE('',*,*,#14454,.F.);
#20001=ORIENTED_EDGE('',*,*,#14451,.F.);
#20002=ORIENTED_EDGE('',*,*,#14448,.F.);
#20003=ORIENTED_EDGE('',*,*,#14455,.F.);
#20004=ORIENTED_EDGE('',*,*,#14456,.T.);
#20005=ORIENTED_EDGE('',*,*,#14457,.T.);
#20006=ORIENTED_EDGE('',*,*,#14458,.F.);
#20007=ORIENTED_EDGE('',*,*,#14459,.F.);
#20008=ORIENTED_EDGE('',*,*,#14457,.F.);
#20009=ORIENTED_EDGE('',*,*,#14460,.T.);
#20010=ORIENTED_EDGE('',*,*,#14461,.F.);
#20011=ORIENTED_EDGE('',*,*,#14462,.F.);
#20012=ORIENTED_EDGE('',*,*,#14463,.F.);
#20013=ORIENTED_EDGE('',*,*,#14460,.F.);
#20014=ORIENTED_EDGE('',*,*,#14456,.F.);
#20015=ORIENTED_EDGE('',*,*,#14464,.F.);
#20016=ORIENTED_EDGE('',*,*,#14465,.T.);
#20017=ORIENTED_EDGE('',*,*,#14466,.T.);
#20018=ORIENTED_EDGE('',*,*,#14467,.F.);
#20019=ORIENTED_EDGE('',*,*,#14466,.F.);
#20020=ORIENTED_EDGE('',*,*,#14468,.T.);
#20021=ORIENTED_EDGE('',*,*,#14469,.F.);
#20022=ORIENTED_EDGE('',*,*,#14470,.F.);
#20023=ORIENTED_EDGE('',*,*,#14471,.F.);
#20024=ORIENTED_EDGE('',*,*,#14468,.F.);
#20025=ORIENTED_EDGE('',*,*,#14465,.F.);
#20026=ORIENTED_EDGE('',*,*,#14472,.F.);
#20027=ORIENTED_EDGE('',*,*,#14473,.T.);
#20028=ORIENTED_EDGE('',*,*,#14474,.T.);
#20029=ORIENTED_EDGE('',*,*,#14475,.F.);
#20030=ORIENTED_EDGE('',*,*,#14474,.F.);
#20031=ORIENTED_EDGE('',*,*,#14476,.T.);
#20032=ORIENTED_EDGE('',*,*,#14477,.F.);
#20033=ORIENTED_EDGE('',*,*,#14478,.F.);
#20034=ORIENTED_EDGE('',*,*,#14479,.F.);
#20035=ORIENTED_EDGE('',*,*,#14476,.F.);
#20036=ORIENTED_EDGE('',*,*,#14473,.F.);
#20037=ORIENTED_EDGE('',*,*,#14480,.F.);
#20038=ORIENTED_EDGE('',*,*,#14481,.T.);
#20039=ORIENTED_EDGE('',*,*,#14482,.T.);
#20040=ORIENTED_EDGE('',*,*,#14483,.F.);
#20041=ORIENTED_EDGE('',*,*,#14482,.F.);
#20042=ORIENTED_EDGE('',*,*,#14484,.T.);
#20043=ORIENTED_EDGE('',*,*,#14485,.F.);
#20044=ORIENTED_EDGE('',*,*,#14486,.F.);
#20045=ORIENTED_EDGE('',*,*,#14487,.F.);
#20046=ORIENTED_EDGE('',*,*,#14484,.F.);
#20047=ORIENTED_EDGE('',*,*,#14481,.F.);
#20048=ORIENTED_EDGE('',*,*,#14488,.F.);
#20049=ORIENTED_EDGE('',*,*,#14489,.T.);
#20050=ORIENTED_EDGE('',*,*,#14490,.T.);
#20051=ORIENTED_EDGE('',*,*,#14491,.F.);
#20052=ORIENTED_EDGE('',*,*,#14490,.F.);
#20053=ORIENTED_EDGE('',*,*,#14492,.T.);
#20054=ORIENTED_EDGE('',*,*,#14493,.F.);
#20055=ORIENTED_EDGE('',*,*,#14494,.F.);
#20056=ORIENTED_EDGE('',*,*,#14495,.F.);
#20057=ORIENTED_EDGE('',*,*,#14492,.F.);
#20058=ORIENTED_EDGE('',*,*,#14489,.F.);
#20059=ORIENTED_EDGE('',*,*,#14496,.F.);
#20060=ORIENTED_EDGE('',*,*,#14497,.T.);
#20061=ORIENTED_EDGE('',*,*,#14498,.T.);
#20062=ORIENTED_EDGE('',*,*,#14499,.F.);
#20063=ORIENTED_EDGE('',*,*,#14498,.F.);
#20064=ORIENTED_EDGE('',*,*,#14500,.T.);
#20065=ORIENTED_EDGE('',*,*,#14501,.F.);
#20066=ORIENTED_EDGE('',*,*,#14502,.F.);
#20067=ORIENTED_EDGE('',*,*,#14503,.F.);
#20068=ORIENTED_EDGE('',*,*,#14500,.F.);
#20069=ORIENTED_EDGE('',*,*,#14497,.F.);
#20070=ORIENTED_EDGE('',*,*,#14504,.F.);
#20071=ORIENTED_EDGE('',*,*,#14505,.T.);
#20072=ORIENTED_EDGE('',*,*,#14506,.T.);
#20073=ORIENTED_EDGE('',*,*,#14507,.F.);
#20074=ORIENTED_EDGE('',*,*,#14506,.F.);
#20075=ORIENTED_EDGE('',*,*,#14508,.T.);
#20076=ORIENTED_EDGE('',*,*,#14509,.F.);
#20077=ORIENTED_EDGE('',*,*,#14510,.F.);
#20078=ORIENTED_EDGE('',*,*,#14511,.F.);
#20079=ORIENTED_EDGE('',*,*,#14508,.F.);
#20080=ORIENTED_EDGE('',*,*,#14505,.F.);
#20081=ORIENTED_EDGE('',*,*,#14512,.F.);
#20082=ORIENTED_EDGE('',*,*,#14513,.T.);
#20083=ORIENTED_EDGE('',*,*,#14514,.T.);
#20084=ORIENTED_EDGE('',*,*,#14515,.F.);
#20085=ORIENTED_EDGE('',*,*,#14514,.F.);
#20086=ORIENTED_EDGE('',*,*,#14516,.T.);
#20087=ORIENTED_EDGE('',*,*,#14517,.F.);
#20088=ORIENTED_EDGE('',*,*,#14518,.F.);
#20089=ORIENTED_EDGE('',*,*,#14519,.F.);
#20090=ORIENTED_EDGE('',*,*,#14516,.F.);
#20091=ORIENTED_EDGE('',*,*,#14513,.F.);
#20092=ORIENTED_EDGE('',*,*,#14520,.F.);
#20093=ORIENTED_EDGE('',*,*,#14521,.T.);
#20094=ORIENTED_EDGE('',*,*,#14522,.T.);
#20095=ORIENTED_EDGE('',*,*,#14523,.F.);
#20096=ORIENTED_EDGE('',*,*,#14522,.F.);
#20097=ORIENTED_EDGE('',*,*,#14524,.T.);
#20098=ORIENTED_EDGE('',*,*,#14525,.F.);
#20099=ORIENTED_EDGE('',*,*,#14526,.F.);
#20100=ORIENTED_EDGE('',*,*,#14527,.F.);
#20101=ORIENTED_EDGE('',*,*,#14524,.F.);
#20102=ORIENTED_EDGE('',*,*,#14521,.F.);
#20103=ORIENTED_EDGE('',*,*,#14528,.F.);
#20104=ORIENTED_EDGE('',*,*,#14529,.T.);
#20105=ORIENTED_EDGE('',*,*,#14530,.T.);
#20106=ORIENTED_EDGE('',*,*,#14531,.F.);
#20107=ORIENTED_EDGE('',*,*,#14530,.F.);
#20108=ORIENTED_EDGE('',*,*,#14532,.T.);
#20109=ORIENTED_EDGE('',*,*,#14533,.F.);
#20110=ORIENTED_EDGE('',*,*,#14534,.F.);
#20111=ORIENTED_EDGE('',*,*,#14535,.F.);
#20112=ORIENTED_EDGE('',*,*,#14532,.F.);
#20113=ORIENTED_EDGE('',*,*,#14529,.F.);
#20114=ORIENTED_EDGE('',*,*,#14536,.F.);
#20115=ORIENTED_EDGE('',*,*,#14537,.T.);
#20116=ORIENTED_EDGE('',*,*,#14538,.T.);
#20117=ORIENTED_EDGE('',*,*,#14539,.F.);
#20118=ORIENTED_EDGE('',*,*,#14538,.F.);
#20119=ORIENTED_EDGE('',*,*,#14540,.T.);
#20120=ORIENTED_EDGE('',*,*,#14541,.F.);
#20121=ORIENTED_EDGE('',*,*,#14542,.F.);
#20122=ORIENTED_EDGE('',*,*,#14543,.F.);
#20123=ORIENTED_EDGE('',*,*,#14540,.F.);
#20124=ORIENTED_EDGE('',*,*,#14537,.F.);
#20125=ORIENTED_EDGE('',*,*,#14544,.F.);
#20126=ORIENTED_EDGE('',*,*,#14545,.T.);
#20127=ORIENTED_EDGE('',*,*,#14546,.T.);
#20128=ORIENTED_EDGE('',*,*,#14547,.F.);
#20129=ORIENTED_EDGE('',*,*,#14546,.F.);
#20130=ORIENTED_EDGE('',*,*,#14548,.T.);
#20131=ORIENTED_EDGE('',*,*,#14549,.F.);
#20132=ORIENTED_EDGE('',*,*,#14550,.F.);
#20133=ORIENTED_EDGE('',*,*,#14551,.F.);
#20134=ORIENTED_EDGE('',*,*,#14548,.F.);
#20135=ORIENTED_EDGE('',*,*,#14545,.F.);
#20136=ORIENTED_EDGE('',*,*,#14552,.F.);
#20137=ORIENTED_EDGE('',*,*,#14553,.T.);
#20138=ORIENTED_EDGE('',*,*,#14554,.T.);
#20139=ORIENTED_EDGE('',*,*,#14555,.F.);
#20140=ORIENTED_EDGE('',*,*,#14554,.F.);
#20141=ORIENTED_EDGE('',*,*,#14556,.T.);
#20142=ORIENTED_EDGE('',*,*,#14557,.F.);
#20143=ORIENTED_EDGE('',*,*,#14558,.F.);
#20144=ORIENTED_EDGE('',*,*,#14559,.F.);
#20145=ORIENTED_EDGE('',*,*,#14556,.F.);
#20146=ORIENTED_EDGE('',*,*,#14553,.F.);
#20147=ORIENTED_EDGE('',*,*,#14560,.F.);
#20148=ORIENTED_EDGE('',*,*,#14561,.T.);
#20149=ORIENTED_EDGE('',*,*,#14562,.T.);
#20150=ORIENTED_EDGE('',*,*,#14563,.F.);
#20151=ORIENTED_EDGE('',*,*,#14562,.F.);
#20152=ORIENTED_EDGE('',*,*,#14564,.T.);
#20153=ORIENTED_EDGE('',*,*,#14565,.F.);
#20154=ORIENTED_EDGE('',*,*,#14566,.F.);
#20155=ORIENTED_EDGE('',*,*,#14567,.F.);
#20156=ORIENTED_EDGE('',*,*,#14564,.F.);
#20157=ORIENTED_EDGE('',*,*,#14561,.F.);
#20158=ORIENTED_EDGE('',*,*,#14568,.F.);
#20159=ORIENTED_EDGE('',*,*,#14569,.T.);
#20160=ORIENTED_EDGE('',*,*,#14570,.T.);
#20161=ORIENTED_EDGE('',*,*,#14571,.F.);
#20162=ORIENTED_EDGE('',*,*,#14570,.F.);
#20163=ORIENTED_EDGE('',*,*,#14572,.T.);
#20164=ORIENTED_EDGE('',*,*,#14573,.F.);
#20165=ORIENTED_EDGE('',*,*,#14574,.F.);
#20166=ORIENTED_EDGE('',*,*,#14575,.F.);
#20167=ORIENTED_EDGE('',*,*,#14572,.F.);
#20168=ORIENTED_EDGE('',*,*,#14569,.F.);
#20169=ORIENTED_EDGE('',*,*,#14576,.F.);
#20170=ORIENTED_EDGE('',*,*,#14577,.T.);
#20171=ORIENTED_EDGE('',*,*,#14578,.T.);
#20172=ORIENTED_EDGE('',*,*,#14579,.F.);
#20173=ORIENTED_EDGE('',*,*,#14578,.F.);
#20174=ORIENTED_EDGE('',*,*,#14580,.T.);
#20175=ORIENTED_EDGE('',*,*,#14581,.F.);
#20176=ORIENTED_EDGE('',*,*,#14582,.F.);
#20177=ORIENTED_EDGE('',*,*,#14583,.F.);
#20178=ORIENTED_EDGE('',*,*,#14580,.F.);
#20179=ORIENTED_EDGE('',*,*,#14577,.F.);
#20180=ORIENTED_EDGE('',*,*,#14584,.F.);
#20181=ORIENTED_EDGE('',*,*,#14585,.T.);
#20182=ORIENTED_EDGE('',*,*,#14586,.T.);
#20183=ORIENTED_EDGE('',*,*,#14587,.F.);
#20184=ORIENTED_EDGE('',*,*,#14586,.F.);
#20185=ORIENTED_EDGE('',*,*,#14588,.T.);
#20186=ORIENTED_EDGE('',*,*,#14589,.F.);
#20187=ORIENTED_EDGE('',*,*,#14590,.F.);
#20188=ORIENTED_EDGE('',*,*,#14591,.F.);
#20189=ORIENTED_EDGE('',*,*,#14588,.F.);
#20190=ORIENTED_EDGE('',*,*,#14585,.F.);
#20191=ORIENTED_EDGE('',*,*,#14592,.F.);
#20192=ORIENTED_EDGE('',*,*,#14593,.T.);
#20193=ORIENTED_EDGE('',*,*,#14594,.T.);
#20194=ORIENTED_EDGE('',*,*,#14595,.F.);
#20195=ORIENTED_EDGE('',*,*,#14594,.F.);
#20196=ORIENTED_EDGE('',*,*,#14596,.T.);
#20197=ORIENTED_EDGE('',*,*,#14597,.F.);
#20198=ORIENTED_EDGE('',*,*,#14598,.F.);
#20199=ORIENTED_EDGE('',*,*,#14599,.F.);
#20200=ORIENTED_EDGE('',*,*,#14596,.F.);
#20201=ORIENTED_EDGE('',*,*,#14593,.F.);
#20202=ORIENTED_EDGE('',*,*,#14325,.T.);
#20203=ORIENTED_EDGE('',*,*,#14319,.T.);
#20204=ORIENTED_EDGE('',*,*,#14322,.T.);
#20205=ORIENTED_EDGE('',*,*,#14600,.F.);
#20206=ORIENTED_EDGE('',*,*,#14333,.T.);
#20207=ORIENTED_EDGE('',*,*,#14327,.T.);
#20208=ORIENTED_EDGE('',*,*,#14330,.T.);
#20209=ORIENTED_EDGE('',*,*,#14601,.F.);
#20210=ORIENTED_EDGE('',*,*,#14341,.T.);
#20211=ORIENTED_EDGE('',*,*,#14335,.T.);
#20212=ORIENTED_EDGE('',*,*,#14338,.T.);
#20213=ORIENTED_EDGE('',*,*,#14602,.F.);
#20214=ORIENTED_EDGE('',*,*,#14349,.T.);
#20215=ORIENTED_EDGE('',*,*,#14343,.T.);
#20216=ORIENTED_EDGE('',*,*,#14346,.T.);
#20217=ORIENTED_EDGE('',*,*,#14603,.F.);
#20218=ORIENTED_EDGE('',*,*,#14357,.T.);
#20219=ORIENTED_EDGE('',*,*,#14351,.T.);
#20220=ORIENTED_EDGE('',*,*,#14354,.T.);
#20221=ORIENTED_EDGE('',*,*,#14604,.F.);
#20222=ORIENTED_EDGE('',*,*,#14365,.T.);
#20223=ORIENTED_EDGE('',*,*,#14359,.T.);
#20224=ORIENTED_EDGE('',*,*,#14362,.T.);
#20225=ORIENTED_EDGE('',*,*,#14605,.F.);
#20226=ORIENTED_EDGE('',*,*,#14373,.T.);
#20227=ORIENTED_EDGE('',*,*,#14367,.T.);
#20228=ORIENTED_EDGE('',*,*,#14370,.T.);
#20229=ORIENTED_EDGE('',*,*,#14606,.F.);
#20230=ORIENTED_EDGE('',*,*,#14381,.T.);
#20231=ORIENTED_EDGE('',*,*,#14375,.T.);
#20232=ORIENTED_EDGE('',*,*,#14378,.T.);
#20233=ORIENTED_EDGE('',*,*,#14607,.F.);
#20234=ORIENTED_EDGE('',*,*,#14389,.T.);
#20235=ORIENTED_EDGE('',*,*,#14383,.T.);
#20236=ORIENTED_EDGE('',*,*,#14386,.T.);
#20237=ORIENTED_EDGE('',*,*,#14608,.F.);
#20238=ORIENTED_EDGE('',*,*,#14397,.T.);
#20239=ORIENTED_EDGE('',*,*,#14391,.T.);
#20240=ORIENTED_EDGE('',*,*,#14394,.T.);
#20241=ORIENTED_EDGE('',*,*,#14609,.F.);
#20242=ORIENTED_EDGE('',*,*,#14405,.T.);
#20243=ORIENTED_EDGE('',*,*,#14399,.T.);
#20244=ORIENTED_EDGE('',*,*,#14402,.T.);
#20245=ORIENTED_EDGE('',*,*,#14610,.F.);
#20246=ORIENTED_EDGE('',*,*,#14413,.T.);
#20247=ORIENTED_EDGE('',*,*,#14407,.T.);
#20248=ORIENTED_EDGE('',*,*,#14410,.T.);
#20249=ORIENTED_EDGE('',*,*,#14611,.F.);
#20250=ORIENTED_EDGE('',*,*,#14421,.T.);
#20251=ORIENTED_EDGE('',*,*,#14415,.T.);
#20252=ORIENTED_EDGE('',*,*,#14418,.T.);
#20253=ORIENTED_EDGE('',*,*,#14612,.F.);
#20254=ORIENTED_EDGE('',*,*,#14429,.T.);
#20255=ORIENTED_EDGE('',*,*,#14423,.T.);
#20256=ORIENTED_EDGE('',*,*,#14426,.T.);
#20257=ORIENTED_EDGE('',*,*,#14613,.F.);
#20258=ORIENTED_EDGE('',*,*,#14437,.T.);
#20259=ORIENTED_EDGE('',*,*,#14431,.T.);
#20260=ORIENTED_EDGE('',*,*,#14434,.T.);
#20261=ORIENTED_EDGE('',*,*,#14614,.F.);
#20262=ORIENTED_EDGE('',*,*,#14445,.T.);
#20263=ORIENTED_EDGE('',*,*,#14439,.T.);
#20264=ORIENTED_EDGE('',*,*,#14442,.T.);
#20265=ORIENTED_EDGE('',*,*,#14615,.F.);
#20266=ORIENTED_EDGE('',*,*,#14453,.T.);
#20267=ORIENTED_EDGE('',*,*,#14447,.T.);
#20268=ORIENTED_EDGE('',*,*,#14450,.T.);
#20269=ORIENTED_EDGE('',*,*,#14616,.F.);
#20270=ORIENTED_EDGE('',*,*,#14462,.T.);
#20271=ORIENTED_EDGE('',*,*,#14455,.T.);
#20272=ORIENTED_EDGE('',*,*,#14617,.T.);
#20273=ORIENTED_EDGE('',*,*,#14618,.T.);
#20274=ORIENTED_EDGE('',*,*,#14617,.F.);
#20275=ORIENTED_EDGE('',*,*,#14458,.T.);
#20276=ORIENTED_EDGE('',*,*,#14459,.T.);
#20277=ORIENTED_EDGE('',*,*,#14619,.F.);
#20278=ORIENTED_EDGE('',*,*,#14470,.T.);
#20279=ORIENTED_EDGE('',*,*,#14464,.T.);
#20280=ORIENTED_EDGE('',*,*,#14467,.T.);
#20281=ORIENTED_EDGE('',*,*,#14620,.F.);
#20282=ORIENTED_EDGE('',*,*,#14478,.T.);
#20283=ORIENTED_EDGE('',*,*,#14472,.T.);
#20284=ORIENTED_EDGE('',*,*,#14475,.T.);
#20285=ORIENTED_EDGE('',*,*,#14621,.F.);
#20286=ORIENTED_EDGE('',*,*,#14486,.T.);
#20287=ORIENTED_EDGE('',*,*,#14480,.T.);
#20288=ORIENTED_EDGE('',*,*,#14483,.T.);
#20289=ORIENTED_EDGE('',*,*,#14622,.F.);
#20290=ORIENTED_EDGE('',*,*,#14494,.T.);
#20291=ORIENTED_EDGE('',*,*,#14488,.T.);
#20292=ORIENTED_EDGE('',*,*,#14491,.T.);
#20293=ORIENTED_EDGE('',*,*,#14623,.F.);
#20294=ORIENTED_EDGE('',*,*,#14502,.T.);
#20295=ORIENTED_EDGE('',*,*,#14496,.T.);
#20296=ORIENTED_EDGE('',*,*,#14499,.T.);
#20297=ORIENTED_EDGE('',*,*,#14624,.F.);
#20298=ORIENTED_EDGE('',*,*,#14510,.T.);
#20299=ORIENTED_EDGE('',*,*,#14504,.T.);
#20300=ORIENTED_EDGE('',*,*,#14507,.T.);
#20301=ORIENTED_EDGE('',*,*,#14625,.F.);
#20302=ORIENTED_EDGE('',*,*,#14518,.T.);
#20303=ORIENTED_EDGE('',*,*,#14512,.T.);
#20304=ORIENTED_EDGE('',*,*,#14515,.T.);
#20305=ORIENTED_EDGE('',*,*,#14626,.F.);
#20306=ORIENTED_EDGE('',*,*,#14526,.T.);
#20307=ORIENTED_EDGE('',*,*,#14520,.T.);
#20308=ORIENTED_EDGE('',*,*,#14523,.T.);
#20309=ORIENTED_EDGE('',*,*,#14627,.F.);
#20310=ORIENTED_EDGE('',*,*,#14534,.T.);
#20311=ORIENTED_EDGE('',*,*,#14528,.T.);
#20312=ORIENTED_EDGE('',*,*,#14531,.T.);
#20313=ORIENTED_EDGE('',*,*,#14628,.F.);
#20314=ORIENTED_EDGE('',*,*,#14542,.T.);
#20315=ORIENTED_EDGE('',*,*,#14536,.T.);
#20316=ORIENTED_EDGE('',*,*,#14539,.T.);
#20317=ORIENTED_EDGE('',*,*,#14629,.F.);
#20318=ORIENTED_EDGE('',*,*,#14550,.T.);
#20319=ORIENTED_EDGE('',*,*,#14544,.T.);
#20320=ORIENTED_EDGE('',*,*,#14547,.T.);
#20321=ORIENTED_EDGE('',*,*,#14630,.F.);
#20322=ORIENTED_EDGE('',*,*,#14558,.T.);
#20323=ORIENTED_EDGE('',*,*,#14552,.T.);
#20324=ORIENTED_EDGE('',*,*,#14555,.T.);
#20325=ORIENTED_EDGE('',*,*,#14631,.F.);
#20326=ORIENTED_EDGE('',*,*,#14566,.T.);
#20327=ORIENTED_EDGE('',*,*,#14560,.T.);
#20328=ORIENTED_EDGE('',*,*,#14563,.T.);
#20329=ORIENTED_EDGE('',*,*,#14632,.F.);
#20330=ORIENTED_EDGE('',*,*,#14574,.T.);
#20331=ORIENTED_EDGE('',*,*,#14568,.T.);
#20332=ORIENTED_EDGE('',*,*,#14571,.T.);
#20333=ORIENTED_EDGE('',*,*,#14633,.F.);
#20334=ORIENTED_EDGE('',*,*,#14582,.T.);
#20335=ORIENTED_EDGE('',*,*,#14576,.T.);
#20336=ORIENTED_EDGE('',*,*,#14579,.T.);
#20337=ORIENTED_EDGE('',*,*,#14634,.F.);
#20338=ORIENTED_EDGE('',*,*,#14590,.T.);
#20339=ORIENTED_EDGE('',*,*,#14584,.T.);
#20340=ORIENTED_EDGE('',*,*,#14587,.T.);
#20341=ORIENTED_EDGE('',*,*,#14635,.F.);
#20342=ORIENTED_EDGE('',*,*,#14598,.T.);
#20343=ORIENTED_EDGE('',*,*,#14592,.T.);
#20344=ORIENTED_EDGE('',*,*,#14595,.T.);
#20345=ORIENTED_EDGE('',*,*,#14636,.F.);
#20346=ORIENTED_EDGE('',*,*,#14637,.T.);
#20347=ORIENTED_EDGE('',*,*,#14638,.T.);
#20348=ORIENTED_EDGE('',*,*,#14639,.T.);
#20349=ORIENTED_EDGE('',*,*,#14640,.F.);
#20350=ORIENTED_EDGE('',*,*,#14639,.F.);
#20351=ORIENTED_EDGE('',*,*,#14641,.F.);
#20352=ORIENTED_EDGE('',*,*,#14642,.T.);
#20353=ORIENTED_EDGE('',*,*,#14643,.F.);
#20354=ORIENTED_EDGE('',*,*,#14644,.F.);
#20355=ORIENTED_EDGE('',*,*,#14642,.F.);
#20356=ORIENTED_EDGE('',*,*,#14645,.F.);
#20357=ORIENTED_EDGE('',*,*,#14637,.F.);
#20358=ORIENTED_EDGE('',*,*,#14638,.F.);
#20359=ORIENTED_EDGE('',*,*,#14645,.T.);
#20360=ORIENTED_EDGE('',*,*,#14641,.T.);
#20361=ORIENTED_EDGE('',*,*,#14646,.F.);
#20362=ORIENTED_EDGE('',*,*,#14647,.T.);
#20363=ORIENTED_EDGE('',*,*,#14463,.T.);
#20364=ORIENTED_EDGE('',*,*,#14616,.T.);
#20365=ORIENTED_EDGE('',*,*,#14452,.T.);
#20366=ORIENTED_EDGE('',*,*,#14454,.T.);
#20367=ORIENTED_EDGE('',*,*,#14615,.T.);
#20368=ORIENTED_EDGE('',*,*,#14444,.T.);
#20369=ORIENTED_EDGE('',*,*,#14446,.T.);
#20370=ORIENTED_EDGE('',*,*,#14614,.T.);
#20371=ORIENTED_EDGE('',*,*,#14436,.T.);
#20372=ORIENTED_EDGE('',*,*,#14438,.T.);
#20373=ORIENTED_EDGE('',*,*,#14613,.T.);
#20374=ORIENTED_EDGE('',*,*,#14428,.T.);
#20375=ORIENTED_EDGE('',*,*,#14430,.T.);
#20376=ORIENTED_EDGE('',*,*,#14612,.T.);
#20377=ORIENTED_EDGE('',*,*,#14420,.T.);
#20378=ORIENTED_EDGE('',*,*,#14422,.T.);
#20379=ORIENTED_EDGE('',*,*,#14611,.T.);
#20380=ORIENTED_EDGE('',*,*,#14412,.T.);
#20381=ORIENTED_EDGE('',*,*,#14414,.T.);
#20382=ORIENTED_EDGE('',*,*,#14610,.T.);
#20383=ORIENTED_EDGE('',*,*,#14404,.T.);
#20384=ORIENTED_EDGE('',*,*,#14406,.T.);
#20385=ORIENTED_EDGE('',*,*,#14609,.T.);
#20386=ORIENTED_EDGE('',*,*,#14396,.T.);
#20387=ORIENTED_EDGE('',*,*,#14398,.T.);
#20388=ORIENTED_EDGE('',*,*,#14608,.T.);
#20389=ORIENTED_EDGE('',*,*,#14388,.T.);
#20390=ORIENTED_EDGE('',*,*,#14390,.T.);
#20391=ORIENTED_EDGE('',*,*,#14607,.T.);
#20392=ORIENTED_EDGE('',*,*,#14380,.T.);
#20393=ORIENTED_EDGE('',*,*,#14382,.T.);
#20394=ORIENTED_EDGE('',*,*,#14606,.T.);
#20395=ORIENTED_EDGE('',*,*,#14372,.T.);
#20396=ORIENTED_EDGE('',*,*,#14374,.T.);
#20397=ORIENTED_EDGE('',*,*,#14605,.T.);
#20398=ORIENTED_EDGE('',*,*,#14364,.T.);
#20399=ORIENTED_EDGE('',*,*,#14366,.T.);
#20400=ORIENTED_EDGE('',*,*,#14604,.T.);
#20401=ORIENTED_EDGE('',*,*,#14356,.T.);
#20402=ORIENTED_EDGE('',*,*,#14358,.T.);
#20403=ORIENTED_EDGE('',*,*,#14603,.T.);
#20404=ORIENTED_EDGE('',*,*,#14348,.T.);
#20405=ORIENTED_EDGE('',*,*,#14350,.T.);
#20406=ORIENTED_EDGE('',*,*,#14602,.T.);
#20407=ORIENTED_EDGE('',*,*,#14340,.T.);
#20408=ORIENTED_EDGE('',*,*,#14342,.T.);
#20409=ORIENTED_EDGE('',*,*,#14601,.T.);
#20410=ORIENTED_EDGE('',*,*,#14332,.T.);
#20411=ORIENTED_EDGE('',*,*,#14334,.T.);
#20412=ORIENTED_EDGE('',*,*,#14600,.T.);
#20413=ORIENTED_EDGE('',*,*,#14324,.T.);
#20414=ORIENTED_EDGE('',*,*,#14326,.T.);
#20415=ORIENTED_EDGE('',*,*,#14640,.T.);
#20416=ORIENTED_EDGE('',*,*,#14643,.T.);
#20417=ORIENTED_EDGE('',*,*,#14644,.T.);
#20418=ORIENTED_EDGE('',*,*,#14636,.T.);
#20419=ORIENTED_EDGE('',*,*,#14597,.T.);
#20420=ORIENTED_EDGE('',*,*,#14599,.T.);
#20421=ORIENTED_EDGE('',*,*,#14635,.T.);
#20422=ORIENTED_EDGE('',*,*,#14589,.T.);
#20423=ORIENTED_EDGE('',*,*,#14591,.T.);
#20424=ORIENTED_EDGE('',*,*,#14634,.T.);
#20425=ORIENTED_EDGE('',*,*,#14581,.T.);
#20426=ORIENTED_EDGE('',*,*,#14583,.T.);
#20427=ORIENTED_EDGE('',*,*,#14633,.T.);
#20428=ORIENTED_EDGE('',*,*,#14573,.T.);
#20429=ORIENTED_EDGE('',*,*,#14575,.T.);
#20430=ORIENTED_EDGE('',*,*,#14632,.T.);
#20431=ORIENTED_EDGE('',*,*,#14565,.T.);
#20432=ORIENTED_EDGE('',*,*,#14567,.T.);
#20433=ORIENTED_EDGE('',*,*,#14631,.T.);
#20434=ORIENTED_EDGE('',*,*,#14557,.T.);
#20435=ORIENTED_EDGE('',*,*,#14559,.T.);
#20436=ORIENTED_EDGE('',*,*,#14630,.T.);
#20437=ORIENTED_EDGE('',*,*,#14549,.T.);
#20438=ORIENTED_EDGE('',*,*,#14551,.T.);
#20439=ORIENTED_EDGE('',*,*,#14629,.T.);
#20440=ORIENTED_EDGE('',*,*,#14541,.T.);
#20441=ORIENTED_EDGE('',*,*,#14543,.T.);
#20442=ORIENTED_EDGE('',*,*,#14628,.T.);
#20443=ORIENTED_EDGE('',*,*,#14533,.T.);
#20444=ORIENTED_EDGE('',*,*,#14535,.T.);
#20445=ORIENTED_EDGE('',*,*,#14627,.T.);
#20446=ORIENTED_EDGE('',*,*,#14525,.T.);
#20447=ORIENTED_EDGE('',*,*,#14527,.T.);
#20448=ORIENTED_EDGE('',*,*,#14626,.T.);
#20449=ORIENTED_EDGE('',*,*,#14517,.T.);
#20450=ORIENTED_EDGE('',*,*,#14519,.T.);
#20451=ORIENTED_EDGE('',*,*,#14625,.T.);
#20452=ORIENTED_EDGE('',*,*,#14509,.T.);
#20453=ORIENTED_EDGE('',*,*,#14511,.T.);
#20454=ORIENTED_EDGE('',*,*,#14624,.T.);
#20455=ORIENTED_EDGE('',*,*,#14501,.T.);
#20456=ORIENTED_EDGE('',*,*,#14503,.T.);
#20457=ORIENTED_EDGE('',*,*,#14623,.T.);
#20458=ORIENTED_EDGE('',*,*,#14493,.T.);
#20459=ORIENTED_EDGE('',*,*,#14495,.T.);
#20460=ORIENTED_EDGE('',*,*,#14622,.T.);
#20461=ORIENTED_EDGE('',*,*,#14485,.T.);
#20462=ORIENTED_EDGE('',*,*,#14487,.T.);
#20463=ORIENTED_EDGE('',*,*,#14621,.T.);
#20464=ORIENTED_EDGE('',*,*,#14477,.T.);
#20465=ORIENTED_EDGE('',*,*,#14479,.T.);
#20466=ORIENTED_EDGE('',*,*,#14620,.T.);
#20467=ORIENTED_EDGE('',*,*,#14469,.T.);
#20468=ORIENTED_EDGE('',*,*,#14471,.T.);
#20469=ORIENTED_EDGE('',*,*,#14619,.T.);
#20470=ORIENTED_EDGE('',*,*,#14461,.T.);
#20471=ORIENTED_EDGE('',*,*,#14647,.F.);
#20472=ORIENTED_EDGE('',*,*,#14648,.T.);
#20473=ORIENTED_EDGE('',*,*,#14649,.F.);
#20474=ORIENTED_EDGE('',*,*,#14648,.F.);
#20475=ORIENTED_EDGE('',*,*,#14650,.F.);
#20476=ORIENTED_EDGE('',*,*,#14651,.T.);
#20477=ORIENTED_EDGE('',*,*,#14652,.T.);
#20478=ORIENTED_EDGE('',*,*,#14653,.F.);
#20479=ORIENTED_EDGE('',*,*,#14654,.F.);
#20480=ORIENTED_EDGE('',*,*,#14655,.T.);
#20481=ORIENTED_EDGE('',*,*,#14656,.T.);
#20482=ORIENTED_EDGE('',*,*,#14651,.F.);
#20483=ORIENTED_EDGE('',*,*,#14657,.F.);
#20484=ORIENTED_EDGE('',*,*,#14658,.T.);
#20485=ORIENTED_EDGE('',*,*,#14659,.T.);
#20486=ORIENTED_EDGE('',*,*,#14655,.F.);
#20487=ORIENTED_EDGE('',*,*,#14660,.F.);
#20488=ORIENTED_EDGE('',*,*,#14661,.T.);
#20489=ORIENTED_EDGE('',*,*,#14662,.T.);
#20490=ORIENTED_EDGE('',*,*,#14658,.F.);
#20491=ORIENTED_EDGE('',*,*,#14663,.F.);
#20492=ORIENTED_EDGE('',*,*,#14664,.T.);
#20493=ORIENTED_EDGE('',*,*,#14665,.T.);
#20494=ORIENTED_EDGE('',*,*,#14661,.F.);
#20495=ORIENTED_EDGE('',*,*,#14666,.F.);
#20496=ORIENTED_EDGE('',*,*,#14653,.T.);
#20497=ORIENTED_EDGE('',*,*,#14667,.T.);
#20498=ORIENTED_EDGE('',*,*,#14664,.F.);
#20499=ORIENTED_EDGE('',*,*,#14667,.F.);
#20500=ORIENTED_EDGE('',*,*,#14652,.F.);
#20501=ORIENTED_EDGE('',*,*,#14656,.F.);
#20502=ORIENTED_EDGE('',*,*,#14659,.F.);
#20503=ORIENTED_EDGE('',*,*,#14662,.F.);
#20504=ORIENTED_EDGE('',*,*,#14665,.F.);
#20505=ORIENTED_EDGE('',*,*,#14649,.T.);
#20506=ORIENTED_EDGE('',*,*,#14668,.F.);
#20507=ORIENTED_EDGE('',*,*,#14136,.F.);
#20508=ORIENTED_EDGE('',*,*,#14669,.T.);
#20509=ORIENTED_EDGE('',*,*,#14668,.T.);
#20510=ORIENTED_EDGE('',*,*,#14669,.F.);
#20511=ORIENTED_EDGE('',*,*,#14217,.T.);
#20512=ORIENTED_EDGE('',*,*,#14313,.T.);
#20513=ORIENTED_EDGE('',*,*,#14670,.F.);
#20514=ORIENTED_EDGE('',*,*,#14318,.T.);
#20515=ORIENTED_EDGE('',*,*,#14671,.F.);
#20516=ORIENTED_EDGE('',*,*,#14672,.T.);
#20517=ORIENTED_EDGE('',*,*,#14310,.T.);
#20518=ORIENTED_EDGE('',*,*,#14670,.T.);
#20519=ORIENTED_EDGE('',*,*,#14311,.T.);
#20520=ORIENTED_EDGE('',*,*,#14672,.F.);
#20521=ORIENTED_EDGE('',*,*,#14618,.F.);
#20522=ORIENTED_EDGE('',*,*,#14671,.T.);
#20523=ORIENTED_EDGE('',*,*,#14646,.T.);
#20524=ORIENTED_EDGE('',*,*,#14650,.T.);
#20525=ORIENTED_EDGE('',*,*,#14666,.T.);
#20526=ORIENTED_EDGE('',*,*,#14663,.T.);
#20527=ORIENTED_EDGE('',*,*,#14660,.T.);
#20528=ORIENTED_EDGE('',*,*,#14657,.T.);
#20529=ORIENTED_EDGE('',*,*,#14654,.T.);
#23149=CONICAL_SURFACE('',#26504,0.1825,0.785398163397448);
#23150=CONICAL_SURFACE('',#26506,0.0346410161513776,1.00188494390461);
#23151=CONICAL_SURFACE('',#26517,0.088,0.785398163397448);
#23152=CONICAL_SURFACE('',#26520,0.105,0.785398163397449);
#23918=ADVANCED_FACE('',(#3165),#2221,.T.);
#23919=ADVANCED_FACE('',(#3166),#2222,.T.);
#23920=ADVANCED_FACE('',(#3167),#2223,.T.);
#23921=ADVANCED_FACE('',(#3168),#2224,.T.);
#23922=ADVANCED_FACE('',(#3169),#2225,.T.);
#23923=ADVANCED_FACE('',(#3170),#2226,.T.);
#23924=ADVANCED_FACE('',(#3171),#2227,.T.);
#23925=ADVANCED_FACE('',(#3172),#2228,.T.);
#23926=ADVANCED_FACE('',(#3173),#2229,.T.);
#23927=ADVANCED_FACE('',(#3174),#2230,.T.);
#23928=ADVANCED_FACE('',(#3175),#2231,.T.);
#23929=ADVANCED_FACE('',(#3176),#2232,.T.);
#23930=ADVANCED_FACE('',(#3177),#2233,.T.);
#23931=ADVANCED_FACE('',(#3178),#2234,.T.);
#23932=ADVANCED_FACE('',(#3179),#2235,.T.);
#23933=ADVANCED_FACE('',(#3180),#2236,.T.);
#23934=ADVANCED_FACE('',(#3181),#2237,.T.);
#23935=ADVANCED_FACE('',(#3182),#2238,.T.);
#23936=ADVANCED_FACE('',(#3183),#2239,.T.);
#23937=ADVANCED_FACE('',(#3184),#2240,.T.);
#23938=ADVANCED_FACE('',(#3185),#2241,.T.);
#23939=ADVANCED_FACE('',(#3186),#2242,.T.);
#23940=ADVANCED_FACE('',(#3187),#2243,.T.);
#23941=ADVANCED_FACE('',(#3188),#2244,.T.);
#23942=ADVANCED_FACE('',(#3189),#2245,.T.);
#23943=ADVANCED_FACE('',(#3190),#2246,.T.);
#23944=ADVANCED_FACE('',(#3191),#2247,.T.);
#23945=ADVANCED_FACE('',(#3192),#2248,.T.);
#23946=ADVANCED_FACE('',(#3193),#2249,.T.);
#23947=ADVANCED_FACE('',(#3194),#2250,.T.);
#23948=ADVANCED_FACE('',(#3195),#2251,.T.);
#23949=ADVANCED_FACE('',(#3196),#2252,.T.);
#23950=ADVANCED_FACE('',(#3197),#2253,.T.);
#23951=ADVANCED_FACE('',(#3198),#2254,.T.);
#23952=ADVANCED_FACE('',(#3199),#2255,.T.);
#23953=ADVANCED_FACE('',(#3200),#2256,.T.);
#23954=ADVANCED_FACE('',(#3201),#2257,.T.);
#23955=ADVANCED_FACE('',(#3202),#2258,.T.);
#23956=ADVANCED_FACE('',(#3203),#2259,.T.);
#23957=ADVANCED_FACE('',(#3204),#2260,.T.);
#23958=ADVANCED_FACE('',(#3205),#2261,.T.);
#23959=ADVANCED_FACE('',(#3206),#2262,.T.);
#23960=ADVANCED_FACE('',(#3207),#2263,.T.);
#23961=ADVANCED_FACE('',(#3208),#2264,.T.);
#23962=ADVANCED_FACE('',(#3209),#2265,.T.);
#23963=ADVANCED_FACE('',(#3210),#2266,.T.);
#23964=ADVANCED_FACE('',(#3211),#2267,.T.);
#23965=ADVANCED_FACE('',(#3212),#2268,.T.);
#23966=ADVANCED_FACE('',(#3213),#2269,.T.);
#23967=ADVANCED_FACE('',(#3214),#2270,.T.);
#23968=ADVANCED_FACE('',(#3215),#2271,.T.);
#23969=ADVANCED_FACE('',(#3216),#2272,.T.);
#23970=ADVANCED_FACE('',(#3217),#2273,.T.);
#23971=ADVANCED_FACE('',(#3218),#2274,.T.);
#23972=ADVANCED_FACE('',(#3219),#2275,.T.);
#23973=ADVANCED_FACE('',(#3220),#2276,.T.);
#23974=ADVANCED_FACE('',(#3221),#2277,.T.);
#23975=ADVANCED_FACE('',(#3222),#1558,.F.);
#23976=ADVANCED_FACE('',(#3223),#474,.F.);
#23977=ADVANCED_FACE('',(#3224),#1559,.T.);
#23978=ADVANCED_FACE('',(#3225),#2278,.T.);
#23979=ADVANCED_FACE('',(#3226),#475,.F.);
#23980=ADVANCED_FACE('',(#3227),#1560,.T.);
#23981=ADVANCED_FACE('',(#3228),#1561,.F.);
#23982=ADVANCED_FACE('',(#3229),#1562,.F.);
#23983=ADVANCED_FACE('',(#3230),#1563,.T.);
#23984=ADVANCED_FACE('',(#3231),#1564,.F.);
#23985=ADVANCED_FACE('',(#3232),#1565,.F.);
#23986=ADVANCED_FACE('',(#3233),#1566,.T.);
#23987=ADVANCED_FACE('',(#3234),#1567,.F.);
#23988=ADVANCED_FACE('',(#3235),#1568,.F.);
#23989=ADVANCED_FACE('',(#3236),#1569,.T.);
#23990=ADVANCED_FACE('',(#3237),#1570,.F.);
#23991=ADVANCED_FACE('',(#3238),#1571,.F.);
#23992=ADVANCED_FACE('',(#3239),#1572,.T.);
#23993=ADVANCED_FACE('',(#3240),#1573,.F.);
#23994=ADVANCED_FACE('',(#3241),#1574,.F.);
#23995=ADVANCED_FACE('',(#3242),#1575,.T.);
#23996=ADVANCED_FACE('',(#3243),#1576,.F.);
#23997=ADVANCED_FACE('',(#3244),#1577,.F.);
#23998=ADVANCED_FACE('',(#3245),#1578,.T.);
#23999=ADVANCED_FACE('',(#3246),#1579,.F.);
#24000=ADVANCED_FACE('',(#3247),#1580,.F.);
#24001=ADVANCED_FACE('',(#3248),#1581,.T.);
#24002=ADVANCED_FACE('',(#3249),#1582,.F.);
#24003=ADVANCED_FACE('',(#3250),#1583,.F.);
#24004=ADVANCED_FACE('',(#3251),#1584,.T.);
#24005=ADVANCED_FACE('',(#3252),#1585,.F.);
#24006=ADVANCED_FACE('',(#3253),#1586,.F.);
#24007=ADVANCED_FACE('',(#3254),#1587,.T.);
#24008=ADVANCED_FACE('',(#3255),#1588,.F.);
#24009=ADVANCED_FACE('',(#3256),#1589,.F.);
#24010=ADVANCED_FACE('',(#3257),#1590,.T.);
#24011=ADVANCED_FACE('',(#3258),#1591,.F.);
#24012=ADVANCED_FACE('',(#3259),#1592,.F.);
#24013=ADVANCED_FACE('',(#3260),#1593,.T.);
#24014=ADVANCED_FACE('',(#3261),#1594,.F.);
#24015=ADVANCED_FACE('',(#3262),#1595,.F.);
#24016=ADVANCED_FACE('',(#3263),#1596,.T.);
#24017=ADVANCED_FACE('',(#3264),#1597,.F.);
#24018=ADVANCED_FACE('',(#3265),#1598,.F.);
#24019=ADVANCED_FACE('',(#3266),#1599,.T.);
#24020=ADVANCED_FACE('',(#3267),#1600,.F.);
#24021=ADVANCED_FACE('',(#3268),#1601,.F.);
#24022=ADVANCED_FACE('',(#3269),#1602,.T.);
#24023=ADVANCED_FACE('',(#3270),#1603,.F.);
#24024=ADVANCED_FACE('',(#3271),#1604,.F.);
#24025=ADVANCED_FACE('',(#3272),#1605,.T.);
#24026=ADVANCED_FACE('',(#3273),#1606,.F.);
#24027=ADVANCED_FACE('',(#3274),#1607,.F.);
#24028=ADVANCED_FACE('',(#3275),#1608,.T.);
#24029=ADVANCED_FACE('',(#3276),#1609,.F.);
#24030=ADVANCED_FACE('',(#3277),#1610,.F.);
#24031=ADVANCED_FACE('',(#3278),#1611,.T.);
#24032=ADVANCED_FACE('',(#3279),#1612,.F.);
#24033=ADVANCED_FACE('',(#3280),#1613,.F.);
#24034=ADVANCED_FACE('',(#3281),#1614,.T.);
#24035=ADVANCED_FACE('',(#3282),#1615,.F.);
#24036=ADVANCED_FACE('',(#3283),#1616,.F.);
#24037=ADVANCED_FACE('',(#3284),#1617,.T.);
#24038=ADVANCED_FACE('',(#3285),#1618,.F.);
#24039=ADVANCED_FACE('',(#3286),#1619,.F.);
#24040=ADVANCED_FACE('',(#3287),#1620,.T.);
#24041=ADVANCED_FACE('',(#3288),#1621,.F.);
#24042=ADVANCED_FACE('',(#3289),#1622,.F.);
#24043=ADVANCED_FACE('',(#3290),#1623,.T.);
#24044=ADVANCED_FACE('',(#3291),#1624,.F.);
#24045=ADVANCED_FACE('',(#3292),#1625,.F.);
#24046=ADVANCED_FACE('',(#3293),#1626,.T.);
#24047=ADVANCED_FACE('',(#3294),#1627,.F.);
#24048=ADVANCED_FACE('',(#3295),#1628,.F.);
#24049=ADVANCED_FACE('',(#3296),#1629,.T.);
#24050=ADVANCED_FACE('',(#3297),#1630,.F.);
#24051=ADVANCED_FACE('',(#3298),#1631,.F.);
#24052=ADVANCED_FACE('',(#3299),#1632,.T.);
#24053=ADVANCED_FACE('',(#3300),#1633,.F.);
#24054=ADVANCED_FACE('',(#3301),#1634,.F.);
#24055=ADVANCED_FACE('',(#3302),#1635,.T.);
#24056=ADVANCED_FACE('',(#3303),#1636,.F.);
#24057=ADVANCED_FACE('',(#3304),#1637,.F.);
#24058=ADVANCED_FACE('',(#3305),#1638,.T.);
#24059=ADVANCED_FACE('',(#3306),#1639,.F.);
#24060=ADVANCED_FACE('',(#3307),#1640,.F.);
#24061=ADVANCED_FACE('',(#3308),#1641,.T.);
#24062=ADVANCED_FACE('',(#3309),#1642,.F.);
#24063=ADVANCED_FACE('',(#3310),#1643,.F.);
#24064=ADVANCED_FACE('',(#3311),#1644,.T.);
#24065=ADVANCED_FACE('',(#3312),#1645,.F.);
#24066=ADVANCED_FACE('',(#3313),#1646,.F.);
#24067=ADVANCED_FACE('',(#3314),#1647,.T.);
#24068=ADVANCED_FACE('',(#3315),#1648,.F.);
#24069=ADVANCED_FACE('',(#3316),#1649,.F.);
#24070=ADVANCED_FACE('',(#3317),#1650,.T.);
#24071=ADVANCED_FACE('',(#3318),#1651,.F.);
#24072=ADVANCED_FACE('',(#3319),#1652,.F.);
#24073=ADVANCED_FACE('',(#3320),#1653,.T.);
#24074=ADVANCED_FACE('',(#3321),#1654,.F.);
#24075=ADVANCED_FACE('',(#3322),#1655,.F.);
#24076=ADVANCED_FACE('',(#3323),#1656,.T.);
#24077=ADVANCED_FACE('',(#3324),#1657,.F.);
#24078=ADVANCED_FACE('',(#3325),#1658,.F.);
#24079=ADVANCED_FACE('',(#3326),#1659,.T.);
#24080=ADVANCED_FACE('',(#3327),#1660,.F.);
#24081=ADVANCED_FACE('',(#3328),#1661,.F.);
#24082=ADVANCED_FACE('',(#3329),#1662,.T.);
#24083=ADVANCED_FACE('',(#3330),#1663,.F.);
#24084=ADVANCED_FACE('',(#3331),#1664,.F.);
#24085=ADVANCED_FACE('',(#3332),#2279,.T.);
#24086=ADVANCED_FACE('',(#3333),#1665,.F.);
#24087=ADVANCED_FACE('',(#3334),#1666,.F.);
#24088=ADVANCED_FACE('',(#3335),#1667,.T.);
#24089=ADVANCED_FACE('',(#3336),#23149,.T.);
#24090=ADVANCED_FACE('',(#3337),#23150,.F.);
#24091=ADVANCED_FACE('',(#3338),#1668,.F.);
#24092=ADVANCED_FACE('',(#3339),#1669,.F.);
#24093=ADVANCED_FACE('',(#3340),#1670,.F.);
#24094=ADVANCED_FACE('',(#3341),#1671,.F.);
#24095=ADVANCED_FACE('',(#3342),#1672,.F.);
#24096=ADVANCED_FACE('',(#3343),#1673,.F.);
#24097=ADVANCED_FACE('',(#3344,#1263),#1674,.F.);
#24098=ADVANCED_FACE('',(#3345),#1675,.T.);
#24099=ADVANCED_FACE('',(#3346),#23151,.T.);
#24100=ADVANCED_FACE('',(#3347),#2280,.T.);
#24101=ADVANCED_FACE('',(#3348),#23152,.T.);
#24102=ADVANCED_FACE('',(#3349,#1264),#1676,.T.);
#24103=ADVANCED_FACE('',(#3350,#1265),#1677,.T.);
#24544=CLOSED_SHELL('',(#23918,#23919,#23920,#23921,#23922,#23923,#23924,
#23925,#23926,#23927,#23928,#23929,#23930,#23931,#23932,#23933,#23934,#23935,
#23936,#23937,#23938,#23939,#23940,#23941,#23942,#23943,#23944,#23945,#23946,
#23947,#23948,#23949,#23950,#23951,#23952,#23953,#23954,#23955,#23956,#23957,
#23958,#23959,#23960,#23961,#23962,#23963,#23964,#23965,#23966,#23967,#23968,
#23969,#23970,#23971,#23972,#23973,#23974,#23975,#23976,#23977,#23978,#23979,
#23980,#23981,#23982,#23983,#23984,#23985,#23986,#23987,#23988,#23989,#23990,
#23991,#23992,#23993,#23994,#23995,#23996,#23997,#23998,#23999,#24000,#24001,
#24002,#24003,#24004,#24005,#24006,#24007,#24008,#24009,#24010,#24011,#24012,
#24013,#24014,#24015,#24016,#24017,#24018,#24019,#24020,#24021,#24022,#24023,
#24024,#24025,#24026,#24027,#24028,#24029,#24030,#24031,#24032,#24033,#24034,
#24035,#24036,#24037,#24038,#24039,#24040,#24041,#24042,#24043,#24044,#24045,
#24046,#24047,#24048,#24049,#24050,#24051,#24052,#24053,#24054,#24055,#24056,
#24057,#24058,#24059,#24060,#24061,#24062,#24063,#24064,#24065,#24066,#24067,
#24068,#24069,#24070,#24071,#24072,#24073,#24074,#24075,#24076,#24077,#24078,
#24079,#24080,#24081,#24082,#24083,#24084,#24085,#24086,#24087,#24088,#24089,
#24090,#24091,#24092,#24093,#24094,#24095,#24096,#24097,#24098,#24099,#24100,
#24101,#24102,#24103));
#26252=AXIS2_PLACEMENT_3D('',#39974,#31113,#31114);
#26253=AXIS2_PLACEMENT_3D('',#39975,#31115,#31116);
#26254=AXIS2_PLACEMENT_3D('',#39994,#31118,#31119);
#26255=AXIS2_PLACEMENT_3D('',#39997,#31121,#31122);
#26256=AXIS2_PLACEMENT_3D('',#39999,#31123,#31124);
#26257=AXIS2_PLACEMENT_3D('',#40010,#31125,#31126);
#26258=AXIS2_PLACEMENT_3D('',#40058,#31128,#31129);
#26259=AXIS2_PLACEMENT_3D('',#40109,#31131,#31132);
#26260=AXIS2_PLACEMENT_3D('',#40157,#31134,#31135);
#26261=AXIS2_PLACEMENT_3D('',#40205,#31137,#31138);
#26262=AXIS2_PLACEMENT_3D('',#40259,#31140,#31141);
#26263=AXIS2_PLACEMENT_3D('',#40307,#31143,#31144);
#26264=AXIS2_PLACEMENT_3D('',#40355,#31146,#31147);
#26265=AXIS2_PLACEMENT_3D('',#40409,#31149,#31150);
#26266=AXIS2_PLACEMENT_3D('',#40457,#31152,#31153);
#26267=AXIS2_PLACEMENT_3D('',#40505,#31155,#31156);
#26268=AXIS2_PLACEMENT_3D('',#40553,#31158,#31159);
#26269=AXIS2_PLACEMENT_3D('',#40604,#31161,#31162);
#26270=AXIS2_PLACEMENT_3D('',#40652,#31164,#31165);
#26271=AXIS2_PLACEMENT_3D('',#40700,#31167,#31168);
#26272=AXIS2_PLACEMENT_3D('',#40754,#31170,#31171);
#26273=AXIS2_PLACEMENT_3D('',#40802,#31173,#31174);
#26274=AXIS2_PLACEMENT_3D('',#40850,#31176,#31177);
#26275=AXIS2_PLACEMENT_3D('',#40904,#31179,#31180);
#26276=AXIS2_PLACEMENT_3D('',#40952,#31182,#31183);
#26277=AXIS2_PLACEMENT_3D('',#41000,#31185,#31186);
#26278=AXIS2_PLACEMENT_3D('',#41048,#31188,#31189);
#26279=AXIS2_PLACEMENT_3D('',#41099,#31191,#31192);
#26280=AXIS2_PLACEMENT_3D('',#41147,#31194,#31195);
#26281=AXIS2_PLACEMENT_3D('',#41195,#31197,#31198);
#26282=AXIS2_PLACEMENT_3D('',#41249,#31200,#31201);
#26283=AXIS2_PLACEMENT_3D('',#41297,#31203,#31204);
#26284=AXIS2_PLACEMENT_3D('',#41345,#31206,#31207);
#26285=AXIS2_PLACEMENT_3D('',#41358,#31209,#31210);
#26286=AXIS2_PLACEMENT_3D('',#41364,#31211,#31212);
#26287=AXIS2_PLACEMENT_3D('',#41389,#31214,#31215);
#26288=AXIS2_PLACEMENT_3D('',#41413,#31217,#31218);
#26289=AXIS2_PLACEMENT_3D('',#41438,#31220,#31221);
#26290=AXIS2_PLACEMENT_3D('',#41463,#31223,#31224);
#26291=AXIS2_PLACEMENT_3D('',#41487,#31226,#31227);
#26292=AXIS2_PLACEMENT_3D('',#41512,#31229,#31230);
#26293=AXIS2_PLACEMENT_3D('',#41536,#31232,#31233);
#26294=AXIS2_PLACEMENT_3D('',#41561,#31235,#31236);
#26295=AXIS2_PLACEMENT_3D('',#41585,#31238,#31239);
#26296=AXIS2_PLACEMENT_3D('',#41610,#31241,#31242);
#26297=AXIS2_PLACEMENT_3D('',#41635,#31244,#31245);
#26298=AXIS2_PLACEMENT_3D('',#41659,#31247,#31248);
#26299=AXIS2_PLACEMENT_3D('',#41684,#31250,#31251);
#26300=AXIS2_PLACEMENT_3D('',#41709,#31253,#31254);
#26301=AXIS2_PLACEMENT_3D('',#41733,#31256,#31257);
#26302=AXIS2_PLACEMENT_3D('',#41758,#31259,#31260);
#26303=AXIS2_PLACEMENT_3D('',#41783,#31262,#31263);
#26304=AXIS2_PLACEMENT_3D('',#41807,#31265,#31266);
#26305=AXIS2_PLACEMENT_3D('',#41831,#31268,#31269);
#26306=AXIS2_PLACEMENT_3D('',#41856,#31271,#31272);
#26307=AXIS2_PLACEMENT_3D('',#41881,#31274,#31275);
#26308=AXIS2_PLACEMENT_3D('',#41905,#31277,#31278);
#26309=AXIS2_PLACEMENT_3D('',#41930,#31280,#31281);
#26310=AXIS2_PLACEMENT_3D('',#41955,#31283,#31284);
#26311=AXIS2_PLACEMENT_3D('',#41979,#31286,#31287);
#26312=AXIS2_PLACEMENT_3D('',#42004,#31289,#31290);
#26313=AXIS2_PLACEMENT_3D('',#42029,#31292,#31293);
#26314=AXIS2_PLACEMENT_3D('',#42034,#31295,#31296);
#26315=AXIS2_PLACEMENT_3D('',#42054,#31297,#31298);
#26316=AXIS2_PLACEMENT_3D('',#42103,#31299,#31300);
#26317=AXIS2_PLACEMENT_3D('',#42105,#31301,#31302);
#26318=AXIS2_PLACEMENT_3D('',#42964,#31303,#31304);
#26319=AXIS2_PLACEMENT_3D('',#43014,#31305,#31306);
#26320=AXIS2_PLACEMENT_3D('',#43015,#31307,#31308);
#26321=AXIS2_PLACEMENT_3D('',#43771,#31309,#31310);
#26322=AXIS2_PLACEMENT_3D('',#43774,#31311,#31312);
#26323=AXIS2_PLACEMENT_3D('',#43778,#31315,#31316);
#26324=AXIS2_PLACEMENT_3D('',#43786,#31319,#31320);
#26325=AXIS2_PLACEMENT_3D('',#43792,#31322,#31323);
#26326=AXIS2_PLACEMENT_3D('',#43795,#31324,#31325);
#26327=AXIS2_PLACEMENT_3D('',#43799,#31328,#31329);
#26328=AXIS2_PLACEMENT_3D('',#43807,#31332,#31333);
#26329=AXIS2_PLACEMENT_3D('',#43813,#31335,#31336);
#26330=AXIS2_PLACEMENT_3D('',#43816,#31337,#31338);
#26331=AXIS2_PLACEMENT_3D('',#43820,#31341,#31342);
#26332=AXIS2_PLACEMENT_3D('',#43828,#31345,#31346);
#26333=AXIS2_PLACEMENT_3D('',#43834,#31348,#31349);
#26334=AXIS2_PLACEMENT_3D('',#43837,#31350,#31351);
#26335=AXIS2_PLACEMENT_3D('',#43841,#31354,#31355);
#26336=AXIS2_PLACEMENT_3D('',#43849,#31358,#31359);
#26337=AXIS2_PLACEMENT_3D('',#43855,#31361,#31362);
#26338=AXIS2_PLACEMENT_3D('',#43858,#31363,#31364);
#26339=AXIS2_PLACEMENT_3D('',#43862,#31367,#31368);
#26340=AXIS2_PLACEMENT_3D('',#43870,#31371,#31372);
#26341=AXIS2_PLACEMENT_3D('',#43876,#31374,#31375);
#26342=AXIS2_PLACEMENT_3D('',#43879,#31376,#31377);
#26343=AXIS2_PLACEMENT_3D('',#43883,#31380,#31381);
#26344=AXIS2_PLACEMENT_3D('',#43891,#31384,#31385);
#26345=AXIS2_PLACEMENT_3D('',#43897,#31387,#31388);
#26346=AXIS2_PLACEMENT_3D('',#43900,#31389,#31390);
#26347=AXIS2_PLACEMENT_3D('',#43904,#31393,#31394);
#26348=AXIS2_PLACEMENT_3D('',#43912,#31397,#31398);
#26349=AXIS2_PLACEMENT_3D('',#43918,#31400,#31401);
#26350=AXIS2_PLACEMENT_3D('',#43921,#31402,#31403);
#26351=AXIS2_PLACEMENT_3D('',#43925,#31406,#31407);
#26352=AXIS2_PLACEMENT_3D('',#43933,#31410,#31411);
#26353=AXIS2_PLACEMENT_3D('',#43939,#31413,#31414);
#26354=AXIS2_PLACEMENT_3D('',#43942,#31415,#31416);
#26355=AXIS2_PLACEMENT_3D('',#43946,#31419,#31420);
#26356=AXIS2_PLACEMENT_3D('',#43954,#31423,#31424);
#26357=AXIS2_PLACEMENT_3D('',#43960,#31426,#31427);
#26358=AXIS2_PLACEMENT_3D('',#43963,#31428,#31429);
#26359=AXIS2_PLACEMENT_3D('',#43967,#31432,#31433);
#26360=AXIS2_PLACEMENT_3D('',#43975,#31436,#31437);
#26361=AXIS2_PLACEMENT_3D('',#43981,#31439,#31440);
#26362=AXIS2_PLACEMENT_3D('',#43984,#31441,#31442);
#26363=AXIS2_PLACEMENT_3D('',#43988,#31445,#31446);
#26364=AXIS2_PLACEMENT_3D('',#43996,#31449,#31450);
#26365=AXIS2_PLACEMENT_3D('',#44002,#31452,#31453);
#26366=AXIS2_PLACEMENT_3D('',#44005,#31454,#31455);
#26367=AXIS2_PLACEMENT_3D('',#44009,#31458,#31459);
#26368=AXIS2_PLACEMENT_3D('',#44017,#31462,#31463);
#26369=AXIS2_PLACEMENT_3D('',#44023,#31465,#31466);
#26370=AXIS2_PLACEMENT_3D('',#44026,#31467,#31468);
#26371=AXIS2_PLACEMENT_3D('',#44030,#31471,#31472);
#26372=AXIS2_PLACEMENT_3D('',#44038,#31475,#31476);
#26373=AXIS2_PLACEMENT_3D('',#44044,#31478,#31479);
#26374=AXIS2_PLACEMENT_3D('',#44047,#31480,#31481);
#26375=AXIS2_PLACEMENT_3D('',#44051,#31484,#31485);
#26376=AXIS2_PLACEMENT_3D('',#44059,#31488,#31489);
#26377=AXIS2_PLACEMENT_3D('',#44065,#31491,#31492);
#26378=AXIS2_PLACEMENT_3D('',#44068,#31493,#31494);
#26379=AXIS2_PLACEMENT_3D('',#44072,#31497,#31498);
#26380=AXIS2_PLACEMENT_3D('',#44080,#31501,#31502);
#26381=AXIS2_PLACEMENT_3D('',#44086,#31504,#31505);
#26382=AXIS2_PLACEMENT_3D('',#44089,#31506,#31507);
#26383=AXIS2_PLACEMENT_3D('',#44093,#31510,#31511);
#26384=AXIS2_PLACEMENT_3D('',#44101,#31514,#31515);
#26385=AXIS2_PLACEMENT_3D('',#44107,#31517,#31518);
#26386=AXIS2_PLACEMENT_3D('',#44110,#31519,#31520);
#26387=AXIS2_PLACEMENT_3D('',#44114,#31523,#31524);
#26388=AXIS2_PLACEMENT_3D('',#44122,#31527,#31528);
#26389=AXIS2_PLACEMENT_3D('',#44128,#31530,#31531);
#26390=AXIS2_PLACEMENT_3D('',#44131,#31532,#31533);
#26391=AXIS2_PLACEMENT_3D('',#44136,#31536,#31537);
#26392=AXIS2_PLACEMENT_3D('',#44137,#31538,#31539);
#26393=AXIS2_PLACEMENT_3D('',#44145,#31542,#31543);
#26394=AXIS2_PLACEMENT_3D('',#44151,#31545,#31546);
#26395=AXIS2_PLACEMENT_3D('',#44154,#31547,#31548);
#26396=AXIS2_PLACEMENT_3D('',#44158,#31551,#31552);
#26397=AXIS2_PLACEMENT_3D('',#44166,#31555,#31556);
#26398=AXIS2_PLACEMENT_3D('',#44172,#31558,#31559);
#26399=AXIS2_PLACEMENT_3D('',#44175,#31560,#31561);
#26400=AXIS2_PLACEMENT_3D('',#44179,#31564,#31565);
#26401=AXIS2_PLACEMENT_3D('',#44187,#31568,#31569);
#26402=AXIS2_PLACEMENT_3D('',#44193,#31571,#31572);
#26403=AXIS2_PLACEMENT_3D('',#44196,#31573,#31574);
#26404=AXIS2_PLACEMENT_3D('',#44200,#31577,#31578);
#26405=AXIS2_PLACEMENT_3D('',#44208,#31581,#31582);
#26406=AXIS2_PLACEMENT_3D('',#44214,#31584,#31585);
#26407=AXIS2_PLACEMENT_3D('',#44217,#31586,#31587);
#26408=AXIS2_PLACEMENT_3D('',#44221,#31590,#31591);
#26409=AXIS2_PLACEMENT_3D('',#44229,#31594,#31595);
#26410=AXIS2_PLACEMENT_3D('',#44235,#31597,#31598);
#26411=AXIS2_PLACEMENT_3D('',#44238,#31599,#31600);
#26412=AXIS2_PLACEMENT_3D('',#44242,#31603,#31604);
#26413=AXIS2_PLACEMENT_3D('',#44250,#31607,#31608);
#26414=AXIS2_PLACEMENT_3D('',#44256,#31610,#31611);
#26415=AXIS2_PLACEMENT_3D('',#44259,#31612,#31613);
#26416=AXIS2_PLACEMENT_3D('',#44263,#31616,#31617);
#26417=AXIS2_PLACEMENT_3D('',#44271,#31620,#31621);
#26418=AXIS2_PLACEMENT_3D('',#44277,#31623,#31624);
#26419=AXIS2_PLACEMENT_3D('',#44280,#31625,#31626);
#26420=AXIS2_PLACEMENT_3D('',#44284,#31629,#31630);
#26421=AXIS2_PLACEMENT_3D('',#44292,#31633,#31634);
#26422=AXIS2_PLACEMENT_3D('',#44298,#31636,#31637);
#26423=AXIS2_PLACEMENT_3D('',#44301,#31638,#31639);
#26424=AXIS2_PLACEMENT_3D('',#44305,#31642,#31643);
#26425=AXIS2_PLACEMENT_3D('',#44313,#31646,#31647);
#26426=AXIS2_PLACEMENT_3D('',#44319,#31649,#31650);
#26427=AXIS2_PLACEMENT_3D('',#44322,#31651,#31652);
#26428=AXIS2_PLACEMENT_3D('',#44326,#31655,#31656);
#26429=AXIS2_PLACEMENT_3D('',#44334,#31659,#31660);
#26430=AXIS2_PLACEMENT_3D('',#44340,#31662,#31663);
#26431=AXIS2_PLACEMENT_3D('',#44343,#31664,#31665);
#26432=AXIS2_PLACEMENT_3D('',#44347,#31668,#31669);
#26433=AXIS2_PLACEMENT_3D('',#44355,#31672,#31673);
#26434=AXIS2_PLACEMENT_3D('',#44361,#31675,#31676);
#26435=AXIS2_PLACEMENT_3D('',#44364,#31677,#31678);
#26436=AXIS2_PLACEMENT_3D('',#44368,#31681,#31682);
#26437=AXIS2_PLACEMENT_3D('',#44376,#31685,#31686);
#26438=AXIS2_PLACEMENT_3D('',#44382,#31688,#31689);
#26439=AXIS2_PLACEMENT_3D('',#44385,#31690,#31691);
#26440=AXIS2_PLACEMENT_3D('',#44389,#31694,#31695);
#26441=AXIS2_PLACEMENT_3D('',#44397,#31698,#31699);
#26442=AXIS2_PLACEMENT_3D('',#44403,#31701,#31702);
#26443=AXIS2_PLACEMENT_3D('',#44406,#31703,#31704);
#26444=AXIS2_PLACEMENT_3D('',#44410,#31707,#31708);
#26445=AXIS2_PLACEMENT_3D('',#44418,#31711,#31712);
#26446=AXIS2_PLACEMENT_3D('',#44424,#31714,#31715);
#26447=AXIS2_PLACEMENT_3D('',#44427,#31716,#31717);
#26448=AXIS2_PLACEMENT_3D('',#44431,#31720,#31721);
#26449=AXIS2_PLACEMENT_3D('',#44439,#31724,#31725);
#26450=AXIS2_PLACEMENT_3D('',#44445,#31727,#31728);
#26451=AXIS2_PLACEMENT_3D('',#44448,#31729,#31730);
#26452=AXIS2_PLACEMENT_3D('',#44452,#31733,#31734);
#26453=AXIS2_PLACEMENT_3D('',#44460,#31737,#31738);
#26454=AXIS2_PLACEMENT_3D('',#44466,#31740,#31741);
#26455=AXIS2_PLACEMENT_3D('',#44469,#31742,#31743);
#26456=AXIS2_PLACEMENT_3D('',#44473,#31746,#31747);
#26457=AXIS2_PLACEMENT_3D('',#44481,#31750,#31751);
#26458=AXIS2_PLACEMENT_3D('',#44487,#31753,#31754);
#26459=AXIS2_PLACEMENT_3D('',#44490,#31755,#31756);
#26460=AXIS2_PLACEMENT_3D('',#44494,#31759,#31760);
#26461=AXIS2_PLACEMENT_3D('',#44502,#31763,#31764);
#26462=AXIS2_PLACEMENT_3D('',#44508,#31766,#31767);
#26463=AXIS2_PLACEMENT_3D('',#44509,#31768,#31769);
#26464=AXIS2_PLACEMENT_3D('',#44510,#31770,#31771);
#26465=AXIS2_PLACEMENT_3D('',#44511,#31772,#31773);
#26466=AXIS2_PLACEMENT_3D('',#44512,#31774,#31775);
#26467=AXIS2_PLACEMENT_3D('',#44513,#31776,#31777);
#26468=AXIS2_PLACEMENT_3D('',#44514,#31778,#31779);
#26469=AXIS2_PLACEMENT_3D('',#44515,#31780,#31781);
#26470=AXIS2_PLACEMENT_3D('',#44516,#31782,#31783);
#26471=AXIS2_PLACEMENT_3D('',#44517,#31784,#31785);
#26472=AXIS2_PLACEMENT_3D('',#44518,#31786,#31787);
#26473=AXIS2_PLACEMENT_3D('',#44519,#31788,#31789);
#26474=AXIS2_PLACEMENT_3D('',#44520,#31790,#31791);
#26475=AXIS2_PLACEMENT_3D('',#44521,#31792,#31793);
#26476=AXIS2_PLACEMENT_3D('',#44522,#31794,#31795);
#26477=AXIS2_PLACEMENT_3D('',#44523,#31796,#31797);
#26478=AXIS2_PLACEMENT_3D('',#44524,#31798,#31799);
#26479=AXIS2_PLACEMENT_3D('',#44525,#31800,#31801);
#26480=AXIS2_PLACEMENT_3D('',#44528,#31803,#31804);
#26481=AXIS2_PLACEMENT_3D('',#44529,#31805,#31806);
#26482=AXIS2_PLACEMENT_3D('',#44530,#31807,#31808);
#26483=AXIS2_PLACEMENT_3D('',#44531,#31809,#31810);
#26484=AXIS2_PLACEMENT_3D('',#44532,#31811,#31812);
#26485=AXIS2_PLACEMENT_3D('',#44533,#31813,#31814);
#26486=AXIS2_PLACEMENT_3D('',#44534,#31815,#31816);
#26487=AXIS2_PLACEMENT_3D('',#44535,#31817,#31818);
#26488=AXIS2_PLACEMENT_3D('',#44536,#31819,#31820);
#26489=AXIS2_PLACEMENT_3D('',#44537,#31821,#31822);
#26490=AXIS2_PLACEMENT_3D('',#44538,#31823,#31824);
#26491=AXIS2_PLACEMENT_3D('',#44539,#31825,#31826);
#26492=AXIS2_PLACEMENT_3D('',#44540,#31827,#31828);
#26493=AXIS2_PLACEMENT_3D('',#44541,#31829,#31830);
#26494=AXIS2_PLACEMENT_3D('',#44542,#31831,#31832);
#26495=AXIS2_PLACEMENT_3D('',#44543,#31833,#31834);
#26496=AXIS2_PLACEMENT_3D('',#44544,#31835,#31836);
#26497=AXIS2_PLACEMENT_3D('',#44545,#31837,#31838);
#26498=AXIS2_PLACEMENT_3D('',#44547,#31839,#31840);
#26499=AXIS2_PLACEMENT_3D('',#44551,#31842,#31843);
#26500=AXIS2_PLACEMENT_3D('',#44554,#31845,#31846);
#26501=AXIS2_PLACEMENT_3D('',#44555,#31847,#31848);
#26502=AXIS2_PLACEMENT_3D('',#44563,#31851,#31852);
#26503=AXIS2_PLACEMENT_3D('',#44568,#31854,#31855);
#26504=AXIS2_PLACEMENT_3D('',#44569,#31856,#31857);
#26505=AXIS2_PLACEMENT_3D('',#44571,#31858,#31859);
#26506=AXIS2_PLACEMENT_3D('',#44573,#31861,#31862);
#26507=AXIS2_PLACEMENT_3D('',#44577,#31864,#31865);
#26508=AXIS2_PLACEMENT_3D('',#44578,#31866,#31867);
#26509=AXIS2_PLACEMENT_3D('',#44587,#31872,#31873);
#26510=AXIS2_PLACEMENT_3D('',#44593,#31877,#31878);
#26511=AXIS2_PLACEMENT_3D('',#44599,#31882,#31883);
#26512=AXIS2_PLACEMENT_3D('',#44605,#31887,#31888);
#26513=AXIS2_PLACEMENT_3D('',#44611,#31892,#31893);
#26514=AXIS2_PLACEMENT_3D('',#44614,#31896,#31897);
#26515=AXIS2_PLACEMENT_3D('',#44615,#31898,#31899);
#26516=AXIS2_PLACEMENT_3D('',#44617,#31900,#31901);
#26517=AXIS2_PLACEMENT_3D('',#44618,#31902,#31903);
#26518=AXIS2_PLACEMENT_3D('',#44620,#31905,#31906);
#26519=AXIS2_PLACEMENT_3D('',#44621,#31907,#31908);
#26520=AXIS2_PLACEMENT_3D('',#44622,#31909,#31910);
#26521=AXIS2_PLACEMENT_3D('',#44624,#31911,#31912);
#26522=AXIS2_PLACEMENT_3D('',#44626,#31914,#31915);
#26523=AXIS2_PLACEMENT_3D('',#44627,#31916,#31917);
#31113=DIRECTION('axis',(0.,0.,1.));
#31114=DIRECTION('refdir',(1.,0.,0.));
#31115=DIRECTION('center_axis',(0.,0.,1.));
#31116=DIRECTION('ref_axis',(1.,0.,0.));
#31117=DIRECTION('',(0.,0.,-1.));
#31118=DIRECTION('center_axis',(0.,0.,-1.));
#31119=DIRECTION('ref_axis',(1.,0.,0.));
#31120=DIRECTION('',(0.,0.,-1.));
#31121=DIRECTION('center_axis',(0.,0.,1.));
#31122=DIRECTION('ref_axis',(1.,0.,0.));
#31123=DIRECTION('center_axis',(0.,0.,-1.));
#31124=DIRECTION('ref_axis',(1.,0.,0.));
#31125=DIRECTION('center_axis',(0.,0.,1.));
#31126=DIRECTION('ref_axis',(1.,0.,0.));
#31127=DIRECTION('',(0.,0.,-1.));
#31128=DIRECTION('center_axis',(0.,0.,1.));
#31129=DIRECTION('ref_axis',(1.,0.,0.));
#31130=DIRECTION('',(0.,0.,-1.));
#31131=DIRECTION('center_axis',(0.,0.,1.));
#31132=DIRECTION('ref_axis',(1.,0.,0.));
#31133=DIRECTION('',(0.,0.,-1.));
#31134=DIRECTION('center_axis',(0.,0.,1.));
#31135=DIRECTION('ref_axis',(1.,0.,0.));
#31136=DIRECTION('',(0.,0.,-1.));
#31137=DIRECTION('center_axis',(0.,0.,1.));
#31138=DIRECTION('ref_axis',(1.,0.,0.));
#31139=DIRECTION('',(0.,0.,-1.));
#31140=DIRECTION('center_axis',(0.,0.,1.));
#31141=DIRECTION('ref_axis',(1.,0.,0.));
#31142=DIRECTION('',(0.,0.,-1.));
#31143=DIRECTION('center_axis',(0.,0.,1.));
#31144=DIRECTION('ref_axis',(1.,0.,0.));
#31145=DIRECTION('',(0.,0.,-1.));
#31146=DIRECTION('center_axis',(0.,0.,1.));
#31147=DIRECTION('ref_axis',(1.,0.,0.));
#31148=DIRECTION('',(0.,0.,-1.));
#31149=DIRECTION('center_axis',(0.,0.,1.));
#31150=DIRECTION('ref_axis',(1.,0.,0.));
#31151=DIRECTION('',(0.,0.,-1.));
#31152=DIRECTION('center_axis',(0.,0.,1.));
#31153=DIRECTION('ref_axis',(1.,0.,0.));
#31154=DIRECTION('',(0.,0.,-1.));
#31155=DIRECTION('center_axis',(0.,0.,1.));
#31156=DIRECTION('ref_axis',(1.,0.,0.));
#31157=DIRECTION('',(0.,0.,-1.));
#31158=DIRECTION('center_axis',(0.,0.,1.));
#31159=DIRECTION('ref_axis',(1.,0.,0.));
#31160=DIRECTION('',(0.,0.,-1.));
#31161=DIRECTION('center_axis',(0.,0.,1.));
#31162=DIRECTION('ref_axis',(1.,0.,0.));
#31163=DIRECTION('',(0.,0.,-1.));
#31164=DIRECTION('center_axis',(0.,0.,1.));
#31165=DIRECTION('ref_axis',(1.,0.,0.));
#31166=DIRECTION('',(0.,0.,-1.));
#31167=DIRECTION('center_axis',(0.,0.,1.));
#31168=DIRECTION('ref_axis',(1.,0.,0.));
#31169=DIRECTION('',(0.,0.,-1.));
#31170=DIRECTION('center_axis',(0.,0.,1.));
#31171=DIRECTION('ref_axis',(1.,0.,0.));
#31172=DIRECTION('',(0.,0.,-1.));
#31173=DIRECTION('center_axis',(0.,0.,1.));
#31174=DIRECTION('ref_axis',(1.,0.,0.));
#31175=DIRECTION('',(0.,0.,-1.));
#31176=DIRECTION('center_axis',(0.,0.,1.));
#31177=DIRECTION('ref_axis',(1.,0.,0.));
#31178=DIRECTION('',(0.,0.,-1.));
#31179=DIRECTION('center_axis',(0.,0.,1.));
#31180=DIRECTION('ref_axis',(1.,0.,0.));
#31181=DIRECTION('',(0.,0.,-1.));
#31182=DIRECTION('center_axis',(0.,0.,1.));
#31183=DIRECTION('ref_axis',(1.,0.,0.));
#31184=DIRECTION('',(0.,0.,-1.));
#31185=DIRECTION('center_axis',(0.,0.,1.));
#31186=DIRECTION('ref_axis',(1.,0.,0.));
#31187=DIRECTION('',(0.,0.,-1.));
#31188=DIRECTION('center_axis',(0.,0.,1.));
#31189=DIRECTION('ref_axis',(1.,0.,0.));
#31190=DIRECTION('',(0.,0.,-1.));
#31191=DIRECTION('center_axis',(0.,0.,1.));
#31192=DIRECTION('ref_axis',(1.,0.,0.));
#31193=DIRECTION('',(0.,0.,-1.));
#31194=DIRECTION('center_axis',(0.,0.,1.));
#31195=DIRECTION('ref_axis',(1.,0.,0.));
#31196=DIRECTION('',(0.,0.,-1.));
#31197=DIRECTION('center_axis',(0.,0.,1.));
#31198=DIRECTION('ref_axis',(1.,0.,0.));
#31199=DIRECTION('',(0.,0.,-1.));
#31200=DIRECTION('center_axis',(0.,0.,1.));
#31201=DIRECTION('ref_axis',(1.,0.,0.));
#31202=DIRECTION('',(0.,0.,-1.));
#31203=DIRECTION('center_axis',(0.,0.,1.));
#31204=DIRECTION('ref_axis',(1.,0.,0.));
#31205=DIRECTION('',(0.,0.,-1.));
#31206=DIRECTION('center_axis',(0.,0.,1.));
#31207=DIRECTION('ref_axis',(-0.00388812637901143,-0.999992441208063,0.));
#31208=DIRECTION('',(0.,0.,1.));
#31209=DIRECTION('center_axis',(0.,0.,1.));
#31210=DIRECTION('ref_axis',(1.,-1.57698425990146E-13,0.));
#31211=DIRECTION('center_axis',(0.,0.,1.));
#31212=DIRECTION('ref_axis',(1.,-1.57698425990146E-13,0.));
#31213=DIRECTION('',(0.,0.,1.));
#31214=DIRECTION('center_axis',(0.,0.,1.));
#31215=DIRECTION('ref_axis',(1.,-1.57698425990146E-13,0.));
#31216=DIRECTION('',(0.,0.,1.));
#31217=DIRECTION('center_axis',(0.,0.,1.));
#31218=DIRECTION('ref_axis',(1.,-1.57698425990146E-13,0.));
#31219=DIRECTION('',(0.,0.,1.));
#31220=DIRECTION('center_axis',(0.,0.,1.));
#31221=DIRECTION('ref_axis',(1.,-1.57698425990146E-13,0.));
#31222=DIRECTION('',(0.,0.,1.));
#31223=DIRECTION('center_axis',(0.,0.,1.));
#31224=DIRECTION('ref_axis',(1.,-1.57698425990146E-13,0.));
#31225=DIRECTION('',(0.,0.,1.));
#31226=DIRECTION('center_axis',(0.,0.,1.));
#31227=DIRECTION('ref_axis',(1.,-1.57698425990146E-13,0.));
#31228=DIRECTION('',(0.,0.,1.));
#31229=DIRECTION('center_axis',(0.,0.,1.));
#31230=DIRECTION('ref_axis',(1.,-1.57698425990146E-13,0.));
#31231=DIRECTION('',(0.,0.,1.));
#31232=DIRECTION('center_axis',(0.,0.,1.));
#31233=DIRECTION('ref_axis',(1.,-1.57698425990146E-13,0.));
#31234=DIRECTION('',(0.,0.,1.));
#31235=DIRECTION('center_axis',(0.,0.,1.));
#31236=DIRECTION('ref_axis',(1.,-1.57698425990146E-13,0.));
#31237=DIRECTION('',(0.,0.,1.));
#31238=DIRECTION('center_axis',(0.,0.,1.));
#31239=DIRECTION('ref_axis',(1.,-1.57698425990146E-13,0.));
#31240=DIRECTION('',(0.,0.,1.));
#31241=DIRECTION('center_axis',(0.,0.,1.));
#31242=DIRECTION('ref_axis',(1.,-1.57698425990146E-13,0.));
#31243=DIRECTION('',(0.,0.,1.));
#31244=DIRECTION('center_axis',(0.,0.,1.));
#31245=DIRECTION('ref_axis',(1.,-1.57698425990146E-13,0.));
#31246=DIRECTION('',(0.,0.,1.));
#31247=DIRECTION('center_axis',(0.,0.,1.));
#31248=DIRECTION('ref_axis',(1.,-1.57698425990146E-13,0.));
#31249=DIRECTION('',(0.,0.,1.));
#31250=DIRECTION('center_axis',(0.,0.,1.));
#31251=DIRECTION('ref_axis',(1.,-1.57698425990146E-13,0.));
#31252=DIRECTION('',(0.,0.,1.));
#31253=DIRECTION('center_axis',(0.,0.,1.));
#31254=DIRECTION('ref_axis',(1.,-1.57698425990146E-13,0.));
#31255=DIRECTION('',(0.,0.,1.));
#31256=DIRECTION('center_axis',(0.,0.,1.));
#31257=DIRECTION('ref_axis',(1.,-1.57698425990146E-13,0.));
#31258=DIRECTION('',(0.,0.,1.));
#31259=DIRECTION('center_axis',(0.,0.,1.));
#31260=DIRECTION('ref_axis',(1.,-1.57698425990146E-13,0.));
#31261=DIRECTION('',(0.,0.,1.));
#31262=DIRECTION('center_axis',(0.,0.,1.));
#31263=DIRECTION('ref_axis',(1.,-1.57698425990146E-13,0.));
#31264=DIRECTION('',(0.,0.,1.));
#31265=DIRECTION('center_axis',(0.,0.,1.));
#31266=DIRECTION('ref_axis',(1.,-1.57698425990146E-13,0.));
#31267=DIRECTION('',(0.,0.,1.));
#31268=DIRECTION('center_axis',(0.,0.,1.));
#31269=DIRECTION('ref_axis',(1.,-1.57698425990146E-13,0.));
#31270=DIRECTION('',(0.,0.,1.));
#31271=DIRECTION('center_axis',(0.,0.,1.));
#31272=DIRECTION('ref_axis',(1.,-1.57698425990146E-13,0.));
#31273=DIRECTION('',(0.,0.,1.));
#31274=DIRECTION('center_axis',(0.,0.,1.));
#31275=DIRECTION('ref_axis',(1.,-1.57698425990146E-13,0.));
#31276=DIRECTION('',(0.,0.,1.));
#31277=DIRECTION('center_axis',(0.,0.,1.));
#31278=DIRECTION('ref_axis',(1.,-1.57698425990146E-13,0.));
#31279=DIRECTION('',(0.,0.,1.));
#31280=DIRECTION('center_axis',(0.,0.,1.));
#31281=DIRECTION('ref_axis',(1.,-1.57698425990146E-13,0.));
#31282=DIRECTION('',(0.,0.,1.));
#31283=DIRECTION('center_axis',(0.,0.,1.));
#31284=DIRECTION('ref_axis',(1.,-1.57698425990146E-13,0.));
#31285=DIRECTION('',(0.,0.,1.));
#31286=DIRECTION('center_axis',(0.,0.,1.));
#31287=DIRECTION('ref_axis',(1.,-1.57698425990146E-13,0.));
#31288=DIRECTION('',(0.,0.,1.));
#31289=DIRECTION('center_axis',(0.,0.,1.));
#31290=DIRECTION('ref_axis',(1.,-1.57698425990146E-13,0.));
#31291=DIRECTION('',(0.,0.,1.));
#31292=DIRECTION('center_axis',(0.,0.,1.));
#31293=DIRECTION('ref_axis',(1.,-1.57698425990146E-13,0.));
#31294=DIRECTION('',(0.,0.,1.));
#31295=DIRECTION('center_axis',(0.,0.,-1.));
#31296=DIRECTION('ref_axis',(1.,-1.57698425990146E-13,0.));
#31297=DIRECTION('center_axis',(0.,0.,1.));
#31298=DIRECTION('ref_axis',(1.,0.,0.));
#31299=DIRECTION('center_axis',(0.,0.,1.));
#31300=DIRECTION('ref_axis',(1.,0.,0.));
#31301=DIRECTION('center_axis',(0.,0.,1.));
#31302=DIRECTION('ref_axis',(1.,0.,0.));
#31303=DIRECTION('center_axis',(0.,0.,1.));
#31304=DIRECTION('ref_axis',(1.,0.,0.));
#31305=DIRECTION('center_axis',(0.,0.,-1.));
#31306=DIRECTION('ref_axis',(1.,-1.57698425990146E-13,0.));
#31307=DIRECTION('center_axis',(0.,0.,1.));
#31308=DIRECTION('ref_axis',(-0.952281269972968,0.30522185842215,0.));
#31309=DIRECTION('center_axis',(0.,0.,1.));
#31310=DIRECTION('ref_axis',(0.984807753012208,-0.17364817766693,0.));
#31311=DIRECTION('center_axis',(0.,0.,-1.));
#31312=DIRECTION('ref_axis',(1.,0.,0.));
#31313=DIRECTION('',(-0.996089805327885,-0.0883464754353932,0.));
#31314=DIRECTION('',(0.905801965515954,-0.423701309022563,0.));
#31315=DIRECTION('center_axis',(-0.423701309022563,-0.905801965515954,0.));
#31316=DIRECTION('ref_axis',(0.905801965515954,-0.423701309022563,0.));
#31317=DIRECTION('',(0.,0.,1.));
#31318=DIRECTION('',(0.,0.,1.));
#31319=DIRECTION('center_axis',(-0.0883464754353932,0.996089805327885,0.));
#31320=DIRECTION('ref_axis',(-0.996089805327885,-0.0883464754353932,0.));
#31321=DIRECTION('',(0.,0.,-1.));
#31322=DIRECTION('center_axis',(0.,0.,1.));
#31323=DIRECTION('ref_axis',(0.939692620785908,-0.342020143325669,0.));
#31324=DIRECTION('center_axis',(0.,0.,-1.));
#31325=DIRECTION('ref_axis',(1.,0.,0.));
#31326=DIRECTION('',(-0.996298167445974,0.0859648855277176,0.));
#31327=DIRECTION('',(0.818465838146947,-0.574555194725812,0.));
#31328=DIRECTION('center_axis',(-0.574555194725812,-0.818465838146947,0.));
#31329=DIRECTION('ref_axis',(0.818465838146947,-0.574555194725812,0.));
#31330=DIRECTION('',(0.,0.,1.));
#31331=DIRECTION('',(0.,0.,1.));
#31332=DIRECTION('center_axis',(0.0859648855277176,0.996298167445974,0.));
#31333=DIRECTION('ref_axis',(-0.996298167445974,0.0859648855277176,0.));
#31334=DIRECTION('',(0.,0.,-1.));
#31335=DIRECTION('center_axis',(0.,0.,1.));
#31336=DIRECTION('ref_axis',(0.866025403784438,-0.5,0.));
#31337=DIRECTION('center_axis',(0.,0.,-1.));
#31338=DIRECTION('ref_axis',(1.,0.,0.));
#31339=DIRECTION('',(-0.966234513897416,0.257664246944399,0.));
#31340=DIRECTION('',(0.706261040449543,-0.707951511576272,0.));
#31341=DIRECTION('center_axis',(-0.707951511576272,-0.706261040449543,0.));
#31342=DIRECTION('ref_axis',(0.706261040449543,-0.707951511576272,0.));
#31343=DIRECTION('',(0.,0.,1.));
#31344=DIRECTION('',(0.,0.,1.));
#31345=DIRECTION('center_axis',(0.257664246944399,0.966234513897416,0.));
#31346=DIRECTION('ref_axis',(-0.966234513897416,0.257664246944399,0.));
#31347=DIRECTION('',(0.,0.,-1.));
#31348=DIRECTION('center_axis',(0.,0.,1.));
#31349=DIRECTION('ref_axis',(0.766044443118978,-0.64278760968654,0.));
#31350=DIRECTION('center_axis',(0.,0.,-1.));
#31351=DIRECTION('ref_axis',(1.,0.,0.));
#31352=DIRECTION('',(-0.906812313582341,0.421534610602074,0.));
#31353=DIRECTION('',(0.572596858423411,-0.819837079988238,0.));
#31354=DIRECTION('center_axis',(-0.819837079988238,-0.572596858423411,0.));
#31355=DIRECTION('ref_axis',(0.572596858423411,-0.819837079988238,0.));
#31356=DIRECTION('',(0.,0.,1.));
#31357=DIRECTION('',(0.,0.,1.));
#31358=DIRECTION('center_axis',(0.421534610602074,0.906812313582341,0.));
#31359=DIRECTION('ref_axis',(-0.906812313582341,0.421534610602074,0.));
#31360=DIRECTION('',(0.,0.,-1.));
#31361=DIRECTION('center_axis',(0.,0.,1.));
#31362=DIRECTION('ref_axis',(0.642787609686539,-0.766044443118978,0.));
#31363=DIRECTION('center_axis',(0.,0.,-1.));
#31364=DIRECTION('ref_axis',(1.,0.,0.));
#31365=DIRECTION('',(-0.819837079988238,0.572596858423411,0.));
#31366=DIRECTION('',(0.421534610602074,-0.906812313582341,0.));
#31367=DIRECTION('center_axis',(-0.906812313582341,-0.421534610602074,0.));
#31368=DIRECTION('ref_axis',(0.421534610602074,-0.906812313582341,0.));
#31369=DIRECTION('',(0.,0.,1.));
#31370=DIRECTION('',(0.,0.,1.));
#31371=DIRECTION('center_axis',(0.572596858423411,0.819837079988238,0.));
#31372=DIRECTION('ref_axis',(-0.819837079988238,0.572596858423411,0.));
#31373=DIRECTION('',(0.,0.,-1.));
#31374=DIRECTION('center_axis',(0.,0.,1.));
#31375=DIRECTION('ref_axis',(0.5,-0.866025403784438,0.));
#31376=DIRECTION('center_axis',(0.,0.,-1.));
#31377=DIRECTION('ref_axis',(1.,0.,0.));
#31378=DIRECTION('',(-0.707951511576272,0.706261040449544,0.));
#31379=DIRECTION('',(0.257664246944398,-0.966234513897416,0.));
#31380=DIRECTION('center_axis',(-0.966234513897416,-0.257664246944398,0.));
#31381=DIRECTION('ref_axis',(0.257664246944398,-0.966234513897416,0.));
#31382=DIRECTION('',(0.,0.,1.));
#31383=DIRECTION('',(0.,0.,1.));
#31384=DIRECTION('center_axis',(0.706261040449544,0.707951511576272,0.));
#31385=DIRECTION('ref_axis',(-0.707951511576272,0.706261040449544,0.));
#31386=DIRECTION('',(0.,0.,-1.));
#31387=DIRECTION('center_axis',(0.,0.,1.));
#31388=DIRECTION('ref_axis',(0.342020143325668,-0.939692620785909,0.));
#31389=DIRECTION('center_axis',(0.,0.,-1.));
#31390=DIRECTION('ref_axis',(1.,0.,0.));
#31391=DIRECTION('',(-0.57455519472581,0.818465838146948,0.));
#31392=DIRECTION('',(0.0859648855277162,-0.996298167445974,0.));
#31393=DIRECTION('center_axis',(-0.996298167445974,-0.0859648855277162,
0.));
#31394=DIRECTION('ref_axis',(0.0859648855277162,-0.996298167445974,0.));
#31395=DIRECTION('',(0.,0.,1.));
#31396=DIRECTION('',(0.,0.,1.));
#31397=DIRECTION('center_axis',(0.818465838146948,0.57455519472581,0.));
#31398=DIRECTION('ref_axis',(-0.57455519472581,0.818465838146948,0.));
#31399=DIRECTION('',(0.,0.,-1.));
#31400=DIRECTION('center_axis',(0.,0.,1.));
#31401=DIRECTION('ref_axis',(0.17364817766693,-0.984807753012208,0.));
#31402=DIRECTION('center_axis',(0.,0.,-1.));
#31403=DIRECTION('ref_axis',(1.,0.,0.));
#31404=DIRECTION('',(-0.423701309022563,0.905801965515955,0.));
#31405=DIRECTION('',(-0.0883464754353936,-0.996089805327885,0.));
#31406=DIRECTION('center_axis',(-0.996089805327885,0.0883464754353937,0.));
#31407=DIRECTION('ref_axis',(-0.0883464754353937,-0.996089805327885,0.));
#31408=DIRECTION('',(0.,0.,1.));
#31409=DIRECTION('',(0.,0.,1.));
#31410=DIRECTION('center_axis',(0.905801965515955,0.423701309022563,0.));
#31411=DIRECTION('ref_axis',(-0.423701309022563,0.905801965515955,0.));
#31412=DIRECTION('',(0.,0.,-1.));
#31413=DIRECTION('center_axis',(0.,0.,1.));
#31414=DIRECTION('ref_axis',(-1.94289029309402E-16,-1.,0.));
#31415=DIRECTION('center_axis',(0.,0.,-1.));
#31416=DIRECTION('ref_axis',(1.,0.,0.));
#31417=DIRECTION('',(-0.259973473447872,0.96561575852067,0.));
#31418=DIRECTION('',(-0.259973473447873,-0.96561575852067,0.));
#31419=DIRECTION('center_axis',(-0.96561575852067,0.259973473447873,0.));
#31420=DIRECTION('ref_axis',(-0.259973473447873,-0.96561575852067,0.));
#31421=DIRECTION('',(0.,0.,1.));
#31422=DIRECTION('',(0.,0.,1.));
#31423=DIRECTION('center_axis',(0.96561575852067,0.259973473447872,0.));
#31424=DIRECTION('ref_axis',(-0.259973473447872,0.96561575852067,0.));
#31425=DIRECTION('',(0.,0.,-1.));
#31426=DIRECTION('center_axis',(0.,0.,1.));
#31427=DIRECTION('ref_axis',(-0.17364817766693,-0.984807753012208,0.));
#31428=DIRECTION('center_axis',(0.,0.,-1.));
#31429=DIRECTION('ref_axis',(1.,0.,0.));
#31430=DIRECTION('',(-0.0883464754353933,0.996089805327885,0.));
#31431=DIRECTION('',(-0.423701309022563,-0.905801965515955,0.));
#31432=DIRECTION('center_axis',(-0.905801965515955,0.423701309022563,0.));
#31433=DIRECTION('ref_axis',(-0.423701309022563,-0.905801965515955,0.));
#31434=DIRECTION('',(0.,0.,1.));
#31435=DIRECTION('',(0.,0.,1.));
#31436=DIRECTION('center_axis',(0.996089805327885,0.0883464754353932,0.));
#31437=DIRECTION('ref_axis',(-0.0883464754353932,0.996089805327885,0.));
#31438=DIRECTION('',(0.,0.,-1.));
#31439=DIRECTION('center_axis',(0.,0.,1.));
#31440=DIRECTION('ref_axis',(-0.342020143325669,-0.939692620785908,0.));
#31441=DIRECTION('center_axis',(0.,0.,-1.));
#31442=DIRECTION('ref_axis',(1.,0.,0.));
#31443=DIRECTION('',(0.0859648855277175,0.996298167445974,0.));
#31444=DIRECTION('',(-0.574555194725811,-0.818465838146947,0.));
#31445=DIRECTION('center_axis',(-0.818465838146947,0.574555194725811,0.));
#31446=DIRECTION('ref_axis',(-0.574555194725811,-0.818465838146947,0.));
#31447=DIRECTION('',(0.,0.,1.));
#31448=DIRECTION('',(0.,0.,1.));
#31449=DIRECTION('center_axis',(0.996298167445974,-0.0859648855277175,0.));
#31450=DIRECTION('ref_axis',(0.0859648855277175,0.996298167445974,0.));
#31451=DIRECTION('',(0.,0.,-1.));
#31452=DIRECTION('center_axis',(0.,0.,1.));
#31453=DIRECTION('ref_axis',(-0.5,-0.866025403784438,0.));
#31454=DIRECTION('center_axis',(0.,0.,-1.));
#31455=DIRECTION('ref_axis',(1.,0.,0.));
#31456=DIRECTION('',(0.257664246944399,0.966234513897416,0.));
#31457=DIRECTION('',(-0.707951511576272,-0.706261040449543,0.));
#31458=DIRECTION('center_axis',(-0.706261040449543,0.707951511576272,0.));
#31459=DIRECTION('ref_axis',(-0.707951511576272,-0.706261040449543,0.));
#31460=DIRECTION('',(0.,0.,1.));
#31461=DIRECTION('',(0.,0.,1.));
#31462=DIRECTION('center_axis',(0.966234513897416,-0.257664246944399,0.));
#31463=DIRECTION('ref_axis',(0.257664246944399,0.966234513897416,0.));
#31464=DIRECTION('',(0.,0.,-1.));
#31465=DIRECTION('center_axis',(0.,0.,1.));
#31466=DIRECTION('ref_axis',(-0.642787609686539,-0.766044443118978,0.));
#31467=DIRECTION('center_axis',(0.,0.,-1.));
#31468=DIRECTION('ref_axis',(1.,0.,0.));
#31469=DIRECTION('',(0.421534610602074,0.906812313582341,0.));
#31470=DIRECTION('',(-0.819837079988238,-0.572596858423411,0.));
#31471=DIRECTION('center_axis',(-0.572596858423411,0.819837079988238,0.));
#31472=DIRECTION('ref_axis',(-0.819837079988238,-0.572596858423411,0.));
#31473=DIRECTION('',(0.,0.,1.));
#31474=DIRECTION('',(0.,0.,1.));
#31475=DIRECTION('center_axis',(0.906812313582341,-0.421534610602074,0.));
#31476=DIRECTION('ref_axis',(0.421534610602074,0.906812313582341,0.));
#31477=DIRECTION('',(0.,0.,-1.));
#31478=DIRECTION('center_axis',(0.,0.,1.));
#31479=DIRECTION('ref_axis',(-0.766044443118978,-0.642787609686539,0.));
#31480=DIRECTION('center_axis',(0.,0.,-1.));
#31481=DIRECTION('ref_axis',(1.,0.,0.));
#31482=DIRECTION('',(0.572596858423411,0.819837079988238,0.));
#31483=DIRECTION('',(-0.906812313582341,-0.421534610602074,0.));
#31484=DIRECTION('center_axis',(-0.421534610602074,0.906812313582341,0.));
#31485=DIRECTION('ref_axis',(-0.906812313582341,-0.421534610602074,0.));
#31486=DIRECTION('',(0.,0.,1.));
#31487=DIRECTION('',(0.,0.,1.));
#31488=DIRECTION('center_axis',(0.819837079988238,-0.572596858423411,0.));
#31489=DIRECTION('ref_axis',(0.572596858423411,0.819837079988238,0.));
#31490=DIRECTION('',(0.,0.,-1.));
#31491=DIRECTION('center_axis',(0.,0.,1.));
#31492=DIRECTION('ref_axis',(-0.866025403784439,-0.5,0.));
#31493=DIRECTION('center_axis',(0.,0.,-1.));
#31494=DIRECTION('ref_axis',(1.,0.,0.));
#31495=DIRECTION('',(0.706261040449544,0.707951511576271,0.));
#31496=DIRECTION('',(-0.966234513897416,-0.257664246944398,0.));
#31497=DIRECTION('center_axis',(-0.257664246944398,0.966234513897416,0.));
#31498=DIRECTION('ref_axis',(-0.966234513897416,-0.257664246944398,0.));
#31499=DIRECTION('',(0.,0.,1.));
#31500=DIRECTION('',(0.,0.,1.));
#31501=DIRECTION('center_axis',(0.707951511576271,-0.706261040449544,0.));
#31502=DIRECTION('ref_axis',(0.706261040449544,0.707951511576271,0.));
#31503=DIRECTION('',(0.,0.,-1.));
#31504=DIRECTION('center_axis',(0.,0.,1.));
#31505=DIRECTION('ref_axis',(-0.939692620785909,-0.342020143325669,0.));
#31506=DIRECTION('center_axis',(0.,0.,-1.));
#31507=DIRECTION('ref_axis',(1.,0.,0.));
#31508=DIRECTION('',(0.818465838146948,0.574555194725811,0.));
#31509=DIRECTION('',(-0.996298167445974,-0.0859648855277167,0.));
#31510=DIRECTION('center_axis',(-0.0859648855277167,0.996298167445974,0.));
#31511=DIRECTION('ref_axis',(-0.996298167445974,-0.0859648855277167,0.));
#31512=DIRECTION('',(0.,0.,1.));
#31513=DIRECTION('',(0.,0.,1.));
#31514=DIRECTION('center_axis',(0.574555194725811,-0.818465838146948,0.));
#31515=DIRECTION('ref_axis',(0.818465838146948,0.574555194725811,0.));
#31516=DIRECTION('',(0.,0.,-1.));
#31517=DIRECTION('center_axis',(0.,0.,1.));
#31518=DIRECTION('ref_axis',(-0.984807753012208,-0.17364817766693,0.));
#31519=DIRECTION('center_axis',(0.,0.,-1.));
#31520=DIRECTION('ref_axis',(1.,0.,0.));
#31521=DIRECTION('',(0.905801965515955,0.423701309022563,0.));
#31522=DIRECTION('',(-0.996089805327885,0.0883464754353936,0.));
#31523=DIRECTION('center_axis',(0.0883464754353936,0.996089805327885,0.));
#31524=DIRECTION('ref_axis',(-0.996089805327885,0.0883464754353936,0.));
#31525=DIRECTION('',(0.,0.,1.));
#31526=DIRECTION('',(0.,0.,1.));
#31527=DIRECTION('center_axis',(0.423701309022563,-0.905801965515955,0.));
#31528=DIRECTION('ref_axis',(0.905801965515955,0.423701309022563,0.));
#31529=DIRECTION('',(0.,0.,-1.));
#31530=DIRECTION('center_axis',(0.,0.,1.));
#31531=DIRECTION('ref_axis',(-1.,1.11022302462516E-16,0.));
#31532=DIRECTION('center_axis',(0.,0.,-1.));
#31533=DIRECTION('ref_axis',(1.,0.,0.));
#31534=DIRECTION('',(0.96561575852067,0.259973473447872,0.));
#31535=DIRECTION('',(-0.96561575852067,0.259973473447873,0.));
#31536=DIRECTION('center_axis',(0.,0.,-1.));
#31537=DIRECTION('ref_axis',(1.,0.,0.));
#31538=DIRECTION('center_axis',(0.259973473447873,0.96561575852067,0.));
#31539=DIRECTION('ref_axis',(-0.96561575852067,0.259973473447873,0.));
#31540=DIRECTION('',(0.,0.,1.));
#31541=DIRECTION('',(0.,0.,1.));
#31542=DIRECTION('center_axis',(0.259973473447872,-0.96561575852067,0.));
#31543=DIRECTION('ref_axis',(0.96561575852067,0.259973473447872,0.));
#31544=DIRECTION('',(0.,0.,-1.));
#31545=DIRECTION('center_axis',(0.,0.,1.));
#31546=DIRECTION('ref_axis',(-0.984807753012208,0.173648177666931,0.));
#31547=DIRECTION('center_axis',(0.,0.,-1.));
#31548=DIRECTION('ref_axis',(1.,0.,0.));
#31549=DIRECTION('',(0.996089805327885,0.0883464754353928,0.));
#31550=DIRECTION('',(-0.905801965515954,0.423701309022564,0.));
#31551=DIRECTION('center_axis',(0.423701309022564,0.905801965515954,0.));
#31552=DIRECTION('ref_axis',(-0.905801965515954,0.423701309022564,0.));
#31553=DIRECTION('',(0.,0.,1.));
#31554=DIRECTION('',(0.,0.,1.));
#31555=DIRECTION('center_axis',(0.0883464754353928,-0.996089805327885,0.));
#31556=DIRECTION('ref_axis',(0.996089805327885,0.0883464754353928,0.));
#31557=DIRECTION('',(0.,0.,-1.));
#31558=DIRECTION('center_axis',(0.,0.,1.));
#31559=DIRECTION('ref_axis',(-0.939692620785908,0.342020143325669,0.));
#31560=DIRECTION('center_axis',(0.,0.,-1.));
#31561=DIRECTION('ref_axis',(1.,0.,0.));
#31562=DIRECTION('',(0.996298167445974,-0.085964885527717,0.));
#31563=DIRECTION('',(-0.818465838146948,0.574555194725811,0.));
#31564=DIRECTION('center_axis',(0.574555194725811,0.818465838146948,0.));
#31565=DIRECTION('ref_axis',(-0.818465838146948,0.574555194725811,0.));
#31566=DIRECTION('',(0.,0.,1.));
#31567=DIRECTION('',(0.,0.,1.));
#31568=DIRECTION('center_axis',(-0.085964885527717,-0.996298167445974,0.));
#31569=DIRECTION('ref_axis',(0.996298167445974,-0.085964885527717,0.));
#31570=DIRECTION('',(0.,0.,-1.));
#31571=DIRECTION('center_axis',(0.,0.,1.));
#31572=DIRECTION('ref_axis',(-0.866025403784439,0.5,0.));
#31573=DIRECTION('center_axis',(0.,0.,-1.));
#31574=DIRECTION('ref_axis',(1.,0.,0.));
#31575=DIRECTION('',(0.966234513897416,-0.257664246944398,0.));
#31576=DIRECTION('',(-0.706261040449544,0.707951511576272,0.));
#31577=DIRECTION('center_axis',(0.707951511576272,0.706261040449544,0.));
#31578=DIRECTION('ref_axis',(-0.706261040449544,0.707951511576272,0.));
#31579=DIRECTION('',(0.,0.,1.));
#31580=DIRECTION('',(0.,0.,1.));
#31581=DIRECTION('center_axis',(-0.257664246944398,-0.966234513897416,0.));
#31582=DIRECTION('ref_axis',(0.966234513897416,-0.257664246944398,0.));
#31583=DIRECTION('',(0.,0.,-1.));
#31584=DIRECTION('center_axis',(0.,0.,1.));
#31585=DIRECTION('ref_axis',(-0.766044443118978,0.642787609686539,0.));
#31586=DIRECTION('center_axis',(0.,0.,-1.));
#31587=DIRECTION('ref_axis',(1.,0.,0.));
#31588=DIRECTION('',(0.906812313582341,-0.421534610602074,0.));
#31589=DIRECTION('',(-0.572596858423411,0.819837079988238,0.));
#31590=DIRECTION('center_axis',(0.819837079988238,0.572596858423411,0.));
#31591=DIRECTION('ref_axis',(-0.572596858423411,0.819837079988238,0.));
#31592=DIRECTION('',(0.,0.,1.));
#31593=DIRECTION('',(0.,0.,1.));
#31594=DIRECTION('center_axis',(-0.421534610602074,-0.906812313582341,0.));
#31595=DIRECTION('ref_axis',(0.906812313582341,-0.421534610602074,0.));
#31596=DIRECTION('',(0.,0.,-1.));
#31597=DIRECTION('center_axis',(0.,0.,1.));
#31598=DIRECTION('ref_axis',(-0.642787609686539,0.766044443118978,0.));
#31599=DIRECTION('center_axis',(0.,0.,-1.));
#31600=DIRECTION('ref_axis',(1.,0.,0.));
#31601=DIRECTION('',(0.819837079988238,-0.572596858423411,0.));
#31602=DIRECTION('',(-0.421534610602074,0.906812313582341,0.));
#31603=DIRECTION('center_axis',(0.906812313582341,0.421534610602074,0.));
#31604=DIRECTION('ref_axis',(-0.421534610602074,0.906812313582341,0.));
#31605=DIRECTION('',(0.,0.,1.));
#31606=DIRECTION('',(0.,0.,1.));
#31607=DIRECTION('center_axis',(-0.572596858423411,-0.819837079988238,0.));
#31608=DIRECTION('ref_axis',(0.819837079988238,-0.572596858423411,0.));
#31609=DIRECTION('',(0.,0.,-1.));
#31610=DIRECTION('center_axis',(0.,0.,1.));
#31611=DIRECTION('ref_axis',(-0.5,0.866025403784439,0.));
#31612=DIRECTION('center_axis',(0.,0.,-1.));
#31613=DIRECTION('ref_axis',(1.,0.,0.));
#31614=DIRECTION('',(0.707951511576272,-0.706261040449544,0.));
#31615=DIRECTION('',(-0.257664246944398,0.966234513897416,0.));
#31616=DIRECTION('center_axis',(0.966234513897416,0.257664246944398,0.));
#31617=DIRECTION('ref_axis',(-0.257664246944398,0.966234513897416,0.));
#31618=DIRECTION('',(0.,0.,1.));
#31619=DIRECTION('',(0.,0.,1.));
#31620=DIRECTION('center_axis',(-0.706261040449544,-0.707951511576272,0.));
#31621=DIRECTION('ref_axis',(0.707951511576272,-0.706261040449544,0.));
#31622=DIRECTION('',(0.,0.,-1.));
#31623=DIRECTION('center_axis',(0.,0.,1.));
#31624=DIRECTION('ref_axis',(-0.342020143325669,0.939692620785909,0.));
#31625=DIRECTION('center_axis',(0.,0.,-1.));
#31626=DIRECTION('ref_axis',(1.,0.,0.));
#31627=DIRECTION('',(0.574555194725811,-0.818465838146948,0.));
#31628=DIRECTION('',(-0.0859648855277167,0.996298167445974,0.));
#31629=DIRECTION('center_axis',(0.996298167445974,0.0859648855277167,0.));
#31630=DIRECTION('ref_axis',(-0.0859648855277167,0.996298167445974,0.));
#31631=DIRECTION('',(0.,0.,1.));
#31632=DIRECTION('',(0.,0.,1.));
#31633=DIRECTION('center_axis',(-0.818465838146948,-0.574555194725811,0.));
#31634=DIRECTION('ref_axis',(0.574555194725811,-0.818465838146948,0.));
#31635=DIRECTION('',(0.,0.,-1.));
#31636=DIRECTION('center_axis',(0.,0.,1.));
#31637=DIRECTION('ref_axis',(-0.17364817766693,0.984807753012208,0.));
#31638=DIRECTION('center_axis',(0.,0.,-1.));
#31639=DIRECTION('ref_axis',(1.,0.,0.));
#31640=DIRECTION('',(0.423701309022563,-0.905801965515955,0.));
#31641=DIRECTION('',(0.0883464754353932,0.996089805327885,0.));
#31642=DIRECTION('center_axis',(0.996089805327885,-0.0883464754353932,0.));
#31643=DIRECTION('ref_axis',(0.0883464754353932,0.996089805327885,0.));
#31644=DIRECTION('',(0.,0.,1.));
#31645=DIRECTION('',(0.,0.,1.));
#31646=DIRECTION('center_axis',(-0.905801965515955,-0.423701309022563,0.));
#31647=DIRECTION('ref_axis',(0.423701309022563,-0.905801965515955,0.));
#31648=DIRECTION('',(0.,0.,-1.));
#31649=DIRECTION('center_axis',(0.,0.,1.));
#31650=DIRECTION('ref_axis',(5.55111512312578E-17,1.,0.));
#31651=DIRECTION('center_axis',(0.,0.,-1.));
#31652=DIRECTION('ref_axis',(1.,0.,0.));
#31653=DIRECTION('',(0.259973473447872,-0.96561575852067,0.));
#31654=DIRECTION('',(0.259973473447872,0.96561575852067,0.));
#31655=DIRECTION('center_axis',(0.96561575852067,-0.259973473447873,0.));
#31656=DIRECTION('ref_axis',(0.259973473447873,0.96561575852067,0.));
#31657=DIRECTION('',(0.,0.,1.));
#31658=DIRECTION('',(0.,0.,1.));
#31659=DIRECTION('center_axis',(-0.96561575852067,-0.259973473447872,0.));
#31660=DIRECTION('ref_axis',(0.259973473447872,-0.96561575852067,0.));
#31661=DIRECTION('',(0.,0.,-1.));
#31662=DIRECTION('center_axis',(0.,0.,1.));
#31663=DIRECTION('ref_axis',(0.17364817766693,0.984807753012208,0.));
#31664=DIRECTION('center_axis',(0.,0.,-1.));
#31665=DIRECTION('ref_axis',(1.,0.,0.));
#31666=DIRECTION('',(0.0883464754353931,-0.996089805327885,0.));
#31667=DIRECTION('',(0.423701309022563,0.905801965515954,0.));
#31668=DIRECTION('center_axis',(0.905801965515954,-0.423701309022563,0.));
#31669=DIRECTION('ref_axis',(0.423701309022563,0.905801965515954,0.));
#31670=DIRECTION('',(0.,0.,1.));
#31671=DIRECTION('',(0.,0.,1.));
#31672=DIRECTION('center_axis',(-0.996089805327885,-0.0883464754353932,
0.));
#31673=DIRECTION('ref_axis',(0.0883464754353932,-0.996089805327885,0.));
#31674=DIRECTION('',(0.,0.,-1.));
#31675=DIRECTION('center_axis',(0.,0.,1.));
#31676=DIRECTION('ref_axis',(0.342020143325669,0.939692620785908,0.));
#31677=DIRECTION('center_axis',(0.,0.,-1.));
#31678=DIRECTION('ref_axis',(1.,0.,0.));
#31679=DIRECTION('',(-0.085964885527717,-0.996298167445974,0.));
#31680=DIRECTION('',(0.574555194725811,0.818465838146948,0.));
#31681=DIRECTION('center_axis',(0.818465838146948,-0.574555194725811,0.));
#31682=DIRECTION('ref_axis',(0.574555194725811,0.818465838146948,0.));
#31683=DIRECTION('',(0.,0.,1.));
#31684=DIRECTION('',(0.,0.,1.));
#31685=DIRECTION('center_axis',(-0.996298167445974,0.085964885527717,0.));
#31686=DIRECTION('ref_axis',(-0.085964885527717,-0.996298167445974,0.));
#31687=DIRECTION('',(0.,0.,-1.));
#31688=DIRECTION('center_axis',(0.,0.,1.));
#31689=DIRECTION('ref_axis',(0.5,0.866025403784439,0.));
#31690=DIRECTION('center_axis',(0.,0.,-1.));
#31691=DIRECTION('ref_axis',(1.,0.,0.));
#31692=DIRECTION('',(-0.257664246944398,-0.966234513897416,0.));
#31693=DIRECTION('',(0.707951511576272,0.706261040449544,0.));
#31694=DIRECTION('center_axis',(0.706261040449544,-0.707951511576272,0.));
#31695=DIRECTION('ref_axis',(0.707951511576272,0.706261040449544,0.));
#31696=DIRECTION('',(0.,0.,1.));
#31697=DIRECTION('',(0.,0.,1.));
#31698=DIRECTION('center_axis',(-0.966234513897416,0.257664246944398,0.));
#31699=DIRECTION('ref_axis',(-0.257664246944398,-0.966234513897416,0.));
#31700=DIRECTION('',(0.,0.,-1.));
#31701=DIRECTION('center_axis',(0.,0.,1.));
#31702=DIRECTION('ref_axis',(0.642787609686539,0.766044443118978,0.));
#31703=DIRECTION('center_axis',(0.,0.,-1.));
#31704=DIRECTION('ref_axis',(1.,0.,0.));
#31705=DIRECTION('',(-0.421534610602074,-0.906812313582341,0.));
#31706=DIRECTION('',(0.819837079988238,0.572596858423411,0.));
#31707=DIRECTION('center_axis',(0.572596858423411,-0.819837079988238,0.));
#31708=DIRECTION('ref_axis',(0.819837079988238,0.572596858423411,0.));
#31709=DIRECTION('',(0.,0.,1.));
#31710=DIRECTION('',(0.,0.,1.));
#31711=DIRECTION('center_axis',(-0.906812313582341,0.421534610602074,0.));
#31712=DIRECTION('ref_axis',(-0.421534610602074,-0.906812313582341,0.));
#31713=DIRECTION('',(0.,0.,-1.));
#31714=DIRECTION('center_axis',(0.,0.,1.));
#31715=DIRECTION('ref_axis',(0.766044443118978,0.642787609686539,0.));
#31716=DIRECTION('center_axis',(0.,0.,-1.));
#31717=DIRECTION('ref_axis',(1.,0.,0.));
#31718=DIRECTION('',(-0.572596858423411,-0.819837079988238,0.));
#31719=DIRECTION('',(0.906812313582341,0.421534610602074,0.));
#31720=DIRECTION('center_axis',(0.421534610602074,-0.906812313582341,0.));
#31721=DIRECTION('ref_axis',(0.906812313582341,0.421534610602074,0.));
#31722=DIRECTION('',(0.,0.,1.));
#31723=DIRECTION('',(0.,0.,1.));
#31724=DIRECTION('center_axis',(-0.819837079988238,0.572596858423411,0.));
#31725=DIRECTION('ref_axis',(-0.572596858423411,-0.819837079988238,0.));
#31726=DIRECTION('',(0.,0.,-1.));
#31727=DIRECTION('center_axis',(0.,0.,1.));
#31728=DIRECTION('ref_axis',(0.866025403784439,0.5,0.));
#31729=DIRECTION('center_axis',(0.,0.,-1.));
#31730=DIRECTION('ref_axis',(1.,0.,0.));
#31731=DIRECTION('',(-0.706261040449544,-0.707951511576272,0.));
#31732=DIRECTION('',(0.966234513897416,0.257664246944398,0.));
#31733=DIRECTION('center_axis',(0.257664246944398,-0.966234513897416,0.));
#31734=DIRECTION('ref_axis',(0.966234513897416,0.257664246944398,0.));
#31735=DIRECTION('',(0.,0.,1.));
#31736=DIRECTION('',(0.,0.,1.));
#31737=DIRECTION('center_axis',(-0.707951511576272,0.706261040449544,0.));
#31738=DIRECTION('ref_axis',(-0.706261040449544,-0.707951511576272,0.));
#31739=DIRECTION('',(0.,0.,-1.));
#31740=DIRECTION('center_axis',(0.,0.,1.));
#31741=DIRECTION('ref_axis',(0.939692620785909,0.342020143325669,0.));
#31742=DIRECTION('center_axis',(0.,0.,-1.));
#31743=DIRECTION('ref_axis',(1.,0.,0.));
#31744=DIRECTION('',(-0.818465838146948,-0.574555194725811,0.));
#31745=DIRECTION('',(0.996298167445974,0.0859648855277167,0.));
#31746=DIRECTION('center_axis',(0.0859648855277167,-0.996298167445974,0.));
#31747=DIRECTION('ref_axis',(0.996298167445974,0.0859648855277167,0.));
#31748=DIRECTION('',(0.,0.,1.));
#31749=DIRECTION('',(0.,0.,1.));
#31750=DIRECTION('center_axis',(-0.574555194725811,0.818465838146948,0.));
#31751=DIRECTION('ref_axis',(-0.818465838146948,-0.574555194725811,0.));
#31752=DIRECTION('',(0.,0.,-1.));
#31753=DIRECTION('center_axis',(0.,0.,1.));
#31754=DIRECTION('ref_axis',(0.984807753012208,0.17364817766693,0.));
#31755=DIRECTION('center_axis',(0.,0.,-1.));
#31756=DIRECTION('ref_axis',(1.,0.,0.));
#31757=DIRECTION('',(-0.905801965515955,-0.423701309022563,0.));
#31758=DIRECTION('',(0.996089805327885,-0.0883464754353932,0.));
#31759=DIRECTION('center_axis',(-0.0883464754353933,-0.996089805327885,
0.));
#31760=DIRECTION('ref_axis',(0.996089805327885,-0.0883464754353933,0.));
#31761=DIRECTION('',(0.,0.,1.));
#31762=DIRECTION('',(0.,0.,1.));
#31763=DIRECTION('center_axis',(-0.423701309022563,0.905801965515955,0.));
#31764=DIRECTION('ref_axis',(-0.905801965515954,-0.423701309022563,0.));
#31765=DIRECTION('',(0.,0.,-1.));
#31766=DIRECTION('center_axis',(0.,0.,1.));
#31767=DIRECTION('ref_axis',(1.,0.,0.));
#31768=DIRECTION('center_axis',(0.,0.,1.));
#31769=DIRECTION('ref_axis',(1.,0.,0.));
#31770=DIRECTION('center_axis',(0.,0.,1.));
#31771=DIRECTION('ref_axis',(1.,0.,0.));
#31772=DIRECTION('center_axis',(0.,0.,1.));
#31773=DIRECTION('ref_axis',(1.,0.,0.));
#31774=DIRECTION('center_axis',(0.,0.,1.));
#31775=DIRECTION('ref_axis',(1.,0.,0.));
#31776=DIRECTION('center_axis',(0.,0.,1.));
#31777=DIRECTION('ref_axis',(1.,0.,0.));
#31778=DIRECTION('center_axis',(0.,0.,1.));
#31779=DIRECTION('ref_axis',(1.,0.,0.));
#31780=DIRECTION('center_axis',(0.,0.,1.));
#31781=DIRECTION('ref_axis',(1.,0.,0.));
#31782=DIRECTION('center_axis',(0.,0.,1.));
#31783=DIRECTION('ref_axis',(1.,0.,0.));
#31784=DIRECTION('center_axis',(0.,0.,1.));
#31785=DIRECTION('ref_axis',(1.,0.,0.));
#31786=DIRECTION('center_axis',(0.,0.,1.));
#31787=DIRECTION('ref_axis',(1.,0.,0.));
#31788=DIRECTION('center_axis',(0.,0.,1.));
#31789=DIRECTION('ref_axis',(1.,0.,0.));
#31790=DIRECTION('center_axis',(0.,0.,1.));
#31791=DIRECTION('ref_axis',(1.,0.,0.));
#31792=DIRECTION('center_axis',(0.,0.,1.));
#31793=DIRECTION('ref_axis',(1.,0.,0.));
#31794=DIRECTION('center_axis',(0.,0.,1.));
#31795=DIRECTION('ref_axis',(1.,0.,0.));
#31796=DIRECTION('center_axis',(0.,0.,1.));
#31797=DIRECTION('ref_axis',(1.,0.,0.));
#31798=DIRECTION('center_axis',(0.,0.,1.));
#31799=DIRECTION('ref_axis',(1.,0.,0.));
#31800=DIRECTION('center_axis',(0.,0.,1.));
#31801=DIRECTION('ref_axis',(1.,0.,0.));
#31802=DIRECTION('',(0.,0.,-1.));
#31803=DIRECTION('center_axis',(0.,0.,1.));
#31804=DIRECTION('ref_axis',(1.,0.,0.));
#31805=DIRECTION('center_axis',(0.,0.,1.));
#31806=DIRECTION('ref_axis',(1.,0.,0.));
#31807=DIRECTION('center_axis',(0.,0.,1.));
#31808=DIRECTION('ref_axis',(1.,0.,0.));
#31809=DIRECTION('center_axis',(0.,0.,1.));
#31810=DIRECTION('ref_axis',(1.,0.,0.));
#31811=DIRECTION('center_axis',(0.,0.,1.));
#31812=DIRECTION('ref_axis',(1.,0.,0.));
#31813=DIRECTION('center_axis',(0.,0.,1.));
#31814=DIRECTION('ref_axis',(1.,0.,0.));
#31815=DIRECTION('center_axis',(0.,0.,1.));
#31816=DIRECTION('ref_axis',(1.,0.,0.));
#31817=DIRECTION('center_axis',(0.,0.,1.));
#31818=DIRECTION('ref_axis',(1.,0.,0.));
#31819=DIRECTION('center_axis',(0.,0.,1.));
#31820=DIRECTION('ref_axis',(1.,0.,0.));
#31821=DIRECTION('center_axis',(0.,0.,1.));
#31822=DIRECTION('ref_axis',(1.,0.,0.));
#31823=DIRECTION('center_axis',(0.,0.,1.));
#31824=DIRECTION('ref_axis',(1.,0.,0.));
#31825=DIRECTION('center_axis',(0.,0.,1.));
#31826=DIRECTION('ref_axis',(1.,0.,0.));
#31827=DIRECTION('center_axis',(0.,0.,1.));
#31828=DIRECTION('ref_axis',(1.,0.,0.));
#31829=DIRECTION('center_axis',(0.,0.,1.));
#31830=DIRECTION('ref_axis',(1.,0.,0.));
#31831=DIRECTION('center_axis',(0.,0.,1.));
#31832=DIRECTION('ref_axis',(1.,0.,0.));
#31833=DIRECTION('center_axis',(0.,0.,1.));
#31834=DIRECTION('ref_axis',(1.,0.,0.));
#31835=DIRECTION('center_axis',(0.,0.,1.));
#31836=DIRECTION('ref_axis',(1.,0.,0.));
#31837=DIRECTION('center_axis',(0.,0.,1.));
#31838=DIRECTION('ref_axis',(1.,0.,0.));
#31839=DIRECTION('center_axis',(0.,0.,1.));
#31840=DIRECTION('ref_axis',(1.,0.,0.));
#31841=DIRECTION('',(0.,0.,-1.));
#31842=DIRECTION('center_axis',(0.,0.,-1.));
#31843=DIRECTION('ref_axis',(1.,0.,0.));
#31844=DIRECTION('',(0.,0.,1.));
#31845=DIRECTION('center_axis',(0.,0.,1.));
#31846=DIRECTION('ref_axis',(1.,0.,0.));
#31847=DIRECTION('center_axis',(-0.259973473447872,-0.96561575852067,0.));
#31848=DIRECTION('ref_axis',(0.96561575852067,-0.259973473447872,0.));
#31849=DIRECTION('',(0.96561575852067,-0.259973473447872,0.));
#31850=DIRECTION('',(0.,0.,1.));
#31851=DIRECTION('center_axis',(-0.259973473447872,0.96561575852067,0.));
#31852=DIRECTION('ref_axis',(-0.96561575852067,-0.259973473447872,0.));
#31853=DIRECTION('',(-0.96561575852067,-0.259973473447872,0.));
#31854=DIRECTION('center_axis',(0.,0.,1.));
#31855=DIRECTION('ref_axis',(1.,0.,0.));
#31856=DIRECTION('center_axis',(0.,0.,-1.));
#31857=DIRECTION('ref_axis',(1.,0.,0.));
#31858=DIRECTION('center_axis',(0.,0.,1.));
#31859=DIRECTION('ref_axis',(1.,0.,0.));
#31860=DIRECTION('',(-0.707106781186548,-8.65956056235493E-17,-0.707106781186548));
#31861=DIRECTION('center_axis',(0.,0.,1.));
#31862=DIRECTION('ref_axis',(1.,0.,0.));
#31863=DIRECTION('',(-0.842487928864452,-1.03175014540413E-16,0.538715221353255));
#31864=DIRECTION('center_axis',(0.,0.,-1.));
#31865=DIRECTION('ref_axis',(1.,0.,0.));
#31866=DIRECTION('center_axis',(0.5,0.866025403784439,0.));
#31867=DIRECTION('ref_axis',(0.866025403784439,-0.5,0.));
#31868=DIRECTION('',(0.866025403784439,-0.5,0.));
#31869=DIRECTION('',(0.,0.,-1.));
#31870=DIRECTION('',(0.866025403784439,-0.5,0.));
#31871=DIRECTION('',(0.,0.,-1.));
#31872=DIRECTION('center_axis',(-0.5,0.866025403784439,0.));
#31873=DIRECTION('ref_axis',(0.866025403784439,0.5,0.));
#31874=DIRECTION('',(0.866025403784439,0.5,0.));
#31875=DIRECTION('',(0.,0.,-1.));
#31876=DIRECTION('',(0.866025403784439,0.5,0.));
#31877=DIRECTION('center_axis',(-1.,-1.60246890531964E-16,0.));
#31878=DIRECTION('ref_axis',(-1.60246890531964E-16,1.,0.));
#31879=DIRECTION('',(-1.60246890531964E-16,1.,0.));
#31880=DIRECTION('',(0.,0.,-1.));
#31881=DIRECTION('',(-1.60246890531964E-16,1.,0.));
#31882=DIRECTION('center_axis',(-0.5,-0.866025403784439,0.));
#31883=DIRECTION('ref_axis',(-0.866025403784439,0.5,0.));
#31884=DIRECTION('',(-0.866025403784439,0.5,0.));
#31885=DIRECTION('',(0.,0.,-1.));
#31886=DIRECTION('',(-0.866025403784439,0.5,0.));
#31887=DIRECTION('center_axis',(0.5,-0.866025403784439,0.));
#31888=DIRECTION('ref_axis',(-0.866025403784439,-0.5,0.));
#31889=DIRECTION('',(-0.866025403784439,-0.5,0.));
#31890=DIRECTION('',(0.,0.,-1.));
#31891=DIRECTION('',(-0.866025403784439,-0.5,0.));
#31892=DIRECTION('center_axis',(1.,-3.20493781063927E-16,0.));
#31893=DIRECTION('ref_axis',(-3.20493781063927E-16,-1.,0.));
#31894=DIRECTION('',(-3.20493781063927E-16,-1.,0.));
#31895=DIRECTION('',(-3.20493781063927E-16,-1.,0.));
#31896=DIRECTION('center_axis',(0.,0.,-1.));
#31897=DIRECTION('ref_axis',(-1.,0.,0.));
#31898=DIRECTION('center_axis',(0.,0.,-1.));
#31899=DIRECTION('ref_axis',(-1.,0.,0.));
#31900=DIRECTION('center_axis',(0.,0.,1.));
#31901=DIRECTION('ref_axis',(1.,0.,0.));
#31902=DIRECTION('center_axis',(0.,0.,1.));
#31903=DIRECTION('ref_axis',(1.,0.,0.));
#31904=DIRECTION('',(0.707106781186547,8.65956056235493E-17,-0.707106781186548));
#31905=DIRECTION('center_axis',(0.,0.,1.));
#31906=DIRECTION('ref_axis',(1.,0.,0.));
#31907=DIRECTION('center_axis',(0.,0.,1.));
#31908=DIRECTION('ref_axis',(1.,0.,0.));
#31909=DIRECTION('center_axis',(0.,0.,1.));
#31910=DIRECTION('ref_axis',(1.,0.,0.));
#31911=DIRECTION('center_axis',(0.,0.,1.));
#31912=DIRECTION('ref_axis',(1.,0.,0.));
#31913=DIRECTION('',(0.707106781186548,8.65956056235494E-17,-0.707106781186547));
#31914=DIRECTION('center_axis',(0.,0.,-1.));
#31915=DIRECTION('ref_axis',(-1.,0.,0.));
#31916=DIRECTION('center_axis',(0.,0.,1.));
#31917=DIRECTION('ref_axis',(1.,0.,0.));
#39974=CARTESIAN_POINT('',(0.,0.,0.));
#39975=CARTESIAN_POINT('Origin',(0.,0.,-0.593));
#39976=CARTESIAN_POINT('',(-0.0965944740297558,-7.73963603528036E-5,-1.12642640831103));
#39977=CARTESIAN_POINT('',(-0.096611016528836,-7.98840753066898E-5,-1.13222359168897));
#39978=CARTESIAN_POINT('',(-0.096675,-1.1839272930757E-17,-0.593));
#39979=CARTESIAN_POINT('',(0.0869541681035032,-0.0426122506771691,-1.149325));
#39980=CARTESIAN_POINT('Ctrl Pts',(-0.0965944740297558,-7.73963603528036E-5,
-1.12642640831103));
#39981=CARTESIAN_POINT('Ctrl Pts',(-0.0964320926110229,0.0217456623633545,
-1.12786083909321));
#39982=CARTESIAN_POINT('Ctrl Pts',(-0.0891113319759391,0.0436686423674009,
-1.12929526987539));
#39983=CARTESIAN_POINT('Ctrl Pts',(-0.0755433113465464,0.0605838294610271,
-1.13072970065757));
#39984=CARTESIAN_POINT('Ctrl Pts',(-0.0555256438879884,0.0855397607267844,
-1.13284599743912));
#39985=CARTESIAN_POINT('Ctrl Pts',(-0.0219097104812664,0.0995953453011509,
-1.13496229422066));
#39986=CARTESIAN_POINT('Ctrl Pts',(0.00990845972240706,0.0963245926632457,
-1.13707859100221));
#39987=CARTESIAN_POINT('Ctrl Pts',(0.0417266299260805,0.0930538400253404,
-1.13919488778376));
#39988=CARTESIAN_POINT('Ctrl Pts',(0.0717470369267054,0.0724567501751636,
-1.14131118456531));
#39989=CARTESIAN_POINT('Ctrl Pts',(0.0862756370450348,0.0439486032544623,
-1.14342748134686));
#39990=CARTESIAN_POINT('Ctrl Pts',(0.0997713324422876,0.0174672310611066,
-1.14539332089791));
#39991=CARTESIAN_POINT('Ctrl Pts',(0.0998996855624999,-0.0158403176033588,
-1.14735916044895));
#39992=CARTESIAN_POINT('Ctrl Pts',(0.0869546080653753,-0.0426125957048284,
-1.149325));
#39993=CARTESIAN_POINT('',(-0.096675,-1.1839272930757E-17,-1.149325));
#39994=CARTESIAN_POINT('Origin',(0.,0.,-1.149325));
#39995=CARTESIAN_POINT('',(-0.096675,-1.1839272930757E-17,-1.179325));
#39996=CARTESIAN_POINT('',(-0.096675,-1.1839272930757E-17,-0.593));
#39997=CARTESIAN_POINT('Origin',(0.,0.,-1.179325));
#39998=CARTESIAN_POINT('',(0.08682622236805,0.0425119128515047,-1.149325));
#39999=CARTESIAN_POINT('Origin',(0.,0.,-1.149325));
#40000=CARTESIAN_POINT('Ctrl Pts',(0.08682622236805,0.0425119128515047,
-1.149325));
#40001=CARTESIAN_POINT('Ctrl Pts',(0.0726941095669478,0.0713753039881243,
-1.14720870321845));
#40002=CARTESIAN_POINT('Ctrl Pts',(0.0431634374388978,0.0923900516972262,
-1.1450924064369));
#40003=CARTESIAN_POINT('Ctrl Pts',(0.0114476307410008,0.0961473177162503,
-1.14297610965536));
#40004=CARTESIAN_POINT('Ctrl Pts',(-0.0202681759568963,0.0999045837352744,
-1.14085981287381));
#40005=CARTESIAN_POINT('Ctrl Pts',(-0.0541691172246404,0.0864043680642206,
-1.13874351609226));
#40006=CARTESIAN_POINT('Ctrl Pts',(-0.0745947204902793,0.061772848111434,
-1.13662721931071));
#40007=CARTESIAN_POINT('Ctrl Pts',(-0.0887620388480758,0.0446882812436053,
-1.1351593434368));
#40008=CARTESIAN_POINT('Ctrl Pts',(-0.0964465189036506,0.0222485651587381,
-1.13369146756288));
#40009=CARTESIAN_POINT('Ctrl Pts',(-0.096611016528836,-7.98840753066898E-5,
-1.13222359168897));
#40010=CARTESIAN_POINT('Origin',(0.,0.,-0.593));
#40011=CARTESIAN_POINT('',(-0.0968310164775401,-1.30139444537575E-5,-1.08642640831103));
#40012=CARTESIAN_POINT('',(-0.0968328216949734,-3.70492603851143E-6,-1.09222359168897));
#40013=CARTESIAN_POINT('',(-0.096675,-1.1839272930757E-17,-0.593));
#40014=CARTESIAN_POINT('Ctrl Pts',(-0.0968310164775401,-1.30139444537575E-5,
-1.08642640831103));
#40015=CARTESIAN_POINT('Ctrl Pts',(-0.0967718957105941,0.0312797356956772,
-1.08849639173725));
#40016=CARTESIAN_POINT('Ctrl Pts',(-0.0802107361021334,0.062626267764312,
-1.09056637516347));
#40017=CARTESIAN_POINT('Ctrl Pts',(-0.0543031633502282,0.0801738568737231,
-1.0926363585897));
#40018=CARTESIAN_POINT('Ctrl Pts',(-0.0278159402458969,0.0981140518944984,
-1.09475265537124));
#40019=CARTESIAN_POINT('Ctrl Pts',(0.00844060388293086,0.101630927348887,
-1.09686895215279));
#40020=CARTESIAN_POINT('Ctrl Pts',(0.0378818670011569,0.0891158908792016,
-1.09898524893434));
#40021=CARTESIAN_POINT('Ctrl Pts',(0.0673231301193828,0.076600854409516,
-1.10110154571589));
#40022=CARTESIAN_POINT('Ctrl Pts',(0.0899491122270068,0.0480539060157556,
-1.10321784249744));
#40023=CARTESIAN_POINT('Ctrl Pts',(0.095411217499768,0.0165326330719422,
-1.10533413927899));
#40024=CARTESIAN_POINT('Ctrl Pts',(0.100873322772529,-0.0149886398718715,
-1.10745043606053));
#40025=CARTESIAN_POINT('Ctrl Pts',(0.0891715512104276,-0.0494842373657385,
-1.10956673284208));
#40026=CARTESIAN_POINT('Ctrl Pts',(0.0656569152152473,-0.0711752102609996,
-1.11168302962363));
#40027=CARTESIAN_POINT('Ctrl Pts',(0.0421422792200671,-0.0928661831562607,
-1.11379932640518));
#40028=CARTESIAN_POINT('Ctrl Pts',(0.00681477879180795,-0.101752531452916,
-1.11591562318673));
#40029=CARTESIAN_POINT('Ctrl Pts',(-0.0241634814538951,-0.0937700019294862,
-1.11803191996828));
#40030=CARTESIAN_POINT('Ctrl Pts',(-0.0551417416995981,-0.0857874724060563,
-1.12014821674983));
#40031=CARTESIAN_POINT('Ctrl Pts',(-0.0817707617627451,-0.0609360650625416,
-1.12226451353137));
#40032=CARTESIAN_POINT('Ctrl Pts',(-0.0918755710391218,-0.03058222241221,
-1.12438081031292));
#40033=CARTESIAN_POINT('Ctrl Pts',(-0.0951313175562236,-0.020802283495351,
-1.12506267631229));
#40034=CARTESIAN_POINT('Ctrl Pts',(-0.0966716630929989,-0.0104511292241676,
-1.12574454231166));
#40035=CARTESIAN_POINT('Ctrl Pts',(-0.0965944740297558,-7.73963603528036E-5,
-1.12642640831103));
#40036=CARTESIAN_POINT('Ctrl Pts',(-0.096611016528836,-7.98840753066898E-5,
-1.13222359168897));
#40037=CARTESIAN_POINT('Ctrl Pts',(-0.0966836818688159,-0.0099432748263196,
-1.13157517078133));
#40038=CARTESIAN_POINT('Ctrl Pts',(-0.0952889348227196,-0.0197849535113047,
-1.1309267498737));
#40039=CARTESIAN_POINT('Ctrl Pts',(-0.0923373744382648,-0.0291337196589252,
-1.13027832896607));
#40040=CARTESIAN_POINT('Ctrl Pts',(-0.0827041598570778,-0.0596459432419781,
-1.12816203218452));
#40041=CARTESIAN_POINT('Ctrl Pts',(-0.0564874654311699,-0.0849075661735644,
-1.12604573540297));
#40042=CARTESIAN_POINT('Ctrl Pts',(-0.0256429766363193,-0.0933758123919359,
-1.12392943862142));
#40043=CARTESIAN_POINT('Ctrl Pts',(0.00520151215853144,-0.101844058610307,
-1.12181314183987));
#40044=CARTESIAN_POINT('Ctrl Pts',(0.040673795322325,-0.0935189281154639,
-1.11969684505832));
#40045=CARTESIAN_POINT('Ctrl Pts',(0.0645295176708119,-0.0722020325036736,
-1.11758054827677));
#40046=CARTESIAN_POINT('Ctrl Pts',(0.0883852400192985,-0.0508851368918835,
-1.11546425149523));
#40047=CARTESIAN_POINT('Ctrl Pts',(0.100624401552479,-0.0165764761631469,
-1.11334795471368));
#40048=CARTESIAN_POINT('Ctrl Pts',(0.0956586130205045,0.0150273819453597,
-1.11123165793213));
#40049=CARTESIAN_POINT('Ctrl Pts',(0.0906928244885304,0.0466312400538666,
-1.10911536115058));
#40050=CARTESIAN_POINT('Ctrl Pts',(0.0685220858914019,0.0755302955421434,
-1.10699906436903));
#40051=CARTESIAN_POINT('Ctrl Pts',(0.0392823152972172,0.0885075508075104,
-1.10488276758748));
#40052=CARTESIAN_POINT('Ctrl Pts',(0.0100425447030326,0.101484806072877,
-1.10276647080593));
#40053=CARTESIAN_POINT('Ctrl Pts',(-0.0262662578882083,0.0985402611153346,
-1.10065017402439));
#40054=CARTESIAN_POINT('Ctrl Pts',(-0.0530332437966072,0.0810198486041363,
-1.09853387724284));
#40055=CARTESIAN_POINT('Ctrl Pts',(-0.0796374715166379,0.06360596996304,
-1.09643044872488));
#40056=CARTESIAN_POINT('Ctrl Pts',(-0.0968155688864563,0.0317929436444108,
-1.09432702020692));
#40057=CARTESIAN_POINT('Ctrl Pts',(-0.0968328216949734,-3.70492603851143E-6,
-1.09222359168897));
#40058=CARTESIAN_POINT('Origin',(0.,0.,-0.593));
#40059=CARTESIAN_POINT('',(-0.0966316008371174,8.59389927197543E-5,-1.04642640831103));
#40060=CARTESIAN_POINT('',(-0.0966173831184959,8.35728303465981E-5,-1.05222359168897));
#40061=CARTESIAN_POINT('',(-0.096675,-1.1839272930757E-17,-0.593));
#40062=CARTESIAN_POINT('Ctrl Pts',(-0.0966316008371174,8.59389927197543E-5,
-1.04642640831103));
#40063=CARTESIAN_POINT('Ctrl Pts',(-0.0967086374933281,0.00904146025168611,
-1.04701564759975));
#40064=CARTESIAN_POINT('Ctrl Pts',(-0.0955657530108521,0.0179776896157913,
-1.04760488688846));
#40065=CARTESIAN_POINT('Ctrl Pts',(-0.0931241231896304,0.0265437297547207,
-1.04819412617718));
#40066=CARTESIAN_POINT('Ctrl Pts',(-0.0843548278772829,0.057309300760937,
-1.05031042295873));
#40067=CARTESIAN_POINT('Ctrl Pts',(-0.0588324876973109,0.08329965024076,
-1.05242671974028));
#40068=CARTESIAN_POINT('Ctrl Pts',(-0.0282313235457831,0.0926264786465709,
-1.05454301652182));
#40069=CARTESIAN_POINT('Ctrl Pts',(0.00236984060574432,0.101953307052382,
-1.05665931330337));
#40070=CARTESIAN_POINT('Ctrl Pts',(0.0380498287288274,0.094616614384181,
-1.05877561008492));
#40071=CARTESIAN_POINT('Ctrl Pts',(0.0624881756074684,0.0739722936785937,
-1.06089190686647));
#40072=CARTESIAN_POINT('Ctrl Pts',(0.0869265224861093,0.0533279729730065,
-1.06300820364802));
#40073=CARTESIAN_POINT('Ctrl Pts',(0.100123228120308,0.0193760242300328,
-1.06512450042957));
#40074=CARTESIAN_POINT('Ctrl Pts',(0.0960419776750078,-0.0123535252285019,
-1.06724079721111));
#40075=CARTESIAN_POINT('Ctrl Pts',(0.0919607272297077,-0.0440830746870368,
-1.06935709399266));
#40076=CARTESIAN_POINT('Ctrl Pts',(0.0706015207049087,-0.0735902248611326,
-1.07147339077421));
#40077=CARTESIAN_POINT('Ctrl Pts',(0.0417342836900796,-0.0873780446853105,
-1.07358968755576));
#40078=CARTESIAN_POINT('Ctrl Pts',(0.0128670466752505,-0.101165864509488,
-1.07570598433731));
#40079=CARTESIAN_POINT('Ctrl Pts',(-0.0235082208296085,-0.0992343539837484,
-1.07782228111886));
#40080=CARTESIAN_POINT('Ctrl Pts',(-0.0507529716286648,-0.082467019364773,
-1.07993857790041));
#40081=CARTESIAN_POINT('Ctrl Pts',(-0.0779977224277213,-0.0656996847457975,
-1.08205487468195));
#40082=CARTESIAN_POINT('Ctrl Pts',(-0.0961119565209748,-0.0340965260335864,
-1.0841711714635));
#40083=CARTESIAN_POINT('Ctrl Pts',(-0.0968101225276843,-0.00211318938389995,
-1.08628746824505));
#40084=CARTESIAN_POINT('Ctrl Pts',(-0.0968254012970081,-0.0014132612605281,
-1.08633378160038));
#40085=CARTESIAN_POINT('Ctrl Pts',(-0.0968323392326173,-0.000713151063858057,
-1.08638009495571));
#40086=CARTESIAN_POINT('Ctrl Pts',(-0.0968310164775401,-1.30139444537575E-5,
-1.08642640831103));
#40087=CARTESIAN_POINT('Ctrl Pts',(-0.0968328216949734,-3.70492603851143E-6,
-1.09222359168897));
#40088=CARTESIAN_POINT('Ctrl Pts',(-0.096850285600455,-0.032189401806551,
-1.09009442664383));
#40089=CARTESIAN_POINT('Ctrl Pts',(-0.0791875082743585,-0.0643577242998591,
-1.08796526159869));
#40090=CARTESIAN_POINT('Ctrl Pts',(-0.0520464468139391,-0.0816568732620622,
-1.08583609655355));
#40091=CARTESIAN_POINT('Ctrl Pts',(-0.0250694207033475,-0.0988514694986514,
-1.083719799772));
#40092=CARTESIAN_POINT('Ctrl Pts',(0.0112710839020407,-0.101356085477478,
-1.08160350299045));
#40093=CARTESIAN_POINT('Ctrl Pts',(0.0403520772773434,-0.0880249422318465,
-1.0794872062089));
#40094=CARTESIAN_POINT('Ctrl Pts',(0.069433070652646,-0.074693798986215,
-1.07737090942735));
#40095=CARTESIAN_POINT('Ctrl Pts',(0.0912545527978629,-0.045526896516125,
-1.07525461264581));
#40096=CARTESIAN_POINT('Ctrl Pts',(0.0958353288144589,-0.013865599655261,
-1.07313831586426));
#40097=CARTESIAN_POINT('Ctrl Pts',(0.100416104831055,0.0177956972056032,
-1.07102201908271));
#40098=CARTESIAN_POINT('Ctrl Pts',(0.0877561747190295,0.0519513884572417,
-1.06890572230116));
#40099=CARTESIAN_POINT('Ctrl Pts',(0.0636462302200924,0.0729782879168203,
-1.06678942551961));
#40100=CARTESIAN_POINT('Ctrl Pts',(0.0395362857211552,0.0940051873763989,
-1.06467312873806));
#40101=CARTESIAN_POINT('Ctrl Pts',(0.00397632683530639,0.101903295043918,
-1.06255683195652));
#40102=CARTESIAN_POINT('Ctrl Pts',(-0.0267680336791695,0.0930599012284323,
-1.06044053517497));
#40103=CARTESIAN_POINT('Ctrl Pts',(-0.0575123941936451,0.084216507412947,
-1.05832423839342));
#40104=CARTESIAN_POINT('Ctrl Pts',(-0.0834411563367478,0.0586316121144577,
-1.05620794161187));
#40105=CARTESIAN_POINT('Ctrl Pts',(-0.0926942234682325,0.0280080651033813,
-1.05409164483032));
#40106=CARTESIAN_POINT('Ctrl Pts',(-0.0954167812986275,0.0189976065684176,
-1.05346896044987));
#40107=CARTESIAN_POINT('Ctrl Pts',(-0.0966956730758621,0.00955093650367408,
-1.05284627606942));
#40108=CARTESIAN_POINT('Ctrl Pts',(-0.0966173831184959,8.35728303465981E-5,
-1.05222359168897));
#40109=CARTESIAN_POINT('Origin',(0.,0.,-0.593));
#40110=CARTESIAN_POINT('',(-0.096532558168651,-4.01631997834981E-5,-1.00642640831103));
#40111=CARTESIAN_POINT('',(-0.096539508889345,-4.74460931573492E-5,-1.01222359168897));
#40112=CARTESIAN_POINT('',(-0.096675,-1.1839272930757E-17,-0.593));
#40113=CARTESIAN_POINT('Ctrl Pts',(-0.096532558168651,-4.01631997834981E-5,
-1.00642640831103));
#40114=CARTESIAN_POINT('Ctrl Pts',(-0.0964626778726808,0.0186229076283818,
-1.00765120024379));
#40115=CARTESIAN_POINT('Ctrl Pts',(-0.0912497818101863,0.0373220779001833,
-1.00887599217655));
#40116=CARTESIAN_POINT('Ctrl Pts',(-0.0811472458103819,0.0528374540286397,
-1.01010078410931));
#40117=CARTESIAN_POINT('Ctrl Pts',(-0.0636912487140321,0.0796462038962325,
-1.01221708089086));
#40118=CARTESIAN_POINT('Ctrl Pts',(-0.0316368472773319,0.0969494861144909,
-1.0143333776724));
#40119=CARTESIAN_POINT('Ctrl Pts',(0.000353889460091694,0.0968325710537681,
-1.01644967445395));
#40120=CARTESIAN_POINT('Ctrl Pts',(0.0323446261975153,0.0967156559930454,
-1.0185659712355));
#40121=CARTESIAN_POINT('Ctrl Pts',(0.0642716982356621,0.0791785436533415,
-1.02068226801705));
#40122=CARTESIAN_POINT('Ctrl Pts',(0.0815312782370999,0.0522429203921152,
-1.0227985647986));
#40123=CARTESIAN_POINT('Ctrl Pts',(0.0987908582385379,0.0253072971308888,
-1.02491486158015));
#40124=CARTESIAN_POINT('Ctrl Pts',(0.101382946203267,-0.0110268370518601,
-1.02703115836169));
#40125=CARTESIAN_POINT('Ctrl Pts',(0.0881218902579705,-0.0401398117892546,
-1.02914745514324));
#40126=CARTESIAN_POINT('Ctrl Pts',(0.0748608343126744,-0.0692527865266491,
-1.03126375192479));
#40127=CARTESIAN_POINT('Ctrl Pts',(0.0457466344573533,-0.0911446018186895,
-1.03338004870634));
#40128=CARTESIAN_POINT('Ctrl Pts',(0.0140964755307833,-0.0958016776657067,
-1.03549634548789));
#40129=CARTESIAN_POINT('Ctrl Pts',(-0.0175536833957866,-0.100458753512724,
-1.03761264226944));
#40130=CARTESIAN_POINT('Ctrl Pts',(-0.0517398013936054,-0.0878810899147185,
-1.03972893905098));
#40131=CARTESIAN_POINT('Ctrl Pts',(-0.0728247351701532,-0.0638218618494113,
-1.04184523583253));
#40132=CARTESIAN_POINT('Ctrl Pts',(-0.0880390030318676,-0.0464614307372775,
-1.04337229332537));
#40133=CARTESIAN_POINT('Ctrl Pts',(-0.0964319546062191,-0.0231229611988117,
-1.0448993508182));
#40134=CARTESIAN_POINT('Ctrl Pts',(-0.0966316008371174,8.59389927197543E-5,
-1.04642640831103));
#40135=CARTESIAN_POINT('Ctrl Pts',(-0.0966173831184959,8.35728303465981E-5,
-1.05222359168897));
#40136=CARTESIAN_POINT('Ctrl Pts',(-0.0964295915905974,-0.0226254788692061,
-1.05072997928787));
#40137=CARTESIAN_POINT('Ctrl Pts',(-0.0884331154221412,-0.0454535933732362,
-1.04923636688677));
#40138=CARTESIAN_POINT('Ctrl Pts',(-0.0738215226618864,-0.0626662176126394,
-1.04774275448568));
#40139=CARTESIAN_POINT('Ctrl Pts',(-0.0531183826041891,-0.0870547545939195,
-1.04562645770413));
#40140=CARTESIAN_POINT('Ctrl Pts',(-0.0191347303689279,-0.100169629832816,
-1.04351016092258));
#40141=CARTESIAN_POINT('Ctrl Pts',(0.0125848936453956,-0.0960119385413782,
-1.04139386414103));
#40142=CARTESIAN_POINT('Ctrl Pts',(0.0443045176597189,-0.0918542472499407,
-1.03927756735948));
#40143=CARTESIAN_POINT('Ctrl Pts',(0.0737601134531046,-0.0704239894281696,
-1.03716127057793));
#40144=CARTESIAN_POINT('Ctrl Pts',(0.0874783414676494,-0.0415236245754575,
-1.03504497379639));
#40145=CARTESIAN_POINT('Ctrl Pts',(0.101196569482194,-0.0126232597227454,
-1.03292867701484));
#40146=CARTESIAN_POINT('Ctrl Pts',(0.0991774297178981,0.0237472121609076,
-1.03081238023329));
#40147=CARTESIAN_POINT('Ctrl Pts',(0.0823444985901786,0.0509515001679581,
-1.02869608345174));
#40148=CARTESIAN_POINT('Ctrl Pts',(0.0655115674624591,0.0781557881750087,
-1.02657978667019));
#40149=CARTESIAN_POINT('Ctrl Pts',(0.0338648449713159,0.0961938923054568,
-1.02446348988864));
#40150=CARTESIAN_POINT('Ctrl Pts',(0.00187992427854601,0.09681496612358,
-1.02234719310709));
#40151=CARTESIAN_POINT('Ctrl Pts',(-0.0301049964142237,0.0974360399417031,
-1.02023089632555));
#40152=CARTESIAN_POINT('Ctrl Pts',(-0.0624281153086202,0.0806400834475018,
-1.018114599544));
#40153=CARTESIAN_POINT('Ctrl Pts',(-0.0803044493353819,0.0541097695880409,
-1.01599830276245));
#40154=CARTESIAN_POINT('Ctrl Pts',(-0.0909327626848177,0.0383362620816862,
-1.01474006573796));
#40155=CARTESIAN_POINT('Ctrl Pts',(-0.0964543450128613,0.0191217990142187,
-1.01348182871346));
#40156=CARTESIAN_POINT('Ctrl Pts',(-0.096539508889345,-4.74460931573492E-5,
-1.01222359168897));
#40157=CARTESIAN_POINT('Origin',(0.,0.,-0.593));
#40158=CARTESIAN_POINT('',(-0.0967783240400222,-6.36632972197126E-5,-0.966426408311032));
#40159=CARTESIAN_POINT('',(-0.0967903835966408,-5.70231646415709E-5,-0.972223591688967));
#40160=CARTESIAN_POINT('',(-0.096675,-1.1839272930757E-17,-0.593));
#40161=CARTESIAN_POINT('Ctrl Pts',(-0.0967783240400222,-6.36632972197126E-5,
-0.966426408311032));
#40162=CARTESIAN_POINT('Ctrl Pts',(-0.0965638778054847,0.0281004551149537,
-0.968286752887833));
#40163=CARTESIAN_POINT('Ctrl Pts',(-0.083560586212758,0.0564370375535735,
-0.970147097464634));
#40164=CARTESIAN_POINT('Ctrl Pts',(-0.0619458247367958,0.0744270572529086,
-0.972007442041436));
#40165=CARTESIAN_POINT('Ctrl Pts',(-0.0373572346895846,0.094892201863463,
-0.974123738822984));
#40166=CARTESIAN_POINT('Ctrl Pts',(-0.0016245794286527,0.10196790524414,
-0.976240035604533));
#40167=CARTESIAN_POINT('Ctrl Pts',(0.028907594321538,0.0924176554789381,
-0.978356332386081));
#40168=CARTESIAN_POINT('Ctrl Pts',(0.0594397680717282,0.0828674057137362,
-0.980472629167629));
#40169=CARTESIAN_POINT('Ctrl Pts',(0.0847714603111776,0.0566912028026555,
-0.982588925949178));
#40170=CARTESIAN_POINT('Ctrl Pts',(0.0933156500194906,0.025862357111442,
-0.984705222730726));
#40171=CARTESIAN_POINT('Ctrl Pts',(0.101859839727804,-0.00496648857977159,
-0.986821519512274));
#40172=CARTESIAN_POINT('Ctrl Pts',(0.0936165269049802,-0.0404479770511177,
-0.988937816293823));
#40173=CARTESIAN_POINT('Ctrl Pts',(0.0723563020911069,-0.0643524482907502,
-0.991054113075372));
#40174=CARTESIAN_POINT('Ctrl Pts',(0.0510960772772336,-0.0882569195303827,
-0.99317040985692));
#40175=CARTESIAN_POINT('Ctrl Pts',(0.0168189404723104,-0.100584373538301,
-0.995286706638468));
#40176=CARTESIAN_POINT('Ctrl Pts',(-0.0147963332778374,-0.0956960844300254,
-0.997403003420017));
#40177=CARTESIAN_POINT('Ctrl Pts',(-0.0464116070279851,-0.0908077953217495,
-0.999519300201565));
#40178=CARTESIAN_POINT('Ctrl Pts',(-0.0753650177233574,-0.0687037630972791,
-1.00163559698311));
#40179=CARTESIAN_POINT('Ctrl Pts',(-0.0884129266930442,-0.0394946382265804,
-1.00375189376466));
#40180=CARTESIAN_POINT('Ctrl Pts',(-0.0939094497773613,-0.0271900896971962,
-1.00464339861345));
#40181=CARTESIAN_POINT('Ctrl Pts',(-0.0965834228265787,-0.0136246894295979,
-1.00553490346224));
#40182=CARTESIAN_POINT('Ctrl Pts',(-0.096532558168651,-4.01631997834981E-5,
-1.00642640831103));
#40183=CARTESIAN_POINT('Ctrl Pts',(-0.096539508889345,-4.74460931573492E-5,
-1.01222359168897));
#40184=CARTESIAN_POINT('Ctrl Pts',(-0.0965975867345704,-0.0131199892464291,
-1.01136553193191));
#40185=CARTESIAN_POINT('Ctrl Pts',(-0.0941273970619773,-0.0261715032790142,
-1.01050747217486));
#40186=CARTESIAN_POINT('Ctrl Pts',(-0.0890243793814782,-0.0380963469727379,
-1.0096494124178));
#40187=CARTESIAN_POINT('Ctrl Pts',(-0.0764384262416856,-0.0675074784493349,
-1.00753311563626));
#40188=CARTESIAN_POINT('Ctrl Pts',(-0.0478369708029737,-0.0900650701778077,
-1.00541681885471));
#40189=CARTESIAN_POINT('Ctrl Pts',(-0.016302663323126,-0.0954510080514942,
-1.00330052207316));
#40190=CARTESIAN_POINT('Ctrl Pts',(0.0152316441567213,-0.100836945925181,
-1.00118422529161));
#40191=CARTESIAN_POINT('Ctrl Pts',(0.0496988036777041,-0.0890512299440807,
-0.999067928510063));
#40192=CARTESIAN_POINT('Ctrl Pts',(0.07133312159954,-0.0654847885278765,
-0.996951631728514));
#40193=CARTESIAN_POINT('Ctrl Pts',(0.0929674395213759,-0.0419183471116724,
-0.994835334946965));
#40194=CARTESIAN_POINT('Ctrl Pts',(0.101768915844065,-0.00657118026036393,
-0.992719038165417));
#40195=CARTESIAN_POINT('Ctrl Pts',(0.0937116492784364,0.0243884923567606,
-0.990602741383869));
#40196=CARTESIAN_POINT('Ctrl Pts',(0.0856543827128077,0.0553481649738856,
-0.98848644460232));
#40197=CARTESIAN_POINT('Ctrl Pts',(0.060738373258861,0.0819203433568267,
-0.986370147820772));
#40198=CARTESIAN_POINT('Ctrl Pts',(0.0303605036494764,0.0919505931829567,
-0.984253851039224));
#40199=CARTESIAN_POINT('Ctrl Pts',(-1.7365959907794E-5,0.101980843009087,
-0.982137554257675));
#40200=CARTESIAN_POINT('Ctrl Pts',(-0.0358570957247298,0.0954691642784059,
-0.980021257476126));
#40201=CARTESIAN_POINT('Ctrl Pts',(-0.0607651617655735,0.075394077245872,
-0.977904960694578));
#40202=CARTESIAN_POINT('Ctrl Pts',(-0.0830543976339355,0.0574296817278774,
-0.976011171026041));
#40203=CARTESIAN_POINT('Ctrl Pts',(-0.0965898337721487,0.0286040520070571,
-0.974117381357504));
#40204=CARTESIAN_POINT('Ctrl Pts',(-0.0967903835966408,-5.70231646415709E-5,
-0.972223591688967));
#40205=CARTESIAN_POINT('Origin',(0.,0.,-0.593));
#40206=CARTESIAN_POINT('',(-0.0967266999094946,8.16697450527169E-5,-0.926426408311032));
#40207=CARTESIAN_POINT('',(-0.09671155539721,8.46130275593083E-5,-0.932223591688967));
#40208=CARTESIAN_POINT('',(-0.096675,-1.1839272930757E-17,-0.593));
#40209=CARTESIAN_POINT('Ctrl Pts',(-0.0967266999094946,8.16697450527169E-5,
-0.926426408311032));
#40210=CARTESIAN_POINT('Ctrl Pts',(-0.0967785360195961,0.00583649577189784,
-0.926806008750327));
#40211=CARTESIAN_POINT('Ctrl Pts',(-0.0963090658617653,0.0115828782139499,
-0.927185609189623));
#40212=CARTESIAN_POINT('Ctrl Pts',(-0.0952880641309304,0.0172295353356017,
-0.927565209628919));
#40213=CARTESIAN_POINT('Ctrl Pts',(-0.089595914035079,0.048710010740837,
-0.929681506410467));
#40214=CARTESIAN_POINT('Ctrl Pts',(-0.0667614237514503,0.0770908895838589,
-0.931797803192016));
#40215=CARTESIAN_POINT('Ctrl Pts',(-0.0372293640561305,0.0893904161847099,
-0.933914099973564));
#40216=CARTESIAN_POINT('Ctrl Pts',(-0.00769730436081029,0.101689942785561,
-0.936030396755112));
#40217=CARTESIAN_POINT('Ctrl Pts',(0.0285323247462011,0.0979081171442405,
-0.93814669353666));
#40218=CARTESIAN_POINT('Ctrl Pts',(0.0548876547176703,0.0797747918411131,
-0.940262990318209));
#40219=CARTESIAN_POINT('Ctrl Pts',(0.0812429846891394,0.0616414665379859,
-0.942379287099758));
#40220=CARTESIAN_POINT('Ctrl Pts',(0.0977240155250663,0.0291566415730521,
-0.944495583881307));
#40221=CARTESIAN_POINT('Ctrl Pts',(0.0967921252944012,-0.00282073300728408,
-0.946611880662855));
#40222=CARTESIAN_POINT('Ctrl Pts',(0.0958602350637361,-0.0347981075876205,
-0.948728177444403));
#40223=CARTESIAN_POINT('Ctrl Pts',(0.0775154237664787,-0.0662680317833592,
-0.950844474225951));
#40224=CARTESIAN_POINT('Ctrl Pts',(0.0501488289561232,-0.0828357833790652,
-0.9529607710075));
#40225=CARTESIAN_POINT('Ctrl Pts',(0.0227822341457677,-0.0994035349747711,
-0.955077067789048));
#40226=CARTESIAN_POINT('Ctrl Pts',(-0.0136061441776863,-0.101069113970444,
-0.957193364570597));
#40227=CARTESIAN_POINT('Ctrl Pts',(-0.0423718236643878,-0.0870706644803458,
-0.959309661352146));
#40228=CARTESIAN_POINT('Ctrl Pts',(-0.071137503151089,-0.0730722149902475,
-0.961425958133694));
#40229=CARTESIAN_POINT('Ctrl Pts',(-0.0922804838010382,-0.0434097370143778,
-0.963542254915242));
#40230=CARTESIAN_POINT('Ctrl Pts',(-0.0961297117092678,-0.0116512051062275,
-0.96565855169679));
#40231=CARTESIAN_POINT('Ctrl Pts',(-0.0965952505591475,-0.00781021912907144,
-0.965914503901537));
#40232=CARTESIAN_POINT('Ctrl Pts',(-0.0968078282443584,-0.00393857351130197,
-0.966170456106285));
#40233=CARTESIAN_POINT('Ctrl Pts',(-0.0967783240400222,-6.36632972197126E-5,
-0.966426408311032));
#40234=CARTESIAN_POINT('Ctrl Pts',(-0.0967903835966408,-5.70231646415709E-5,
-0.972223591688967));
#40235=CARTESIAN_POINT('Ctrl Pts',(-0.096813946806011,-0.00342450013328669,
-0.972001084575956));
#40236=CARTESIAN_POINT('Ctrl Pts',(-0.0966534270383089,-0.00678970548966747,
-0.971778577462944));
#40237=CARTESIAN_POINT('Ctrl Pts',(-0.0963013940171612,-0.0101347559966597,
-0.971556070349933));
#40238=CARTESIAN_POINT('Ctrl Pts',(-0.09295315791104,-0.0419500068722704,
-0.969439773568385));
#40239=CARTESIAN_POINT('Ctrl Pts',(-0.0722802833819321,-0.0719420132891045,
-0.967323476786836));
#40240=CARTESIAN_POINT('Ctrl Pts',(-0.043738792138609,-0.0863920704160863,
-0.965207180005287));
#40241=CARTESIAN_POINT('Ctrl Pts',(-0.0151973008952858,-0.100842127543068,
-0.963090883223739));
#40242=CARTESIAN_POINT('Ctrl Pts',(0.0212128070622524,-0.0997502353801977,
-0.960974586442191));
#40243=CARTESIAN_POINT('Ctrl Pts',(0.0488371099897059,-0.0836158385495418,
-0.958858289660643));
#40244=CARTESIAN_POINT('Ctrl Pts',(0.0764614129171591,-0.0674814417188861,
-0.956741992879094));
#40245=CARTESIAN_POINT('Ctrl Pts',(0.0952999108145277,-0.036304540220445,
-0.954625696097545));
#40246=CARTESIAN_POINT('Ctrl Pts',(0.0967356479326414,-0.00434582415965373,
-0.952509399315997));
#40247=CARTESIAN_POINT('Ctrl Pts',(0.0981713850507552,0.0276128919011376,
-0.950393102534449));
#40248=CARTESIAN_POINT('Ctrl Pts',(0.0822043613896141,0.0603534225242792,
-0.9482768057529));
#40249=CARTESIAN_POINT('Ctrl Pts',(0.0561380858105309,0.0788998548164988,
-0.946160508971352));
#40250=CARTESIAN_POINT('Ctrl Pts',(0.0300718102314475,0.0974462871087184,
-0.944044212189803));
#40251=CARTESIAN_POINT('Ctrl Pts',(-0.00609371726557807,0.101798621070016,
-0.941927915408255));
#40252=CARTESIAN_POINT('Ctrl Pts',(-0.0358159489817476,0.0899660467458193,
-0.939811618626706));
#40253=CARTESIAN_POINT('Ctrl Pts',(-0.0655381806979173,0.0781334724216229,
-0.937695321845158));
#40254=CARTESIAN_POINT('Ctrl Pts',(-0.0888171166332309,0.0501159898119325,
-0.93557902506361));
#40255=CARTESIAN_POINT('Ctrl Pts',(-0.0950046912193912,0.0187291327843489,
-0.933462728282061));
#40256=CARTESIAN_POINT('Ctrl Pts',(-0.096212343214622,0.0126032429085056,
-0.93304968275103));
#40257=CARTESIAN_POINT('Ctrl Pts',(-0.0967689376763235,0.00634900418126095,
-0.932636637219998));
#40258=CARTESIAN_POINT('Ctrl Pts',(-0.09671155539721,8.46130275593083E-5,
-0.932223591688967));
#40259=CARTESIAN_POINT('Origin',(0.,0.,-0.593));
#40260=CARTESIAN_POINT('',(-0.0965175797178924,1.07195340507057E-5,-0.886426408311032));
#40261=CARTESIAN_POINT('',(-0.0965165233765785,2.38684902196363E-6,-0.892223591688966));
#40262=CARTESIAN_POINT('',(-0.096675,-1.1839272930757E-17,-0.593));
#40263=CARTESIAN_POINT('Ctrl Pts',(-0.0965175797178924,1.07195340507057E-5,
-0.886426408311032));
#40264=CARTESIAN_POINT('Ctrl Pts',(-0.0965329025079771,0.015485362273297,
-0.88744156139437));
#40265=CARTESIAN_POINT('Ctrl Pts',(-0.0930271006338032,0.0309534509611169,
-0.888456714477709));
#40266=CARTESIAN_POINT('Ctrl Pts',(-0.085962915872296,0.0445763294634369,
-0.889471867561047));
#40267=CARTESIAN_POINT('Ctrl Pts',(-0.0712361601539585,0.0729760402096004,
-0.891588164342595));
#40268=CARTESIAN_POINT('Ctrl Pts',(-0.0410446601273461,0.0933564611217898,
-0.893704461124144));
#40269=CARTESIAN_POINT('Ctrl Pts',(-0.00919837140112475,0.0963953423006903,
-0.895820757905692));
#40270=CARTESIAN_POINT('Ctrl Pts',(0.0226479173250966,0.0994342234795908,
-0.897937054687241));
#40271=CARTESIAN_POINT('Ctrl Pts',(0.0561489947509267,0.0851315649252025,
-0.900053351468789));
#40272=CARTESIAN_POINT('Ctrl Pts',(0.0759810647189922,0.0600295748599686,
-0.902169648250338));
#40273=CARTESIAN_POINT('Ctrl Pts',(0.0958131346870579,0.0349275847947343,
-0.904285945031886));
#40274=CARTESIAN_POINT('Ctrl Pts',(0.101976197197358,-0.000973736781346012,
-0.906402241813434));
#40275=CARTESIAN_POINT('Ctrl Pts',(0.091651193256279,-0.0312526931383618,
-0.908518538594983));
#40276=CARTESIAN_POINT('Ctrl Pts',(0.0813261893151997,-0.0615316494953771,
-0.910634835376531));
#40277=CARTESIAN_POINT('Ctrl Pts',(0.054513118922741,-0.086188240633328,
-0.912751132158081));
#40278=CARTESIAN_POINT('Ctrl Pts',(0.0234766032976432,-0.0939442449078458,
-0.914867428939629));
#40279=CARTESIAN_POINT('Ctrl Pts',(-0.00755991232745468,-0.101700249182364,
-0.916983725721177));
#40280=CARTESIAN_POINT('Ctrl Pts',(-0.0428198731851916,-0.0925556665934481,
-0.919100022502725));
#40281=CARTESIAN_POINT('Ctrl Pts',(-0.0661749486600234,-0.070693339315266,
-0.921216319284273));
#40282=CARTESIAN_POINT('Ctrl Pts',(-0.0853408210952234,-0.0527524606312398,
-0.922953015626526));
#40283=CARTESIAN_POINT('Ctrl Pts',(-0.0964895463830737,-0.0262470282134427,
-0.924689711968779));
#40284=CARTESIAN_POINT('Ctrl Pts',(-0.0967266999094946,8.16697450527169E-5,
-0.926426408311032));
#40285=CARTESIAN_POINT('Ctrl Pts',(-0.09671155539721,8.46130275593083E-5,
-0.932223591688967));
#40286=CARTESIAN_POINT('Ctrl Pts',(-0.0964749315111858,-0.0257474835929374,
-0.93052034043845));
#40287=CARTESIAN_POINT('Ctrl Pts',(-0.0857979951590669,-0.0517522162392853,
-0.928817089187933));
#40288=CARTESIAN_POINT('Ctrl Pts',(-0.0672808542741755,-0.0696416428344169,
-0.927113837937416));
#40289=CARTESIAN_POINT('Ctrl Pts',(-0.0442732295057914,-0.0918693299801235,
-0.924997541155867));
#40290=CARTESIAN_POINT('Ctrl Pts',(-0.00916176673201553,-0.10156847282606,
-0.92288124437432));
#40291=CARTESIAN_POINT('Ctrl Pts',(0.0219931282431221,-0.094302566659775,
-0.920764947592771));
#40292=CARTESIAN_POINT('Ctrl Pts',(0.0531480232182593,-0.0870366604934904,
-0.918648650811222));
#40293=CARTESIAN_POINT('Ctrl Pts',(0.0803463503947581,-0.0628057053149853,
-0.916532354029673));
#40294=CARTESIAN_POINT('Ctrl Pts',(0.0911472674624636,-0.0326932317562424,
-0.914416057248125));
#40295=CARTESIAN_POINT('Ctrl Pts',(0.101948184530169,-0.0025807581974989,
-0.912299760466577));
#40296=CARTESIAN_POINT('Ctrl Pts',(0.0963516914890807,0.0334132337414824,
-0.910183463685029));
#40297=CARTESIAN_POINT('Ctrl Pts',(0.0769176916362815,0.0588246587910732,
-0.90806716690348));
#40298=CARTESIAN_POINT('Ctrl Pts',(0.0574836917834826,0.0842360838406634,
-0.905950870121932));
#40299=CARTESIAN_POINT('Ctrl Pts',(0.0242121851189731,0.0990649420008637,
-0.903834573340383));
#40300=CARTESIAN_POINT('Ctrl Pts',(-0.00767804063006863,0.0965283350142507,
-0.901718276558835));
#40301=CARTESIAN_POINT('Ctrl Pts',(-0.0395682663791108,0.0939917280276376,
-0.899601979777287));
#40302=CARTESIAN_POINT('Ctrl Pts',(-0.0700772112126856,0.0740896558942112,
-0.897485682995738));
#40303=CARTESIAN_POINT('Ctrl Pts',(-0.0852497164454802,0.0459255660227048,
-0.89536938621419));
#40304=CARTESIAN_POINT('Ctrl Pts',(-0.0927675000744725,0.0319706172180849,
-0.894320788039116));
#40305=CARTESIAN_POINT('Ctrl Pts',(-0.0965200702590053,0.0159872797472848,
-0.893272189864041));
#40306=CARTESIAN_POINT('Ctrl Pts',(-0.0965165486863883,2.38646782571199E-6,
-0.892223591688966));
#40307=CARTESIAN_POINT('Origin',(0.,0.,-0.593));
#40308=CARTESIAN_POINT('',(-0.0966873976231268,-8.74994151896375E-5,-0.846426408311032));
#40309=CARTESIAN_POINT('',(-0.0967028036390754,-8.59090990596172E-5,-0.852223591688967));
#40310=CARTESIAN_POINT('',(-0.096675,-1.1839272930757E-17,-0.593));
#40311=CARTESIAN_POINT('Ctrl Pts',(-0.0966873976231268,-8.74994151896374E-5,
-0.846426408311032));
#40312=CARTESIAN_POINT('Ctrl Pts',(-0.0964563468117902,0.0249637526176381,
-0.848077114038413));
#40313=CARTESIAN_POINT('Ctrl Pts',(-0.0864956095149754,0.0501779485389757,
-0.849727819765794));
#40314=CARTESIAN_POINT('Ctrl Pts',(-0.0689844853064945,0.067954490953125,
-0.851378525493176));
#40315=CARTESIAN_POINT('Ctrl Pts',(-0.0465342476966098,0.0907450095017034,
-0.853494822274724));
#40316=CARTESIAN_POINT('Ctrl Pts',(-0.0116736885465889,0.101310502682944,
-0.855611119056273));
#40317=CARTESIAN_POINT('Ctrl Pts',(0.0196515526778018,0.094818186710419,
-0.857727415837821));
#40318=CARTESIAN_POINT('Ctrl Pts',(0.0509767939021918,0.0883258707378936,
-0.859843712619369));
#40319=CARTESIAN_POINT('Ctrl Pts',(0.0787667172009514,0.064775745611602,
-0.861960009400918));
#40320=CARTESIAN_POINT('Ctrl Pts',(0.0903098770749894,0.0349399221006658,
-0.864076306182466));
#40321=CARTESIAN_POINT('Ctrl Pts',(0.101853036949027,0.00510409858972969,
-0.866192602964014));
#40322=CARTESIAN_POINT('Ctrl Pts',(0.097149433398344,-0.0310174233058513,
-0.868308899745563));
#40323=CARTESIAN_POINT('Ctrl Pts',(0.0783505513169802,-0.0569022245788824,
-0.870425196527111));
#40324=CARTESIAN_POINT('Ctrl Pts',(0.0595516692356162,-0.0827870258519136,
-0.87254149330866));
#40325=CARTESIAN_POINT('Ctrl Pts',(0.0266575086235715,-0.098435106502395,
-0.874657790090208));
#40326=CARTESIAN_POINT('Ctrl Pts',(-0.00528574541949839,-0.0966888460426565,
-0.876774086871757));
#40327=CARTESIAN_POINT('Ctrl Pts',(-0.0372289994625683,-0.0949425855829181,
-0.878890383653305));
#40328=CARTESIAN_POINT('Ctrl Pts',(-0.068221346936663,-0.0758019840129603,
-0.881006680434853));
#40329=CARTESIAN_POINT('Ctrl Pts',(-0.0840865149686794,-0.0480221829379125,
-0.883122977216402));
#40330=CARTESIAN_POINT('Ctrl Pts',(-0.0923414204015161,-0.033567899796709,
-0.884224120914612));
#40331=CARTESIAN_POINT('Ctrl Pts',(-0.0965009589795843,-0.0167747344177196,
-0.885325264612822));
#40332=CARTESIAN_POINT('Ctrl Pts',(-0.0965175797178924,1.07195340507057E-5,
-0.886426408311032));
#40333=CARTESIAN_POINT('Ctrl Pts',(-0.0965165486863883,2.38646782571199E-6,
-0.892223591688966));
#40334=CARTESIAN_POINT('Ctrl Pts',(-0.0965129629676018,-0.0162736749299603,
-0.891155893082492));
#40335=CARTESIAN_POINT('Ctrl Pts',(-0.0926152032764517,-0.0325513493313622,
-0.890088194476018));
#40336=CARTESIAN_POINT('Ctrl Pts',(-0.0848328988951623,-0.0466910166261522,
-0.889020495869544));
#40337=CARTESIAN_POINT('Ctrl Pts',(-0.0694075104800352,-0.0747174017939175,
-0.886904199087995));
#40338=CARTESIAN_POINT('Ctrl Pts',(-0.0387206680177668,-0.0943440645198617,
-0.884787902306448));
#40339=CARTESIAN_POINT('Ctrl Pts',(-0.00680890271086272,-0.096593532974079,
-0.882671605524899));
#40340=CARTESIAN_POINT('Ctrl Pts',(0.0251028625960414,-0.0988430014282963,
-0.880555308743351));
#40341=CARTESIAN_POINT('Ctrl Pts',(0.0582395507475817,-0.0837152756107857,
-0.878439011961802));
#40342=CARTESIAN_POINT('Ctrl Pts',(0.0774440416275778,-0.0581299594437026,
-0.876322715180254));
#40343=CARTESIAN_POINT('Ctrl Pts',(0.096648532507574,-0.0325446432766194,
-0.874206418398705));
#40344=CARTESIAN_POINT('Ctrl Pts',(0.101920826116027,0.00349826324003634,
-0.872090121617157));
#40345=CARTESIAN_POINT('Ctrl Pts',(0.090849311879616,0.0335123007198961,
-0.869973824835609));
#40346=CARTESIAN_POINT('Ctrl Pts',(0.0797777976432054,0.0635263381997554,
-0.86785752805406));
#40347=CARTESIAN_POINT('Ctrl Pts',(0.0523624755619313,0.0875115066428186,
-0.865741231272511));
#40348=CARTESIAN_POINT('Ctrl Pts',(0.0211434440279221,0.0944967012290832,
-0.863624934490963));
#40349=CARTESIAN_POINT('Ctrl Pts',(-0.0100755875060871,0.101481895815348,
-0.861508637709414));
#40350=CARTESIAN_POINT('Ctrl Pts',(-0.0450983284928317,0.0914671165448139,
-0.859392340927867));
#40351=CARTESIAN_POINT('Ctrl Pts',(-0.0679049555418073,0.0690332440307253,
-0.857276044146318));
#40352=CARTESIAN_POINT('Ctrl Pts',(-0.0860544891803395,0.0511803487752086,
-0.855591893327202));
#40353=CARTESIAN_POINT('Ctrl Pts',(-0.096467569784056,0.0254624538886146,
-0.853907742508084));
#40354=CARTESIAN_POINT('Ctrl Pts',(-0.0967028036390754,-8.59090990596172E-5,
-0.852223591688967));
#40355=CARTESIAN_POINT('Origin',(0.,0.,-0.593));
#40356=CARTESIAN_POINT('',(-0.0968069805588836,4.52912843358962E-5,-0.806426408311032));
#40357=CARTESIAN_POINT('',(-0.0967967750279647,5.29324940476346E-5,-0.812223591688966));
#40358=CARTESIAN_POINT('',(-0.096675,-1.1839272930757E-17,-0.593));
#40359=CARTESIAN_POINT('Ctrl Pts',(-0.0968069805588836,4.52912843358962E-5,
-0.806426408311032));
#40360=CARTESIAN_POINT('Ctrl Pts',(-0.096821913186225,0.0026163686460789,
-0.806596369900907));
#40361=CARTESIAN_POINT('Ctrl Pts',(-0.0967283557208207,0.00518634230609915,
-0.806766331490783));
#40362=CARTESIAN_POINT('Ctrl Pts',(-0.096522800338362,0.00774732654152389,
-0.806936293080658));
#40363=CARTESIAN_POINT('Ctrl Pts',(-0.0939633032505456,0.0396357237905355,
-0.809052589862207));
#40364=CARTESIAN_POINT('Ctrl Pts',(-0.0740393367051216,0.0701303755759174,
-0.811168886643756));
#40365=CARTESIAN_POINT('Ctrl Pts',(-0.0458643628784741,0.0852826610246885,
-0.813285183425304));
#40366=CARTESIAN_POINT('Ctrl Pts',(-0.017689389051826,0.10043494647346,
-0.815401480206853));
#40367=CARTESIAN_POINT('Ctrl Pts',(0.0187365920560463,0.10024486558562,
-0.817517776988401));
#40368=CARTESIAN_POINT('Ctrl Pts',(0.0467518981286488,0.0847993636477818,
-0.819634073769949));
#40369=CARTESIAN_POINT('Ctrl Pts',(0.0747672042012515,0.0693538617099438,
-0.821750370551497));
#40370=CARTESIAN_POINT('Ctrl Pts',(0.0943718352385847,0.0386529387221085,
-0.823866667333046));
#40371=CARTESIAN_POINT('Ctrl Pts',(0.0965983969703672,0.00673956648870246,
-0.825982964114595));
#40372=CARTESIAN_POINT('Ctrl Pts',(0.0988249587021496,-0.0251738057447027,
-0.828099260896143));
#40373=CARTESIAN_POINT('Ctrl Pts',(0.0836734511283823,-0.0582996272236781,
-0.830215557677691));
#40374=CARTESIAN_POINT('Ctrl Pts',(0.0580743562328568,-0.0774857483789087,
-0.832331854459239));
#40375=CARTESIAN_POINT('Ctrl Pts',(0.0324752613373307,-0.0966718695341397,
-0.834448151240788));
#40376=CARTESIAN_POINT('Ctrl Pts',(-0.00357142087995465,-0.101918290365625,
-0.836564448022337));
#40377=CARTESIAN_POINT('Ctrl Pts',(-0.033577503981703,-0.0908252348197296,
-0.838680744803886));
#40378=CARTESIAN_POINT('Ctrl Pts',(-0.0635835870834512,-0.0797321792738341,
-0.840797041585434));
#40379=CARTESIAN_POINT('Ctrl Pts',(-0.0875490710696629,-0.0522996473505582,
-0.842913338366981));
#40380=CARTESIAN_POINT('Ctrl Pts',(-0.0945118550278948,-0.0210756094309628,
-0.84502963514853));
#40381=CARTESIAN_POINT('Ctrl Pts',(-0.0960436864568877,-0.0142062360722284,
-0.845495226202697));
#40382=CARTESIAN_POINT('Ctrl Pts',(-0.0967525668347142,-0.00715334928091926,
-0.845960817256864));
#40383=CARTESIAN_POINT('Ctrl Pts',(-0.0966873976231268,-8.74994151896374E-5,
-0.846426408311032));
#40384=CARTESIAN_POINT('Ctrl Pts',(-0.0967028036390754,-8.59090990596172E-5,
-0.852223591688967));
#40385=CARTESIAN_POINT('Ctrl Pts',(-0.0967631636493072,-0.00664151076283559,
-0.851791445726535));
#40386=CARTESIAN_POINT('Ctrl Pts',(-0.0961534001335114,-0.0131859502115887,
-0.851359299764104));
#40387=CARTESIAN_POINT('Ctrl Pts',(-0.094832266671799,-0.0195834870855345,
-0.850927153801673));
#40388=CARTESIAN_POINT('Ctrl Pts',(-0.0883624376416084,-0.0509133799300614,
-0.848810857020124));
#40389=CARTESIAN_POINT('Ctrl Pts',(-0.0648322664700212,-0.0787201998614719,
-0.846694560238576));
#40390=CARTESIAN_POINT('Ctrl Pts',(-0.0350047367470373,-0.0902847726574704,
-0.844578263457028));
#40391=CARTESIAN_POINT('Ctrl Pts',(-0.00517720702405281,-0.101849345453469,
-0.842461966675479));
#40392=CARTESIAN_POINT('Ctrl Pts',(0.0309476812503285,-0.0971716711140548,
-0.84034566989393));
#40393=CARTESIAN_POINT('Ctrl Pts',(0.0568459692467185,-0.0783913741998545,
-0.838229373112382));
#40394=CARTESIAN_POINT('Ctrl Pts',(0.082744257243108,-0.0596110772856547,
-0.836113076330834));
#40395=CARTESIAN_POINT('Ctrl Pts',(0.0984159449615066,-0.0267281577966689,
-0.833996779549286));
#40396=CARTESIAN_POINT('Ctrl Pts',(0.0966926137571569,0.00521634099247394,
-0.831880482767737));
#40397=CARTESIAN_POINT('Ctrl Pts',(0.0949692825528072,0.0371608397816173,
-0.829764185986189));
#40398=CARTESIAN_POINT('Ctrl Pts',(0.0758509324257091,0.0681669178709179,
-0.82764788920464));
#40399=CARTESIAN_POINT('Ctrl Pts',(0.0480825269031277,0.0840520218385643,
-0.825531592423091));
#40400=CARTESIAN_POINT('Ctrl Pts',(0.0203141213805463,0.0999371258062107,
-0.823415295641543));
#40401=CARTESIAN_POINT('Ctrl Pts',(-0.0161043395375181,0.100701255652203,
-0.821298998859995));
#40402=CARTESIAN_POINT('Ctrl Pts',(-0.0445146133599316,0.0859948891850922,
-0.819182702078447));
#40403=CARTESIAN_POINT('Ctrl Pts',(-0.0729248871823449,0.0712885227179818,
-0.817066405296898));
#40404=CARTESIAN_POINT('Ctrl Pts',(-0.0933269739091071,0.0411116599377694,
-0.814950108515349));
#40405=CARTESIAN_POINT('Ctrl Pts',(-0.096388713436468,0.00926756120038876,
-0.812833811733801));
#40406=CARTESIAN_POINT('Ctrl Pts',(-0.0966829908188508,0.00620688345917894,
-0.812630405052189));
#40407=CARTESIAN_POINT('Ctrl Pts',(-0.0968170783214265,0.00313080381600502,
-0.812426998370578));
#40408=CARTESIAN_POINT('Ctrl Pts',(-0.0967967750279647,5.29324940476346E-5,
-0.812223591688966));
#40409=CARTESIAN_POINT('Origin',(0.,0.,-0.593));
#40410=CARTESIAN_POINT('',(-0.0965527474869059,5.80210454589614E-5,-0.766426408311032));
#40411=CARTESIAN_POINT('',(-0.0965440014864236,5.14221950347461E-5,-0.772223591688967));
#40412=CARTESIAN_POINT('',(-0.096675,-1.1839272930757E-17,-0.593));
#40413=CARTESIAN_POINT('Ctrl Pts',(-0.0965527474869059,5.80210454589614E-5,
-0.766426408311032));
#40414=CARTESIAN_POINT('Ctrl Pts',(-0.0966199713755426,0.0123258193606181,
-0.76723192254495));
#40415=CARTESIAN_POINT('Ctrl Pts',(-0.0944522024343605,0.0245707460210818,
-0.768037436778869));
#40416=CARTESIAN_POINT('Ctrl Pts',(-0.0899403163476919,0.0358805176798972,
-0.768842951012787));
#40417=CARTESIAN_POINT('Ctrl Pts',(-0.0780864103558861,0.065594248801902,
-0.770959247794335));
#40418=CARTESIAN_POINT('Ctrl Pts',(-0.0500522249818788,0.0888530682223019,
-0.773075544575884));
#40419=CARTESIAN_POINT('Ctrl Pts',(-0.0186609341388208,0.0950181119090823,
-0.775191841357432));
#40420=CARTESIAN_POINT('Ctrl Pts',(0.0127303567042363,0.101183155595862,
-0.777308138138981));
#40421=CARTESIAN_POINT('Ctrl Pts',(0.0474787530163437,0.0902544235490242,
-0.779424434920529));
#40422=CARTESIAN_POINT('Ctrl Pts',(0.0696899199642036,0.0672308493854064,
-0.781540731702077));
#40423=CARTESIAN_POINT('Ctrl Pts',(0.0919010869120639,0.0442072752217881,
-0.783657028483626));
#40424=CARTESIAN_POINT('Ctrl Pts',(0.101575024495676,0.00908885894138933,
-0.785773325265174));
#40425=CARTESIAN_POINT('Ctrl Pts',(0.0942867571930242,-0.0220608130340657,
-0.787889622046723));
#40426=CARTESIAN_POINT('Ctrl Pts',(0.0869984898903725,-0.0532104850095206,
-0.790005918828271));
#40427=CARTESIAN_POINT('Ctrl Pts',(0.0627480177014573,-0.0803914126800321,
-0.792122215609819));
#40428=CARTESIAN_POINT('Ctrl Pts',(0.0326277985738104,-0.0911707124789926,
-0.794238512391368));
#40429=CARTESIAN_POINT('Ctrl Pts',(0.00250757944616346,-0.101950012277953,
-0.796354809172916));
#40430=CARTESIAN_POINT('Ctrl Pts',(-0.0334823866202151,-0.0963276842053627,
-0.798471105954465));
#40431=CARTESIAN_POINT('Ctrl Pts',(-0.0588798558383005,-0.0768754488127468,
-0.800587402736014));
#40432=CARTESIAN_POINT('Ctrl Pts',(-0.0822376327576704,-0.0589854389467146,
-0.802533737927686));
#40433=CARTESIAN_POINT('Ctrl Pts',(-0.0966359778157342,-0.0293977043556654,
-0.804480073119359));
#40434=CARTESIAN_POINT('Ctrl Pts',(-0.0968069805588836,4.52912843358962E-5,
-0.806426408311032));
#40435=CARTESIAN_POINT('Ctrl Pts',(-0.0967967750279647,5.29324940476346E-5,
-0.812223591688966));
#40436=CARTESIAN_POINT('Ctrl Pts',(-0.0966058374995047,-0.0288921814717637,
-0.810310701589029));
#40437=CARTESIAN_POINT('Ctrl Pts',(-0.0827605504412421,-0.0579957518286451,
-0.808397811489093));
#40438=CARTESIAN_POINT('Ctrl Pts',(-0.0600840974796387,-0.0759379549276761,
-0.806484921389156));
#40439=CARTESIAN_POINT('Ctrl Pts',(-0.0349963496674887,-0.0957880376238121,
-0.804368624607608));
#40440=CARTESIAN_POINT('Ctrl Pts',(0.000900538284770831,-0.101976868321535,
-0.802252327826059));
#40441=CARTESIAN_POINT('Ctrl Pts',(0.0311868976401448,-0.0916736013480633,
-0.800136031044511));
#40442=CARTESIAN_POINT('Ctrl Pts',(0.0614732569955178,-0.0813703343745921,
-0.798019734262962));
#40443=CARTESIAN_POINT('Ctrl Pts',(0.0861490877540057,-0.0545749697299277,
-0.795903437481414));
#40444=CARTESIAN_POINT('Ctrl Pts',(0.0939273678371664,-0.0235440298105936,
-0.793787140699865));
#40445=CARTESIAN_POINT('Ctrl Pts',(0.101705647920327,0.00748691010874134,
-0.791670843918317));
#40446=CARTESIAN_POINT('Ctrl Pts',(0.0925863773281602,0.0427534253027464,
-0.789554547136769));
#40447=CARTESIAN_POINT('Ctrl Pts',(0.0707408202227712,0.0661241871235485,
-0.78743825035522));
#40448=CARTESIAN_POINT('Ctrl Pts',(0.0488952631173822,0.0894949489443506,
-0.785321953573672));
#40449=CARTESIAN_POINT('Ctrl Pts',(0.0143234194987715,0.10096995739195,
-0.783205656792123));
#40450=CARTESIAN_POINT('Ctrl Pts',(-0.0171611331274083,0.0953004054467968,
-0.781089360010575));
#40451=CARTESIAN_POINT('Ctrl Pts',(-0.0486456857535873,0.0896308535016439,
-0.778973063229026));
#40452=CARTESIAN_POINT('Ctrl Pts',(-0.0770429473873355,0.0668167411637396,
-0.776856766447478));
#40453=CARTESIAN_POINT('Ctrl Pts',(-0.0893636686629692,0.0372935180914264,
-0.77474046966593));
#40454=CARTESIAN_POINT('Ctrl Pts',(-0.0942479477031789,0.0255896854646212,
-0.773901510340276));
#40455=CARTESIAN_POINT('Ctrl Pts',(-0.0966057153328721,0.0128314814091803,
-0.773062551014621));
#40456=CARTESIAN_POINT('Ctrl Pts',(-0.0965440014864236,5.14221950347461E-5,
-0.772223591688967));
#40457=CARTESIAN_POINT('Origin',(0.,0.,-0.593));
#40458=CARTESIAN_POINT('',(-0.0965963020766926,-7.83064175312459E-5,-0.726426408311032));
#40459=CARTESIAN_POINT('',(-0.0966095321632848,-8.1873982564944E-5,-0.732223591688966));
#40460=CARTESIAN_POINT('',(-0.096675,-1.1839272930757E-17,-0.593));
#40461=CARTESIAN_POINT('Ctrl Pts',(-0.0965963020766926,-7.83064175312459E-5,
-0.726426408311032));
#40462=CARTESIAN_POINT('Ctrl Pts',(-0.0964291685623488,0.0218439313421801,
-0.727867475188993));
#40463=CARTESIAN_POINT('Ctrl Pts',(-0.0890325024660615,0.0438682325777133,
-0.729308542066955));
#40464=CARTESIAN_POINT('Ctrl Pts',(-0.0753504419047513,0.0608192646984407,
-0.730749608944916));
#40465=CARTESIAN_POINT('Ctrl Pts',(-0.0552574807981732,0.0857129148611408,
-0.732865905726464));
#40466=CARTESIAN_POINT('Ctrl Pts',(-0.0216089613936002,0.0996651681664339,
-0.734982202508012));
#40467=CARTESIAN_POINT('Ctrl Pts',(0.0102038784153586,0.0962940959715852,
-0.737098499289561));
#40468=CARTESIAN_POINT('Ctrl Pts',(0.0420167182243175,0.0929230237767366,
-0.739214796071109));
#40469=CARTESIAN_POINT('Ctrl Pts',(0.0719938784376625,0.0722286260817463,
-0.741331092852657));
#40470=CARTESIAN_POINT('Ctrl Pts',(0.0864234450579025,0.0436767695465677,
-0.743447389634206));
#40471=CARTESIAN_POINT('Ctrl Pts',(0.100853011678142,0.0151249130113896,
-0.745563686415754));
#40472=CARTESIAN_POINT('Ctrl Pts',(0.0997349847052779,-0.0212844023639766,
-0.747679983197303));
#40473=CARTESIAN_POINT('Ctrl Pts',(0.0835807631374022,-0.0488971173697365,
-0.749796279978852));
#40474=CARTESIAN_POINT('Ctrl Pts',(0.0674265415695264,-0.0765098323754965,
-0.7519125767604));
#40475=CARTESIAN_POINT('Ctrl Pts',(0.03623612540664,-0.09532594701165,-0.754028873541948));
#40476=CARTESIAN_POINT('Ctrl Pts',(0.00427638652478659,-0.0967387439033137,
-0.756145170323496));
#40477=CARTESIAN_POINT('Ctrl Pts',(-0.0276833523570661,-0.0981515407949775,
-0.758261467105044));
#40478=CARTESIAN_POINT('Ctrl Pts',(-0.0604124139578854,-0.0821610199421518,
-0.760377763886594));
#40479=CARTESIAN_POINT('Ctrl Pts',(-0.0789401314534932,-0.0560814381039349,
-0.762494060668142));
#40480=CARTESIAN_POINT('Ctrl Pts',(-0.0904157472330977,-0.0399283819630976,
-0.763804843215772));
#40481=CARTESIAN_POINT('Ctrl Pts',(-0.0964433566204278,-0.0199048986054247,
-0.765115625763402));
#40482=CARTESIAN_POINT('Ctrl Pts',(-0.0965527474869059,5.80210454589614E-5,
-0.766426408311032));
#40483=CARTESIAN_POINT('Ctrl Pts',(-0.0965440014864236,5.14221950347461E-5,
-0.772223591688967));
#40484=CARTESIAN_POINT('Ctrl Pts',(-0.0964500405455227,-0.0194065513009297,
-0.770946254233073));
#40485=CARTESIAN_POINT('Ctrl Pts',(-0.0907475142576013,-0.0389151869271784,
-0.769668916777178));
#40486=CARTESIAN_POINT('Ctrl Pts',(-0.0798141682827737,-0.0548303776192502,
-0.768391579321284));
#40487=CARTESIAN_POINT('Ctrl Pts',(-0.0616997657094256,-0.0811987164508894,
-0.766275282539736));
#40488=CARTESIAN_POINT('Ctrl Pts',(-0.0292267796452108,-0.097703060307445,
-0.764158985758187));
#40489=CARTESIAN_POINT('Ctrl Pts',(0.00275125511920654,-0.0967941236016399,
-0.762042688976639));
#40490=CARTESIAN_POINT('Ctrl Pts',(0.0347292898836239,-0.0958851868958348,
-0.759926392195091));
#40491=CARTESIAN_POINT('Ctrl Pts',(0.0662123733482439,-0.0775629696276689,
-0.757810095413542));
#40492=CARTESIAN_POINT('Ctrl Pts',(0.082799764089584,-0.050208274569534,
-0.755693798631993));
#40493=CARTESIAN_POINT('Ctrl Pts',(0.0993871548309243,-0.0228535795113987,
-0.753577501850445));
#40494=CARTESIAN_POINT('Ctrl Pts',(0.101078852848984,0.0135335933367059,
-0.751461205068897));
#40495=CARTESIAN_POINT('Ctrl Pts',(0.0871010551027728,0.0423093130235439,
-0.749344908287348));
#40496=CARTESIAN_POINT('Ctrl Pts',(0.0731232573565615,0.0710850327103816,
-0.7472286115058));
#40497=CARTESIAN_POINT('Ctrl Pts',(0.0434759638460791,0.0922492992359529,
-0.745112314724252));
#40498=CARTESIAN_POINT('Ctrl Pts',(0.0117202035674321,0.0961213222801188,
-0.742996017942703));
#40499=CARTESIAN_POINT('Ctrl Pts',(-0.020035556711215,0.0999933453242847,
-0.740879721161155));
#40500=CARTESIAN_POINT('Ctrl Pts',(-0.0538997837580266,0.0865731248870451,
-0.738763424379606));
#40501=CARTESIAN_POINT('Ctrl Pts',(-0.07438257240678,0.0619992313717728,
-0.736647127598058));
#40502=CARTESIAN_POINT('Ctrl Pts',(-0.0886537829943919,0.0448775779031986,
-0.735172615628361));
#40503=CARTESIAN_POINT('Ctrl Pts',(-0.0964289899211591,0.0223413868496905,
-0.733698103658664));
#40504=CARTESIAN_POINT('Ctrl Pts',(-0.0966095321632848,-8.1873982564944E-5,
-0.732223591688966));
#40505=CARTESIAN_POINT('Origin',(0.,0.,-0.593));
#40506=CARTESIAN_POINT('',(-0.0968316171384256,-1.1157892015598E-5,-0.686426408311032));
#40507=CARTESIAN_POINT('',(-0.09683317566692,-1.75825702407311E-6,-0.692223591688967));
#40508=CARTESIAN_POINT('',(-0.096675,-1.1839272930757E-17,-0.593));
#40509=CARTESIAN_POINT('Ctrl Pts',(-0.0968316171384256,-1.1157892015598E-5,
-0.686426408311032));
#40510=CARTESIAN_POINT('Ctrl Pts',(-0.0967803231635655,0.0313814111628826,
-0.688503027833036));
#40511=CARTESIAN_POINT('Ctrl Pts',(-0.080097610772753,0.0628207796501225,
-0.69057964735504));
#40512=CARTESIAN_POINT('Ctrl Pts',(-0.0540521141943119,0.0803432698166147,
-0.692656266877044));
#40513=CARTESIAN_POINT('Ctrl Pts',(-0.027508975213516,0.0982005562145947,
-0.694772563658592));
#40514=CARTESIAN_POINT('Ctrl Pts',(0.00875814900968967,0.101604073658873,
-0.696888860440141));
#40515=CARTESIAN_POINT('Ctrl Pts',(0.038160239210447,0.08899701229312,-0.699005157221689));
#40516=CARTESIAN_POINT('Ctrl Pts',(0.0675623294112047,0.0763899509273669,
-0.701121454003237));
#40517=CARTESIAN_POINT('Ctrl Pts',(0.0900993855895135,0.0477723107515832,
-0.703237750784786));
#40518=CARTESIAN_POINT('Ctrl Pts',(0.0954626869101027,0.0162341449298691,
-0.705354047566334));
#40519=CARTESIAN_POINT('Ctrl Pts',(0.100825988230692,-0.0153040208918445,
-0.707470344347883));
#40520=CARTESIAN_POINT('Ctrl Pts',(0.0890155346935609,-0.0497627123594873,
-0.709586641129431));
#40521=CARTESIAN_POINT('Ctrl Pts',(0.0654335699408682,-0.0713801091235773,
-0.71170293791098));
#40522=CARTESIAN_POINT('Ctrl Pts',(0.0418516051881752,-0.0929975058876676,
-0.713819234692528));
#40523=CARTESIAN_POINT('Ctrl Pts',(0.00649812921991958,-0.101773607948205,
-0.715935531474077));
#40524=CARTESIAN_POINT('Ctrl Pts',(-0.0244557524109016,-0.0936941205610948,
-0.718051828255625));
#40525=CARTESIAN_POINT('Ctrl Pts',(-0.055409634041722,-0.0856146331739852,
-0.720168125037174));
#40526=CARTESIAN_POINT('Ctrl Pts',(-0.0819639213351086,-0.0606795563392294,
-0.722284421818721));
#40527=CARTESIAN_POINT('Ctrl Pts',(-0.0919723635775106,-0.0302944944117986,
-0.72440071860027));
#40528=CARTESIAN_POINT('Ctrl Pts',(-0.0951656772702392,-0.0205997754977805,
-0.725075948503857));
#40529=CARTESIAN_POINT('Ctrl Pts',(-0.0966746145745388,-0.0103502450175289,
-0.725751178407445));
#40530=CARTESIAN_POINT('Ctrl Pts',(-0.0965963020766926,-7.83064175312459E-5,
-0.726426408311032));
#40531=CARTESIAN_POINT('Ctrl Pts',(-0.0966095321632848,-8.1873982564944E-5,
-0.732223591688966));
#40532=CARTESIAN_POINT('Ctrl Pts',(-0.096688113599906,-0.00984165113600456,
-0.731581806877115));
#40533=CARTESIAN_POINT('Ctrl Pts',(-0.0953279267075589,-0.0195800342671315,
-0.730940022065264));
#40534=CARTESIAN_POINT('Ctrl Pts',(-0.0924383800560967,-0.0288412492993127,
-0.730298237253412));
#40535=CARTESIAN_POINT('Ctrl Pts',(-0.0829100488059648,-0.0593802698618187,
-0.728181940471864));
#40536=CARTESIAN_POINT('Ctrl Pts',(-0.0567520360550064,-0.0847307443935267,
-0.726065643690316));
#40537=CARTESIAN_POINT('Ctrl Pts',(-0.0259293317700408,-0.0932970606316171,
-0.723949346908767));
#40538=CARTESIAN_POINT('Ctrl Pts',(0.00489337251492607,-0.101863376869708,
-0.721833050127219));
#40539=CARTESIAN_POINT('Ctrl Pts',(0.0403807683338999,-0.0936455348141805,
-0.71971675334567));
#40540=CARTESIAN_POINT('Ctrl Pts',(0.0643004935818126,-0.072402474361556,
-0.717600456564122));
#40541=CARTESIAN_POINT('Ctrl Pts',(0.088220218829725,-0.0511594139089317,
-0.715484159782573));
#40542=CARTESIAN_POINT('Ctrl Pts',(0.100572273506576,-0.0168911350592103,
-0.713367863001025));
#40543=CARTESIAN_POINT('Ctrl Pts',(0.0957066790881852,0.0147276388620725,
-0.711251566219477));
#40544=CARTESIAN_POINT('Ctrl Pts',(0.0908410846697948,0.0463464127833544,
-0.709135269437928));
#40545=CARTESIAN_POINT('Ctrl Pts',(0.0687578411561641,0.0753156817761985,
-0.70701897265638));
#40546=CARTESIAN_POINT('Ctrl Pts',(0.0395580900059744,0.0883845534220754,
-0.704902675874831));
#40547=CARTESIAN_POINT('Ctrl Pts',(0.0103583388557835,0.101453425067953,
-0.702786379093283));
#40548=CARTESIAN_POINT('Ctrl Pts',(-0.0259579199309663,0.0986218993668624,
-0.700670082311735));
#40549=CARTESIAN_POINT('Ctrl Pts',(-0.0527791923484877,0.0811851502651922,
-0.698553785530186));
#40550=CARTESIAN_POINT('Ctrl Pts',(-0.0795214802530595,0.063799749701868,
-0.696443720916446));
#40551=CARTESIAN_POINT('Ctrl Pts',(-0.0968246219893057,0.0318950193429899,
-0.694333656302706));
#40552=CARTESIAN_POINT('Ctrl Pts',(-0.09683317566692,-1.75825702407311E-6,
-0.692223591688967));
#40553=CARTESIAN_POINT('Origin',(0.,0.,-0.593));
#40554=CARTESIAN_POINT('',(-0.0966287398315909,8.55332849566889E-5,-0.646426408311032));
#40555=CARTESIAN_POINT('',(-0.0966146360987624,8.30122117530267E-5,-0.652223591688966));
#40556=CARTESIAN_POINT('',(-0.096675,-1.1839272930757E-17,-0.593));
#40557=CARTESIAN_POINT('Ctrl Pts',(-0.0966287398315909,8.55332849566889E-5,
-0.646426408311032));
#40558=CARTESIAN_POINT('Ctrl Pts',(-0.0967060986674926,0.00914259352035314,
-0.64702228369553));
#40559=CARTESIAN_POINT('Ctrl Pts',(-0.0955368666845756,0.0181800678202769,
-0.647618159080028));
#40560=CARTESIAN_POINT('Ctrl Pts',(-0.0930406615301446,0.0268348161114135,
-0.648214034464527));
#40561=CARTESIAN_POINT('Ctrl Pts',(-0.0841751989320309,0.0575728134010026,
-0.650330331246075));
#40562=CARTESIAN_POINT('Ctrl Pts',(-0.0585717042856102,0.0834832223577448,
-0.652446628027624));
#40563=CARTESIAN_POINT('Ctrl Pts',(-0.0279415243004564,0.0927143099713701,
-0.654562924809172));
#40564=CARTESIAN_POINT('Ctrl Pts',(0.00268865568469739,0.101945397584995,
-0.656679221590721));
#40565=CARTESIAN_POINT('Ctrl Pts',(0.0383455210085838,0.0944971638555036,
-0.658795518372269));
#40566=CARTESIAN_POINT('Ctrl Pts',(0.062719192174226,0.0737765205652367,
-0.660911815153817));
#40567=CARTESIAN_POINT('Ctrl Pts',(0.0870928633398687,0.0530558772749696,
-0.663028111935366));
#40568=CARTESIAN_POINT('Ctrl Pts',(0.100183340347266,0.0190628244239271,
-0.665144408716914));
#40569=CARTESIAN_POINT('Ctrl Pts',(0.0960028814078669,-0.0126538063477889,
-0.667260705498463));
#40570=CARTESIAN_POINT('Ctrl Pts',(0.0918224224684676,-0.0443704371195039,
-0.669377002280011));
#40571=CARTESIAN_POINT('Ctrl Pts',(0.0703710275822714,-0.0738106458118936,
-0.671493299061559));
#40572=CARTESIAN_POINT('Ctrl Pts',(0.0414608230385063,-0.0875081265178838,
-0.673609595843108));
#40573=CARTESIAN_POINT('Ctrl Pts',(0.0125506184947407,-0.101205607223874,
-0.675725892624656));
#40574=CARTESIAN_POINT('Ctrl Pts',(-0.0238183957065942,-0.099160359943466,
-0.677842189406205));
#40575=CARTESIAN_POINT('Ctrl Pts',(-0.0510105945979204,-0.082307905406874,
-0.679958486187754));
#40576=CARTESIAN_POINT('Ctrl Pts',(-0.0782027934892469,-0.0654554508702817,
-0.682074782969302));
#40577=CARTESIAN_POINT('Ctrl Pts',(-0.096218177070564,-0.0337957890775055,
-0.68419107975085));
#40578=CARTESIAN_POINT('Ctrl Pts',(-0.0968162919920292,-0.00181043050527611,
-0.686307376532398));
#40579=CARTESIAN_POINT('Ctrl Pts',(-0.0968275057127055,-0.00121075498492486,
-0.686347053791943));
#40580=CARTESIAN_POINT('Ctrl Pts',(-0.0968325971948741,-0.000610964980873346,
-0.686386731051487));
#40581=CARTESIAN_POINT('Ctrl Pts',(-0.0968316171384256,-1.1157892015598E-5,
-0.686426408311032));
#40582=CARTESIAN_POINT('Ctrl Pts',(-0.09683317566692,-1.75825702407311E-6,
-0.692223591688967));
#40583=CARTESIAN_POINT('Ctrl Pts',(-0.0968417798718537,-0.0320869529029069,
-0.69010106273961));
#40584=CARTESIAN_POINT('Ctrl Pts',(-0.0793039408690168,-0.0641639627296817,
-0.687978533790253));
#40585=CARTESIAN_POINT('Ctrl Pts',(-0.052301429073298,-0.0814937561131604,
-0.685856004840896));
#40586=CARTESIAN_POINT('Ctrl Pts',(-0.0253782020311814,-0.0987726657711256,
-0.683739708059347));
#40587=CARTESIAN_POINT('Ctrl Pts',(0.0109540616794619,-0.101390833779945,
-0.681623411277799));
#40588=CARTESIAN_POINT('Ctrl Pts',(0.0400765472079607,-0.0881506785704375,
-0.67950711449625));
#40589=CARTESIAN_POINT('Ctrl Pts',(0.0691990327364591,-0.0749105233609298,
-0.677390817714702));
#40590=CARTESIAN_POINT('Ctrl Pts',(0.0911117400828133,-0.0458120449330938,
-0.675274520933153));
#40591=CARTESIAN_POINT('Ctrl Pts',(0.0957915330844569,-0.0141652376566684,
-0.673158224151605));
#40592=CARTESIAN_POINT('Ctrl Pts',(0.1004713260861,0.0174815696197567,-0.671041927370057));
#40593=CARTESIAN_POINT('Ctrl Pts',(0.0879182047430347,0.0516767057447719,
-0.668925630588508));
#40594=CARTESIAN_POINT('Ctrl Pts',(0.0638741178933472,0.07277890375574,
-0.66680933380696));
#40595=CARTESIAN_POINT('Ctrl Pts',(0.039830031043659,0.0938811017667088,
-0.664693037025411));
#40596=CARTESIAN_POINT('Ctrl Pts',(0.00429497868734867,0.101890361663629,
-0.662576740243863));
#40597=CARTESIAN_POINT('Ctrl Pts',(-0.026476878396567,0.0931431515405931,
-0.660460443462315));
#40598=CARTESIAN_POINT('Ctrl Pts',(-0.0572487354804823,0.084395941417557,
-0.658344146680766));
#40599=CARTESIAN_POINT('Ctrl Pts',(-0.0832573972920026,0.0588922612745646,
-0.656227849899217));
#40600=CARTESIAN_POINT('Ctrl Pts',(-0.0926061887821478,0.0282978014655855,
-0.654111553117669));
#40601=CARTESIAN_POINT('Ctrl Pts',(-0.0953862269904411,0.0191999659516889,
-0.653482232641435));
#40602=CARTESIAN_POINT('Ctrl Pts',(-0.0966930635408328,0.0096519621652146,
-0.6528529121652));
#40603=CARTESIAN_POINT('Ctrl Pts',(-0.0966146360987624,8.30122117530267E-5,
-0.652223591688966));
#40604=CARTESIAN_POINT('Origin',(0.,0.,-0.593));
#40605=CARTESIAN_POINT('',(-0.0965338432881175,-4.16383404607604E-5,-0.606426408311032));
#40606=CARTESIAN_POINT('',(-0.0965410275132817,-4.88435499436115E-5,-0.612223591688966));
#40607=CARTESIAN_POINT('',(-0.096675,-1.1839272930757E-17,-0.593));
#40608=CARTESIAN_POINT('Ctrl Pts',(-0.0965338432881175,-4.16383404607604E-5,
-0.606426408311032));
#40609=CARTESIAN_POINT('Ctrl Pts',(-0.0964609475612972,0.0187219270939628,
-0.607657836339573));
#40610=CARTESIAN_POINT('Ctrl Pts',(-0.0911876223337323,0.0375233571128565,
-0.608889264368114));
#40611=CARTESIAN_POINT('Ctrl Pts',(-0.0809816167434835,0.0530909578300473,
-0.610120692396655));
#40612=CARTESIAN_POINT('Ctrl Pts',(-0.0634418691638409,0.0798449885412464,
-0.612236989178203));
#40613=CARTESIAN_POINT('Ctrl Pts',(-0.0313335139014484,0.0970479462159885,
-0.614353285959752));
#40614=CARTESIAN_POINT('Ctrl Pts',(0.000656700771827244,0.0968309908954595,
-0.616469582741301));
#40615=CARTESIAN_POINT('Ctrl Pts',(0.0326469154451024,0.0966140355749306,
-0.618585879522849));
#40616=CARTESIAN_POINT('Ctrl Pts',(0.0645189895292607,0.0789771672591311,
-0.620702176304397));
#40617=CARTESIAN_POINT('Ctrl Pts',(0.0816942526081138,0.051987701858247,
-0.622818473085946));
#40618=CARTESIAN_POINT('Ctrl Pts',(0.0988695156869669,0.0249982364573629,
-0.624934769867494));
#40619=CARTESIAN_POINT('Ctrl Pts',(0.101347967760515,-0.0113438260286058,
-0.627051066649043));
#40620=CARTESIAN_POINT('Ctrl Pts',(0.0879959350105063,-0.0404151886711796,
-0.629167363430591));
#40621=CARTESIAN_POINT('Ctrl Pts',(0.0746439022604976,-0.0694865513137538,
-0.631283660212139));
#40622=CARTESIAN_POINT('Ctrl Pts',(0.0454613846869319,-0.0912872141129328,
-0.633399956993688));
#40623=CARTESIAN_POINT('Ctrl Pts',(0.0137968171766093,-0.0958452914310114,
-0.635516253775236));
#40624=CARTESIAN_POINT('Ctrl Pts',(-0.0178677503337125,-0.10040336874909,
-0.637632550556785));
#40625=CARTESIAN_POINT('Ctrl Pts',(-0.0520143677807911,-0.0877188605860689,
-0.639748847338333));
#40626=CARTESIAN_POINT('Ctrl Pts',(-0.0730239612294275,-0.063593813693341,
-0.641865144119882));
#40627=CARTESIAN_POINT('Ctrl Pts',(-0.0881179857070617,-0.0462615388345649,
-0.643385565516932));
#40628=CARTESIAN_POINT('Ctrl Pts',(-0.0964313528738214,-0.0230242452602008,
-0.644905986913982));
#40629=CARTESIAN_POINT('Ctrl Pts',(-0.0966287398315909,8.55332849566889E-5,
-0.646426408311032));
#40630=CARTESIAN_POINT('Ctrl Pts',(-0.0966146360987624,8.30122117530267E-5,
-0.652223591688966));
#40631=CARTESIAN_POINT('Ctrl Pts',(-0.0964293255098825,-0.0225267746692927,
-0.650736615383652));
#40632=CARTESIAN_POINT('Ctrl Pts',(-0.0885101440476594,-0.0452535031236791,
-0.649249639078338));
#40633=CARTESIAN_POINT('Ctrl Pts',(-0.0740171277690317,-0.0624350587840144,
-0.647762662773024));
#40634=CARTESIAN_POINT('Ctrl Pts',(-0.0533903540970001,-0.0868882197496698,
-0.645646365991476));
#40635=CARTESIAN_POINT('Ctrl Pts',(-0.0194478855841665,-0.100109302206014,
-0.643530069209927));
#40636=CARTESIAN_POINT('Ctrl Pts',(0.0122845840146836,-0.0960508238596976,
-0.641413772428379));
#40637=CARTESIAN_POINT('Ctrl Pts',(0.0440170536135328,-0.091992345513381,
-0.63929747564683));
#40638=CARTESIAN_POINT('Ctrl Pts',(0.0735395242983992,-0.070654306364404,
-0.637181178865282));
#40639=CARTESIAN_POINT('Ctrl Pts',(0.0873480625364419,-0.0417969824230209,
-0.635064882083734));
#40640=CARTESIAN_POINT('Ctrl Pts',(0.101156600774485,-0.0129396584816366,
-0.632948585302185));
#40641=CARTESIAN_POINT('Ctrl Pts',(0.0992512065657041,0.0234369502521536,
-0.630832288520637));
#40642=CARTESIAN_POINT('Ctrl Pts',(0.0825034301615626,0.0506937449801911,
-0.628715991739088));
#40643=CARTESIAN_POINT('Ctrl Pts',(0.0657556537574214,0.0779505397082283,
-0.62659969495754));
#40644=CARTESIAN_POINT('Ctrl Pts',(0.0341654951579198,0.0960875204305122,
-0.624483398175992));
#40645=CARTESIAN_POINT('Ctrl Pts',(0.00218267324238817,0.0968086138009291,
-0.622367101394443));
#40646=CARTESIAN_POINT('Ctrl Pts',(-0.0298001486731421,0.0975297071713459,
-0.620250804612895));
#40647=CARTESIAN_POINT('Ctrl Pts',(-0.0621756339047028,0.0808349131898973,
-0.618134507831346));
#40648=CARTESIAN_POINT('Ctrl Pts',(-0.0801348457163669,0.0543606316239479,
-0.616018211049797));
#40649=CARTESIAN_POINT('Ctrl Pts',(-0.0908687486736435,0.0385374222218539,
-0.61475333792952));
#40650=CARTESIAN_POINT('Ctrl Pts',(-0.0964528109375644,0.0192207439005784,
-0.613488464809243));
#40651=CARTESIAN_POINT('Ctrl Pts',(-0.0965410275132817,-4.88435499436115E-5,
-0.612223591688966));
#40652=CARTESIAN_POINT('Origin',(0.,0.,-0.593));
#40653=CARTESIAN_POINT('',(-0.0967807988947103,-6.24008650121077E-5,-0.566426408311032));
#40654=CARTESIAN_POINT('',(-0.0967926476771765,-5.56256174443557E-5,-0.572223591688966));
#40655=CARTESIAN_POINT('',(-0.096675,-1.1839272930757E-17,-0.593));
#40656=CARTESIAN_POINT('Ctrl Pts',(-0.0967807988947103,-6.24008650121077E-5,
-0.566426408311032));
#40657=CARTESIAN_POINT('Ctrl Pts',(-0.0965688219293542,0.0282002888768916,
-0.568293388983616));
#40658=CARTESIAN_POINT('Ctrl Pts',(-0.0834609918028184,0.0566341393471626,
-0.5701603696562));
#40659=CARTESIAN_POINT('Ctrl Pts',(-0.0617127749374913,0.0746204091600604,
-0.572027350328784));
#40660=CARTESIAN_POINT('Ctrl Pts',(-0.0370603069005264,0.0950085607226655,
-0.574143647110332));
#40661=CARTESIAN_POINT('Ctrl Pts',(-0.00130569935051607,0.101972487011741,
-0.576259943891881));
#40662=CARTESIAN_POINT('Ctrl Pts',(0.0291964597445464,0.0923268042991058,
-0.578376240673429));
#40663=CARTESIAN_POINT('Ctrl Pts',(0.0596986188396094,0.0826811215864704,
-0.580492537454977));
#40664=CARTESIAN_POINT('Ctrl Pts',(0.0849483294797243,0.0564258298721237,
-0.582608834236526));
#40665=CARTESIAN_POINT('Ctrl Pts',(0.0933960700192532,0.0255704156919484,
-0.584725131018074));
#40666=CARTESIAN_POINT('Ctrl Pts',(0.101843810558782,-0.00528499848822653,
-0.586841427799623));
#40667=CARTESIAN_POINT('Ctrl Pts',(0.0934895809977251,-0.0407405351342299,
-0.588957724581171));
#40668=CARTESIAN_POINT('Ctrl Pts',(0.0721547065196973,-0.0645784049102844,
-0.59107402136272));
#40669=CARTESIAN_POINT('Ctrl Pts',(0.0508198320416695,-0.0884162746863389,
-0.593190318144268));
#40670=CARTESIAN_POINT('Ctrl Pts',(0.0165043126466707,-0.100636477592444,
-0.595306614925816));
#40671=CARTESIAN_POINT('Ctrl Pts',(-0.0150955199455927,-0.095649345691816,
-0.597422911707365));
#40672=CARTESIAN_POINT('Ctrl Pts',(-0.046695352537856,-0.0906622137911875,
-0.599539208488913));
#40673=CARTESIAN_POINT('Ctrl Pts',(-0.0755794983273839,-0.0684677470838248,
-0.601655505270462));
#40674=CARTESIAN_POINT('Ctrl Pts',(-0.0885360012737014,-0.0392179618563158,
-0.60377180205201));
#40675=CARTESIAN_POINT('Ctrl Pts',(-0.0939533910771552,-0.0269880037494673,
-0.604656670805017));
#40676=CARTESIAN_POINT('Ctrl Pts',(-0.0965862240601935,-0.0135245966320609,
-0.605541539558025));
#40677=CARTESIAN_POINT('Ctrl Pts',(-0.0965338432881175,-4.16383404607604E-5,
-0.606426408311032));
#40678=CARTESIAN_POINT('Ctrl Pts',(-0.0965410275132817,-4.88435499436115E-5,
-0.612223591688966));
#40679=CARTESIAN_POINT('Ctrl Pts',(-0.0966004087102398,-0.0130197751282173,
-0.611372168027695));
#40680=CARTESIAN_POINT('Ctrl Pts',(-0.0941696024950817,-0.0259693696638901,
-0.610520744366424));
#40681=CARTESIAN_POINT('Ctrl Pts',(-0.0891430782153712,-0.0378177653336196,
-0.609669320705153));
#40682=CARTESIAN_POINT('Ctrl Pts',(-0.0766491605109436,-0.0672681115747841,
-0.607553023923604));
#40683=CARTESIAN_POINT('Ctrl Pts',(-0.0481183867103214,-0.0899150349066602,
-0.605436727142056));
#40684=CARTESIAN_POINT('Ctrl Pts',(-0.016601076251763,-0.0953995599351676,
-0.603320430360507));
#40685=CARTESIAN_POINT('Ctrl Pts',(0.014916234206795,-0.100884084963675,
-0.601204133578959));
#40686=CARTESIAN_POINT('Ctrl Pts',(0.0494200813232888,-0.0892062116888138,
-0.59908783679741));
#40687=CARTESIAN_POINT('Ctrl Pts',(0.071127990010792,-0.065707539944554,
-0.596971540015862));
#40688=CARTESIAN_POINT('Ctrl Pts',(0.0928358986982952,-0.0422088682002942,
-0.594855243234314));
#40689=CARTESIAN_POINT('Ctrl Pts',(0.101747868956808,-0.00688939798663464,
-0.592738946452765));
#40690=CARTESIAN_POINT('Ctrl Pts',(0.0937874582926693,0.024095319784998,
-0.590622649671217));
#40691=CARTESIAN_POINT('Ctrl Pts',(0.0858270476285311,0.0550800375566302,
-0.588506352889668));
#40692=CARTESIAN_POINT('Ctrl Pts',(0.0609942560417432,0.0817300028862363,
-0.586390056108119));
#40693=CARTESIAN_POINT('Ctrl Pts',(0.0306479013833725,0.0918552007745646,
-0.584273759326571));
#40694=CARTESIAN_POINT('Ctrl Pts',(0.000301546725000868,0.101980398662893,
-0.582157462545023));
#40695=CARTESIAN_POINT('Ctrl Pts',(-0.0355583710049534,0.0955808291099426,
-0.580041165763475));
#40696=CARTESIAN_POINT('Ctrl Pts',(-0.0605290936942883,0.075583732278107,
-0.577924868981926));
#40697=CARTESIAN_POINT('Ctrl Pts',(-0.0829526994788125,0.05762642196031,
-0.576024443217606));
#40698=CARTESIAN_POINT('Ctrl Pts',(-0.0965952956441005,0.0287041121739278,
-0.574124017453286));
#40699=CARTESIAN_POINT('Ctrl Pts',(-0.0967926476771765,-5.56256174443557E-5,
-0.572223591688966));
#40700=CARTESIAN_POINT('Origin',(0.,0.,-0.593));
#40701=CARTESIAN_POINT('',(-0.0967237190630299,8.23214974291983E-5,-0.526426408311032));
#40702=CARTESIAN_POINT('',(-0.0967085211101146,8.50951967561498E-5,-0.532223591688966));
#40703=CARTESIAN_POINT('',(-0.096675,-1.1839272930757E-17,-0.593));
#40704=CARTESIAN_POINT('Ctrl Pts',(-0.0967237190630299,8.23214974291983E-5,
-0.526426408311032));
#40705=CARTESIAN_POINT('Ctrl Pts',(-0.0967766851406952,0.00593821845587171,
-0.52681264484611));
#40706=CARTESIAN_POINT('Ctrl Pts',(-0.0962905307316554,0.0117853401103693,
-0.527198881381188));
#40707=CARTESIAN_POINT('Ctrl Pts',(-0.09523371832439,0.0175274341479589,
-0.527585117916267));
#40708=CARTESIAN_POINT('Ctrl Pts',(-0.0894431509050166,0.0489899552391718,
-0.529701414697815));
#40709=CARTESIAN_POINT('Ctrl Pts',(-0.0665200201184249,0.0772992877172744,
-0.531817711479364));
#40710=CARTESIAN_POINT('Ctrl Pts',(-0.0369496419739366,0.089506402071015,
-0.533934008260912));
#40711=CARTESIAN_POINT('Ctrl Pts',(-0.0073792638294475,0.101713516424756,
-0.536050305042461));
#40712=CARTESIAN_POINT('Ctrl Pts',(0.0288383616729391,0.097818412654134,
-0.538166601824009));
#40713=CARTESIAN_POINT('Ctrl Pts',(0.0551368565792162,0.0796027581196986,
-0.540282898605557));
#40714=CARTESIAN_POINT('Ctrl Pts',(0.0814353514854927,0.0613871035852636,
-0.542399195387106));
#40715=CARTESIAN_POINT('Ctrl Pts',(0.0978147157956604,0.0288508982870171,
-0.544515492168655));
#40716=CARTESIAN_POINT('Ctrl Pts',(0.0967828310716766,-0.00312340574559222,
-0.546631788950203));
#40717=CARTESIAN_POINT('Ctrl Pts',(0.0957509463476929,-0.0350977097782011,
-0.548748085731751));
#40718=CARTESIAN_POINT('Ctrl Pts',(0.0773078125895573,-0.0665101125451723,
-0.550864382513299));
#40719=CARTESIAN_POINT('Ctrl Pts',(0.0498895412279715,-0.0829922028251017,
-0.552980679294848));
#40720=CARTESIAN_POINT('Ctrl Pts',(0.0224712698663842,-0.0994742931050322,
-0.555096976076396));
#40721=CARTESIAN_POINT('Ctrl Pts',(-0.0139221390986548,-0.101026070897919,
-0.557213272857945));
#40722=CARTESIAN_POINT('Ctrl Pts',(-0.0426439022409416,-0.0869377343583631,
-0.559329569639493));
#40723=CARTESIAN_POINT('Ctrl Pts',(-0.0713656653832267,-0.0728493978188077,
-0.561445866421042));
#40724=CARTESIAN_POINT('Ctrl Pts',(-0.0924157827027609,-0.0431209469468107,
-0.56356216320259));
#40725=CARTESIAN_POINT('Ctrl Pts',(-0.0961656771005684,-0.0113505330927453,
-0.565678459984138));
#40726=CARTESIAN_POINT('Ctrl Pts',(-0.0966074436280423,-0.00760773291871241,
-0.565927776093103));
#40727=CARTESIAN_POINT('Ctrl Pts',(-0.0968091062430234,-0.0038365930346435,
-0.566177092202067));
#40728=CARTESIAN_POINT('Ctrl Pts',(-0.0967807988947103,-6.24008650121077E-5,
-0.566426408311032));
#40729=CARTESIAN_POINT('Ctrl Pts',(-0.0967926476771765,-5.56256174443557E-5,
-0.572223591688966));
#40730=CARTESIAN_POINT('Ctrl Pts',(-0.0968150650664437,-0.00332246927364548,
-0.572007720671738));
#40731=CARTESIAN_POINT('Ctrl Pts',(-0.0966640000047558,-0.00658721528194418,
-0.571791849654509));
#40732=CARTESIAN_POINT('Ctrl Pts',(-0.0963326163565946,-0.00983355451673743,
-0.57157597863728));
#40733=CARTESIAN_POINT('Ctrl Pts',(-0.0930838886808508,-0.0416591203690247,
-0.569459681855732));
#40734=CARTESIAN_POINT('Ctrl Pts',(-0.0725049056806487,-0.0717156279628795,
-0.567343385074184));
#40735=CARTESIAN_POINT('Ctrl Pts',(-0.0440087419449873,-0.0862548688536479,
-0.565227088292636));
#40736=CARTESIAN_POINT('Ctrl Pts',(-0.015512578209325,-0.100794109744417,
-0.563110791511087));
#40737=CARTESIAN_POINT('Ctrl Pts',(0.020900766261797,-0.0998160839320984,
-0.560994494729539));
#40738=CARTESIAN_POINT('Ctrl Pts',(0.0485753893016762,-0.0837681521983809,
-0.55887819794799));
#40739=CARTESIAN_POINT('Ctrl Pts',(0.0762500123415555,-0.0677202204646633,
-0.556761901166442));
#40740=CARTESIAN_POINT('Ctrl Pts',(0.095185913950192,-0.0366023828095467,
-0.554645604384894));
#40741=CARTESIAN_POINT('Ctrl Pts',(0.0967215847492896,-0.00464831282579854,
-0.552529307603345));
#40742=CARTESIAN_POINT('Ctrl Pts',(0.0982572555483871,0.0273057571579487,
-0.550413010821796));
#40743=CARTESIAN_POINT('Ctrl Pts',(0.0823926955379466,0.0600960594703274,
-0.548296714040247));
#40744=CARTESIAN_POINT('Ctrl Pts',(0.0563845454712289,0.0787239150483727,
-0.546180417258699));
#40745=CARTESIAN_POINT('Ctrl Pts',(0.0303763954045105,0.0973517706264184,
-0.544064120477151));
#40746=CARTESIAN_POINT('Ctrl Pts',(-0.00577534471848571,0.10181717947013,
-0.541947823695603));
#40747=CARTESIAN_POINT('Ctrl Pts',(-0.0355344337095269,0.0900776098122266,
-0.539831526914055));
#40748=CARTESIAN_POINT('Ctrl Pts',(-0.0652935227005681,0.0783380401543233,
-0.537715230132506));
#40749=CARTESIAN_POINT('Ctrl Pts',(-0.0886599605596542,0.0503934919948053,
-0.535598933350957));
#40750=CARTESIAN_POINT('Ctrl Pts',(-0.0949456572852223,0.0190261381057114,
-0.533482636569409));
#40751=CARTESIAN_POINT('Ctrl Pts',(-0.096192170274538,0.0128056957633096,
-0.533062954942594));
#40752=CARTESIAN_POINT('Ctrl Pts',(-0.096766955217955,0.00645064599455275,
-0.53264327331578));
#40753=CARTESIAN_POINT('Ctrl Pts',(-0.0967085211101146,8.50951967561498E-5,
-0.532223591688966));
#40754=CARTESIAN_POINT('Origin',(0.,0.,-0.593));
#40755=CARTESIAN_POINT('',(-0.0965172713955322,9.07121298592689E-6,-0.486426408311032));
#40756=CARTESIAN_POINT('',(-0.0965164910401789,7.28318461152001E-7,-0.492223591688966));
#40757=CARTESIAN_POINT('',(-0.096675,-1.1839272930757E-17,-0.593));
#40758=CARTESIAN_POINT('Ctrl Pts',(-0.0965172713955322,9.07121298592689E-6,
-0.486426408311032));
#40759=CARTESIAN_POINT('Ctrl Pts',(-0.0965303204669342,0.0155849964339054,
-0.487448197490153));
#40760=CARTESIAN_POINT('Ctrl Pts',(-0.0929763058240226,0.0311553037760087,
-0.488469986669274));
#40761=CARTESIAN_POINT('Ctrl Pts',(-0.0858230972773667,0.0448449331298415,
-0.489491775848395));
#40762=CARTESIAN_POINT('Ctrl Pts',(-0.0710076025213427,0.0731984517754618,
-0.491608072629944));
#40763=CARTESIAN_POINT('Ctrl Pts',(-0.0407525168478783,0.0934843587383312,
-0.493724369411492));
#40764=CARTESIAN_POINT('Ctrl Pts',(-0.00889688070606006,0.0964236359374735,
-0.495840666193041));
#40765=CARTESIAN_POINT('Ctrl Pts',(0.0229587554357591,0.0993629131366158,
-0.497956962974589));
#40766=CARTESIAN_POINT('Ctrl Pts',(0.0564149420459315,0.08495556057203,
-0.500073259756137));
#40767=CARTESIAN_POINT('Ctrl Pts',(0.0761684165666363,0.0597916747669077,
-0.502189556537686));
#40768=CARTESIAN_POINT('Ctrl Pts',(0.0959218910873405,0.034627788961786,
-0.504305853319234));
#40769=CARTESIAN_POINT('Ctrl Pts',(0.101972653518578,-0.00129263008387249,
-0.506422150100783));
#40770=CARTESIAN_POINT('Ctrl Pts',(0.091553012274957,-0.0315391502276436,
-0.508538446882331));
#40771=CARTESIAN_POINT('Ctrl Pts',(0.081133371031336,-0.0617856703714156,
-0.510654743663879));
#40772=CARTESIAN_POINT('Ctrl Pts',(0.0542433261128582,-0.0863582916133,
-0.512771040445428));
#40773=CARTESIAN_POINT('Ctrl Pts',(0.0231827078132096,-0.094017201150362,
-0.514887337226976));
#40774=CARTESIAN_POINT('Ctrl Pts',(-0.00787791048643809,-0.101676110687424,
-0.517003634008525));
#40775=CARTESIAN_POINT('Ctrl Pts',(-0.0431091021672566,-0.0924213085196625,
-0.519119930790073));
#40776=CARTESIAN_POINT('Ctrl Pts',(-0.0663956959815876,-0.0704860525836203,
-0.521236227571622));
#40777=CARTESIAN_POINT('Ctrl Pts',(-0.0854323502850516,-0.0525541090953691,
-0.522966287818092));
#40778=CARTESIAN_POINT('Ctrl Pts',(-0.0964864693544764,-0.026147860308577,
-0.524696348064562));
#40779=CARTESIAN_POINT('Ctrl Pts',(-0.0967237190630299,8.23214974291983E-5,
-0.526426408311032));
#40780=CARTESIAN_POINT('Ctrl Pts',(-0.0967085211101146,8.50951967561498E-5,
-0.532223591688966));
#40781=CARTESIAN_POINT('Ctrl Pts',(-0.0964722939641516,-0.0256484353219682,
-0.530526976534232));
#40782=CARTESIAN_POINT('Ctrl Pts',(-0.0858874872503391,-0.0515535821784303,
-0.528830361379498));
#40783=CARTESIAN_POINT('Ctrl Pts',(-0.0674983073426272,-0.0694309028777585,
-0.527133746224764));
#40784=CARTESIAN_POINT('Ctrl Pts',(-0.0445603050824128,-0.091730430353467,
-0.525017449443216));
#40785=CARTESIAN_POINT('Ctrl Pts',(-0.00947934496993338,-0.101539325686214,
-0.522901152661667));
#40786=CARTESIAN_POINT('Ctrl Pts',(0.0216981194752549,-0.0943708820546786,
-0.520784855880119));
#40787=CARTESIAN_POINT('Ctrl Pts',(0.0528755839204423,-0.0872024384231437,
-0.51866855909857));
#40788=CARTESIAN_POINT('Ctrl Pts',(0.0801495526983388,-0.0630566558273281,
-0.516552262317022));
#40789=CARTESIAN_POINT('Ctrl Pts',(0.0910445841196321,-0.0329781059344485,
-0.514435965535473));
#40790=CARTESIAN_POINT('Ctrl Pts',(0.101939615540926,-0.0028995560415681,
-0.512319668753925));
#40791=CARTESIAN_POINT('Ctrl Pts',(0.0964557096056154,0.0331117611483767,
-0.510203371972377));
#40792=CARTESIAN_POINT('Ctrl Pts',(0.0771012709130743,0.0585838355873803,
-0.508087075190828));
#40793=CARTESIAN_POINT('Ctrl Pts',(0.0577468322205332,0.0840559100263839,
-0.50597077840928));
#40794=CARTESIAN_POINT('Ctrl Pts',(0.0245218607707614,0.0989887417144463,
-0.503854481627731));
#40795=CARTESIAN_POINT('Ctrl Pts',(-0.00737614147654734,0.0965518736506882,
-0.501738184846183));
#40796=CARTESIAN_POINT('Ctrl Pts',(-0.0392741437238552,0.0941150055869301,
-0.499621888064634));
#40797=CARTESIAN_POINT('Ctrl Pts',(-0.0698451767686999,0.0743084377713525,
-0.497505591283086));
#40798=CARTESIAN_POINT('Ctrl Pts',(-0.0851056820304146,0.0461919327878629,
-0.495389294501538));
#40799=CARTESIAN_POINT('Ctrl Pts',(-0.0927149210951618,0.0321723964477871,
-0.494334060230681));
#40800=CARTESIAN_POINT('Ctrl Pts',(-0.0965175816304359,0.0160868027612428,
-0.493278825959824));
#40801=CARTESIAN_POINT('Ctrl Pts',(-0.0965165001841129,7.28276446517835E-7,
-0.492223591688966));
#40802=CARTESIAN_POINT('Origin',(0.,0.,-0.593));
#40803=CARTESIAN_POINT('',(-0.096690457956298,-8.72527295337211E-5,-0.446426408311032));
#40804=CARTESIAN_POINT('',(-0.0967058503150131,-8.54906923442515E-5,-0.452223591688966));
#40805=CARTESIAN_POINT('',(-0.096675,-1.1839272930757E-17,-0.593));
#40806=CARTESIAN_POINT('Ctrl Pts',(-0.096690457956298,-8.72527295337211E-5,
-0.446426408311032));
#40807=CARTESIAN_POINT('Ctrl Pts',(-0.0964584083749974,0.0250626678574959,
-0.448083750134195));
#40808=CARTESIAN_POINT('Ctrl Pts',(-0.0864088916390611,0.0503769466530735,
-0.449741091957359));
#40809=CARTESIAN_POINT('Ctrl Pts',(-0.0687716419790343,0.0681698856769454,
-0.451398433780523));
#40810=CARTESIAN_POINT('Ctrl Pts',(-0.0462502440578617,0.0908900868232714,
-0.453514730562072));
#40811=CARTESIAN_POINT('Ctrl Pts',(-0.0113568151501427,0.101346513051999,
-0.455631027343621));
#40812=CARTESIAN_POINT('Ctrl Pts',(0.0199479702554438,0.0947562691139126,
-0.457747324125169));
#40813=CARTESIAN_POINT('Ctrl Pts',(0.0512527556610312,0.0881660251758255,
-0.459863620906718));
#40814=CARTESIAN_POINT('Ctrl Pts',(0.0789688975644853,0.0645291110709228,
-0.461979917688266));
#40815=CARTESIAN_POINT('Ctrl Pts',(0.0904186989652336,0.0346573358920554,
-0.464096214469814));
#40816=CARTESIAN_POINT('Ctrl Pts',(0.101868500365982,0.00478556071318895,
-0.466212511251362));
#40817=CARTESIAN_POINT('Ctrl Pts',(0.097051961264024,-0.0313210755396426,
-0.468328808032911));
#40818=CARTESIAN_POINT('Ctrl Pts',(0.0781722246342648,-0.0571469627314554,
-0.47044510481446));
#40819=CARTESIAN_POINT('Ctrl Pts',(0.0592924880045052,-0.0829728499232685,
-0.472561401596008));
#40820=CARTESIAN_POINT('Ctrl Pts',(0.026349553846944,-0.0985179880540636,
-0.474677698377556));
#40821=CARTESIAN_POINT('Ctrl Pts',(-0.00558808313182638,-0.0966718437840723,
-0.476793995159105));
#40822=CARTESIAN_POINT('Ctrl Pts',(-0.0375257201105967,-0.094825699514081,
-0.478910291940653));
#40823=CARTESIAN_POINT('Ctrl Pts',(-0.0684580599105757,-0.0755882728433033,
-0.481026588722201));
#40824=CARTESIAN_POINT('Ctrl Pts',(-0.0842362778912744,-0.0477589943437285,
-0.48314288550375));
#40825=CARTESIAN_POINT('Ctrl Pts',(-0.0923964658588589,-0.033366231876092,
-0.484237393106177));
#40826=CARTESIAN_POINT('Ctrl Pts',(-0.0965032936512519,-0.0166753573535768,
-0.485331900708604));
#40827=CARTESIAN_POINT('Ctrl Pts',(-0.0965172713955322,9.07121298592689E-6,
-0.486426408311032));
#40828=CARTESIAN_POINT('Ctrl Pts',(-0.0965165001841129,7.28276446517835E-7,
-0.492223591688966));
#40829=CARTESIAN_POINT('Ctrl Pts',(-0.0965154127647765,-0.0161741923562409,
-0.491162529178275));
#40830=CARTESIAN_POINT('Ctrl Pts',(-0.0926684498905901,-0.0323495991129097,
-0.490101466667584));
#40831=CARTESIAN_POINT('Ctrl Pts',(-0.084978495369719,-0.0464255004629906,
-0.489040404156892));
#40832=CARTESIAN_POINT('Ctrl Pts',(-0.0696408259687238,-0.0744999865789511,
-0.486924107375344));
#40833=CARTESIAN_POINT('Ctrl Pts',(-0.0390155096881494,-0.0942225166594689,
-0.484807810593795));
#40834=CARTESIAN_POINT('Ctrl Pts',(-0.0071109349142395,-0.0965717679924415,
-0.482691513812247));
#40835=CARTESIAN_POINT('Ctrl Pts',(0.0247936398596695,-0.098921019325414,
-0.480575217030698));
#40836=CARTESIAN_POINT('Ctrl Pts',(0.0579774731269135,-0.0838969919108423,
-0.47845892024915));
#40837=CARTESIAN_POINT('Ctrl Pts',(0.0772618800277791,-0.0583718567728794,
-0.476342623467602));
#40838=CARTESIAN_POINT('Ctrl Pts',(0.0965462869286451,-0.0328467216349161,
-0.474226326686053));
#40839=CARTESIAN_POINT('Ctrl Pts',(0.101931267463132,0.00317952122643966,
-0.472110029904505));
#40840=CARTESIAN_POINT('Ctrl Pts',(0.0909536667012348,0.033228034581377,
-0.469993733122956));
#40841=CARTESIAN_POINT('Ctrl Pts',(0.0799760659393374,0.0632765479363147,
-0.467877436341408));
#40842=CARTESIAN_POINT('Ctrl Pts',(0.052635883881056,0.0873473317848345,
-0.465761139559859));
#40843=CARTESIAN_POINT('Ctrl Pts',(0.0214388489673388,0.0944301197896949,
-0.463644842778311));
#40844=CARTESIAN_POINT('Ctrl Pts',(-0.00975818594637752,0.101512907794555,
-0.461528545996763));
#40845=CARTESIAN_POINT('Ctrl Pts',(-0.0448120737155289,0.0916076999557566,
-0.459412249215214));
#40846=CARTESIAN_POINT('Ctrl Pts',(-0.0676887440363411,0.0692452575944605,
-0.457295952433666));
#40847=CARTESIAN_POINT('Ctrl Pts',(-0.0859657528056922,0.0513790843529079,
-0.455605165518766));
#40848=CARTESIAN_POINT('Ctrl Pts',(-0.0964700478136312,0.025561462546613,
-0.453914378603866));
#40849=CARTESIAN_POINT('Ctrl Pts',(-0.0967058503150131,-8.54906923442515E-5,
-0.452223591688966));
#40850=CARTESIAN_POINT('Origin',(0.,0.,-0.593));
#40851=CARTESIAN_POINT('',(-0.0968050622971842,4.68532484065691E-5,-0.406426408311032));
#40852=CARTESIAN_POINT('',(-0.0967945983128168,5.43772629733152E-5,-0.412223591688966));
#40853=CARTESIAN_POINT('',(-0.096675,-1.1839272930757E-17,-0.593));
#40854=CARTESIAN_POINT('Ctrl Pts',(-0.0968050622971842,4.68532484065691E-5,
-0.406426408311032));
#40855=CARTESIAN_POINT('Ctrl Pts',(-0.0968210205998854,0.00271845753054062,
-0.40660300599669));
#40856=CARTESIAN_POINT('Ctrl Pts',(-0.0967200026210178,0.00538883683724322,
-0.406779603682348));
#40857=CARTESIAN_POINT('Ctrl Pts',(-0.0964981010810641,0.00804913296256427,
-0.406956201368007));
#40858=CARTESIAN_POINT('Ctrl Pts',(-0.0938388957065765,0.0399293702770765,
-0.409072498149555));
#40859=CARTESIAN_POINT('Ctrl Pts',(-0.0738196642753906,0.0703615670975442,
-0.411188794931103));
#40860=CARTESIAN_POINT('Ctrl Pts',(-0.0455974442696008,0.0854256702038734,
-0.413305091712652));
#40861=CARTESIAN_POINT('Ctrl Pts',(-0.0173752242638107,0.100489773310203,
-0.4154213884942));
#40862=CARTESIAN_POINT('Ctrl Pts',(0.0190499843165828,0.100185782702395,
-0.417537685275749));
#40863=CARTESIAN_POINT('Ctrl Pts',(0.0470168525184595,0.0846527473444171,
-0.419653982057297));
#40864=CARTESIAN_POINT('Ctrl Pts',(0.0749837207203371,0.0691197119864384,
-0.421770278838846));
#40865=CARTESIAN_POINT('Ctrl Pts',(0.0944922485436957,0.0383576318782866,
-0.423886575620394));
#40866=CARTESIAN_POINT('Ctrl Pts',(0.0966190004853783,0.00643745282753642,
-0.426002872401943));
#40867=CARTESIAN_POINT('Ctrl Pts',(0.0987457524270609,-0.0254827262232124,
-0.428119169183491));
#40868=CARTESIAN_POINT('Ctrl Pts',(0.0834907284870702,-0.0585610042165598,
-0.43023546596504));
#40869=CARTESIAN_POINT('Ctrl Pts',(0.0578317602814135,-0.0776669785459265,
-0.432351762746588));
#40870=CARTESIAN_POINT('Ctrl Pts',(0.0321727920757572,-0.096772952875293,
-0.434468059528136));
#40871=CARTESIAN_POINT('Ctrl Pts',(-0.00389012039556526,-0.101906623540679,
-0.436584356309685));
#40872=CARTESIAN_POINT('Ctrl Pts',(-0.0338613667816545,-0.0907197877718999,
-0.438700653091233));
#40873=CARTESIAN_POINT('Ctrl Pts',(-0.063832613167745,-0.0795329520031206,
-0.440816949872781));
#40874=CARTESIAN_POINT('Ctrl Pts',(-0.0877121934686019,-0.0520256098001765,
-0.44293324665433));
#40875=CARTESIAN_POINT('Ctrl Pts',(-0.0945773001517176,-0.0207799506667414,
-0.445049543435878));
#40876=CARTESIAN_POINT('Ctrl Pts',(-0.0960661153214635,-0.0140037979492643,
-0.445508498394263));
#40877=CARTESIAN_POINT('Ctrl Pts',(-0.0967547176669023,-0.00705182732426255,
-0.445967453352647));
#40878=CARTESIAN_POINT('Ctrl Pts',(-0.096690457956298,-8.72527295337211E-5,
-0.446426408311032));
#40879=CARTESIAN_POINT('Ctrl Pts',(-0.0967058503150131,-8.54906923442515E-5,
-0.452223591688966));
#40880=CARTESIAN_POINT('Ctrl Pts',(-0.0967651932694884,-0.00653990050382228,
-0.451798081822318));
#40881=CARTESIAN_POINT('Ctrl Pts',(-0.0961741846374927,-0.0129835010778726,
-0.451372571955669));
#40882=CARTESIAN_POINT('Ctrl Pts',(-0.0948930440917267,-0.019286833631939,
-0.450947062089021));
#40883=CARTESIAN_POINT('Ctrl Pts',(-0.0885212209538268,-0.0506368056132461,
-0.448830765307472));
#40884=CARTESIAN_POINT('Ctrl Pts',(-0.0650781218055549,-0.0785170726920666,
-0.446714468525924));
#40885=CARTESIAN_POINT('Ctrl Pts',(-0.0352869024451259,-0.090174865036598,
-0.444598171744375));
#40886=CARTESIAN_POINT('Ctrl Pts',(-0.00549568308469609,-0.10183265738113,
-0.442481874962827));
#40887=CARTESIAN_POINT('Ctrl Pts',(0.0306436564878915,-0.0972679749913715,
-0.440365578181279));
#40888=CARTESIAN_POINT('Ctrl Pts',(0.0566005472454594,-0.0785687585497888,
-0.43824928139973));
#40889=CARTESIAN_POINT('Ctrl Pts',(0.0825574380030276,-0.0598695421082059,
-0.436132984618182));
#40890=CARTESIAN_POINT('Ctrl Pts',(0.0983318799455758,-0.0270357916147993,
-0.434016687836633));
#40891=CARTESIAN_POINT('Ctrl Pts',(0.0967084534090917,0.00491394014636167,
-0.431900391055085));
#40892=CARTESIAN_POINT('Ctrl Pts',(0.0950850268726077,0.0368636719075213,
-0.429784094273536));
#40893=CARTESIAN_POINT('Ctrl Pts',(0.0760637318570921,0.0679293849364347,
-0.427667797491988));
#40894=CARTESIAN_POINT('Ctrl Pts',(0.048345137713258,0.0839012480719245,
-0.42555150071044));
#40895=CARTESIAN_POINT('Ctrl Pts',(0.0206265435694232,0.0998731112074149,
-0.423435203928891));
#40896=CARTESIAN_POINT('Ctrl Pts',(-0.015789349702731,0.100751124449481,
-0.421318907147343));
#40897=CARTESIAN_POINT('Ctrl Pts',(-0.0442454740842226,0.0861336739701893,
-0.419202610365794));
#40898=CARTESIAN_POINT('Ctrl Pts',(-0.0727015984657142,0.0715162234908976,
-0.417086313584246));
#40899=CARTESIAN_POINT('Ctrl Pts',(-0.0931979539565437,0.0414033092902477,
-0.414970016802697));
#40900=CARTESIAN_POINT('Ctrl Pts',(-0.0963592607853087,0.00956894087396099,
-0.412853720021149));
#40901=CARTESIAN_POINT('Ctrl Pts',(-0.0966730209688041,0.00640937496758658,
-0.412643677243755));
#40902=CARTESIAN_POINT('Ctrl Pts',(-0.0968160206487383,0.00323285171690641,
-0.41243363446636));
#40903=CARTESIAN_POINT('Ctrl Pts',(-0.0967945983128168,5.43772629733152E-5,
-0.412223591688966));
#40904=CARTESIAN_POINT('Origin',(0.,0.,-0.593));
#40905=CARTESIAN_POINT('',(-0.0965509256710446,5.67507499378977E-5,-0.366426408311032));
#40906=CARTESIAN_POINT('',(-0.0965423984694297,5.0056945484775E-5,-0.372223591688966));
#40907=CARTESIAN_POINT('',(-0.096675,-1.1839272930757E-17,-0.593));
#40908=CARTESIAN_POINT('Ctrl Pts',(-0.0965509256710446,5.67507499378977E-5,
-0.366426408311032));
#40909=CARTESIAN_POINT('Ctrl Pts',(-0.0966171433328029,0.0124262003756307,
-0.367238558640733));
#40910=CARTESIAN_POINT('Ctrl Pts',(-0.0944123650341302,0.0247729380575116,
-0.368050708970434));
#40911=CARTESIAN_POINT('Ctrl Pts',(-0.0898276716852722,0.036161601918378,
-0.368862859300135));
#40912=CARTESIAN_POINT('Ctrl Pts',(-0.0778809034285336,0.0658381184368829,
-0.370979156081684));
#40913=CARTESIAN_POINT('Ctrl Pts',(-0.0497741205849931,0.0890091561478041,
-0.373095452863232));
#40914=CARTESIAN_POINT('Ctrl Pts',(-0.0183637040244166,0.0950760034299082,
-0.37521174964478));
#40915=CARTESIAN_POINT('Ctrl Pts',(0.0130467125361599,0.101142850712012,
-0.377328046426329));
#40916=CARTESIAN_POINT('Ctrl Pts',(0.0477607628137719,0.0901055075652994,
-0.379444343207877));
#40917=CARTESIAN_POINT('Ctrl Pts',(0.0698998222648158,0.0670125876313357,
-0.381560639989425));
#40918=CARTESIAN_POINT('Ctrl Pts',(0.0920388817158606,0.043919667697371,
-0.383676936770974));
#40919=CARTESIAN_POINT('Ctrl Pts',(0.101602950340336,0.00877117097615361,
-0.385793233552523));
#40920=CARTESIAN_POINT('Ctrl Pts',(0.0942173080009238,-0.0223555569548012,
-0.387909530334071));
#40921=CARTESIAN_POINT('Ctrl Pts',(0.086831665661512,-0.0534822848857547,
-0.39002582711562));
#40922=CARTESIAN_POINT('Ctrl Pts',(0.0624963123582147,-0.0805872440264466,
-0.392142123897168));
#40923=CARTESIAN_POINT('Ctrl Pts',(0.0323425316822245,-0.0912722997304472,
-0.394258420678716));
#40924=CARTESIAN_POINT('Ctrl Pts',(0.00218875100623434,-0.101957355434448,
-0.396374717460265));
#40925=CARTESIAN_POINT('Ctrl Pts',(-0.0337834570424483,-0.0962225077017568,
-0.398491014241813));
#40926=CARTESIAN_POINT('Ctrl Pts',(-0.0591199714078947,-0.0766909449311324,
-0.400607311023361));
#40927=CARTESIAN_POINT('Ctrl Pts',(-0.0823422408155461,-0.0587892238786714,
-0.402547010119251));
#40928=CARTESIAN_POINT('Ctrl Pts',(-0.0966297808080416,-0.029297293541015,
-0.404486709215142));
#40929=CARTESIAN_POINT('Ctrl Pts',(-0.0968050622971842,4.68532484065691E-5,
-0.406426408311032));
#40930=CARTESIAN_POINT('Ctrl Pts',(-0.0967945983128168,5.43772629733152E-5,
-0.412223591688966));
#40931=CARTESIAN_POINT('Ctrl Pts',(-0.0966001788039178,-0.0287920307405604,
-0.410317337684812));
#40932=CARTESIAN_POINT('Ctrl Pts',(-0.0828630361045588,-0.057799150832469,
-0.408411083680658));
#40933=CARTESIAN_POINT('Ctrl Pts',(-0.0603212754475115,-0.0757496897480507,
-0.406504829676504));
#40934=CARTESIAN_POINT('Ctrl Pts',(-0.0352957251142473,-0.0956781293218542,
-0.404388532894955));
#40935=CARTESIAN_POINT('Ctrl Pts',(0.000581633718982209,-0.101979185837537,
-0.402272236113407));
#40936=CARTESIAN_POINT('Ctrl Pts',(0.0309000651693513,-0.0917706801820185,
-0.400155939331858));
#40937=CARTESIAN_POINT('Ctrl Pts',(0.0612184966197203,-0.0815621745265001,
-0.39803964255031));
#40938=CARTESIAN_POINT('Ctrl Pts',(0.0859780006872285,-0.0548441066997805,
-0.395923345768761));
#40939=CARTESIAN_POINT('Ctrl Pts',(0.0938532821144865,-0.0238376426032253,
-0.393807048987213));
#40940=CARTESIAN_POINT('Ctrl Pts',(0.101728563541744,0.00716882149332862,
-0.391690752205665));
#40941=CARTESIAN_POINT('Ctrl Pts',(0.0927196223287525,0.0424636818597185,
-0.389574455424117));
#40942=CARTESIAN_POINT('Ctrl Pts',(0.0709472566512509,0.0659026444249548,
-0.387458158642568));
#40943=CARTESIAN_POINT('Ctrl Pts',(0.0491748909737483,0.089341606990192,
-0.38534186186102));
#40944=CARTESIAN_POINT('Ctrl Pts',(0.0146391008317351,0.100924671754276,
-0.383225565079471));
#40945=CARTESIAN_POINT('Ctrl Pts',(-0.0168630275634053,0.0953536054375309,
-0.381109268297923));
#40946=CARTESIAN_POINT('Ctrl Pts',(-0.0483651559585449,0.0897825391207864,
-0.378992971516374));
#40947=CARTESIAN_POINT('Ctrl Pts',(-0.0768336226068113,0.0670573417232148,
-0.376876674734826));
#40948=CARTESIAN_POINT('Ctrl Pts',(-0.0892466081115938,0.0375727921389412,
-0.374760377953277));
#40949=CARTESIAN_POINT('Ctrl Pts',(-0.0942063868159446,0.0257918357300971,
-0.37391478253184));
#40950=CARTESIAN_POINT('Ctrl Pts',(-0.0966028891884939,0.0129317408436426,
-0.373069187110403));
#40951=CARTESIAN_POINT('Ctrl Pts',(-0.0965423984694297,5.0056945484775E-5,
-0.372223591688966));
#40952=CARTESIAN_POINT('Origin',(0.,0.,-0.593));
#40953=CARTESIAN_POINT('',(-0.0965988706096985,-7.90725476241677E-5,-0.326426408311032));
#40954=CARTESIAN_POINT('',(-0.0966122385588212,-8.24931776182297E-5,-0.332223591688966));
#40955=CARTESIAN_POINT('',(-0.096675,-1.1839272930757E-17,-0.593));
#40956=CARTESIAN_POINT('Ctrl Pts',(-0.0965988706096985,-7.90725476241677E-5,
-0.326426408311032));
#40957=CARTESIAN_POINT('Ctrl Pts',(-0.0964290112854852,0.0219426387689453,
-0.327874111284776));
#40958=CARTESIAN_POINT('Ctrl Pts',(-0.0889581327325248,0.0440685769717619,
-0.329321814258519));
#40959=CARTESIAN_POINT('Ctrl Pts',(-0.0751598805966252,0.0610546018118317,
-0.330769517232263));
#40960=CARTESIAN_POINT('Ctrl Pts',(-0.054989170778521,0.0858852959198736,
-0.332885814013812));
#40961=CARTESIAN_POINT('Ctrl Pts',(-0.0212971846766535,0.0997322559807113,
-0.33500211079536));
#40962=CARTESIAN_POINT('Ctrl Pts',(0.0105049576247015,0.0962617157493233,
-0.337118407576909));
#40963=CARTESIAN_POINT('Ctrl Pts',(0.0423070999260574,0.0927911755179352,
-0.339234704358457));
#40964=CARTESIAN_POINT('Ctrl Pts',(0.0722193984269001,0.0720031349943205,
-0.341351001140006));
#40965=CARTESIAN_POINT('Ctrl Pts',(0.0865596076579527,0.0434062941956763,
-0.343467297921554));
#40966=CARTESIAN_POINT('Ctrl Pts',(0.100899816889005,0.0148094533970324,
-0.345583594703102));
#40967=CARTESIAN_POINT('Ctrl Pts',(0.0996679368502675,-0.0215961876766415,
-0.347699891484651));
#40968=CARTESIAN_POINT('Ctrl Pts',(0.0834274443029201,-0.049158250485381,
-0.349816188266199));
#40969=CARTESIAN_POINT('Ctrl Pts',(0.0671869517555729,-0.07672031329412,
-0.351932485047748));
#40970=CARTESIAN_POINT('Ctrl Pts',(0.0359378466996168,-0.0954387978379257,
-0.354048781829296));
#40971=CARTESIAN_POINT('Ctrl Pts',(0.0039738460173819,-0.0967516439215915,
-0.356165078610845));
#40972=CARTESIAN_POINT('Ctrl Pts',(-0.027990154664854,-0.0980644900052573,
-0.358281375392393));
#40973=CARTESIAN_POINT('Ctrl Pts',(-0.0606690509733682,-0.0819716976287823,
-0.360397672173941));
#40974=CARTESIAN_POINT('Ctrl Pts',(-0.0791151222926576,-0.0558343037774998,
-0.36251396895549));
#40975=CARTESIAN_POINT('Ctrl Pts',(-0.0904823268696878,-0.0397273996093885,
-0.363818115407337));
#40976=CARTESIAN_POINT('Ctrl Pts',(-0.0964445937205749,-0.0198060421970087,
-0.365122261859184));
#40977=CARTESIAN_POINT('Ctrl Pts',(-0.0965509256710446,5.67507499378977E-5,
-0.366426408311032));
#40978=CARTESIAN_POINT('Ctrl Pts',(-0.0965423984694297,5.0056945484775E-5,
-0.372223591688966));
#40979=CARTESIAN_POINT('Ctrl Pts',(-0.0964514972688789,-0.0193076321277276,
-0.370952890328855));
#40980=CARTESIAN_POINT('Ctrl Pts',(-0.090812222688808,-0.0387140734331841,
-0.369682188968743));
#40981=CARTESIAN_POINT('Ctrl Pts',(-0.079985242555171,-0.0545805161383707,
-0.368411487608632));
#40982=CARTESIAN_POINT('Ctrl Pts',(-0.0619533871326681,-0.0810053730604315,
-0.366295190827084));
#40983=CARTESIAN_POINT('Ctrl Pts',(-0.0295321719263656,-0.0976111851335773,
-0.364178894045535));
#40984=CARTESIAN_POINT('Ctrl Pts',(0.00244854888678868,-0.096802253986617,
-0.362062597263987));
#40985=CARTESIAN_POINT('Ctrl Pts',(0.0344292696999425,-0.0959933228396567,
-0.359946300482439));
#40986=CARTESIAN_POINT('Ctrl Pts',(0.0659694961199474,-0.0777696484725894,
-0.35783000370089));
#40987=CARTESIAN_POINT('Ctrl Pts',(0.082642348847544,-0.0504669589484183,
-0.355713706919342));
#40988=CARTESIAN_POINT('Ctrl Pts',(0.0993152015751415,-0.0231642694242456,
-0.353597410137793));
#40989=CARTESIAN_POINT('Ctrl Pts',(0.101120680610329,0.0132174352570328,
-0.351481113356245));
#40990=CARTESIAN_POINT('Ctrl Pts',(0.0872329381049923,0.042036725349521,
-0.349364816574696));
#40991=CARTESIAN_POINT('Ctrl Pts',(0.0733451955996561,0.0708560154420084,
-0.347248519793148));
#40992=CARTESIAN_POINT('Ctrl Pts',(0.0437642315537964,0.0921128909457067,
-0.345132223011599));
#40993=CARTESIAN_POINT('Ctrl Pts',(0.0120207350678154,0.0960842010788969,
-0.343015926230051));
#40994=CARTESIAN_POINT('Ctrl Pts',(-0.0197227614181652,0.100055511212087,
-0.340899629448502));
#40995=CARTESIAN_POINT('Ctrl Pts',(-0.0536287903442663,0.0867412559747704,
-0.338783332666954));
#40996=CARTESIAN_POINT('Ctrl Pts',(-0.0741883258613981,0.0622315360120855,
-0.336667035885406));
#40997=CARTESIAN_POINT('Ctrl Pts',(-0.0885774779519113,0.0450777395196946,
-0.335185887819926));
#40998=CARTESIAN_POINT('Ctrl Pts',(-0.0964291408375652,0.0224400883890291,
-0.333704739754446));
#40999=CARTESIAN_POINT('Ctrl Pts',(-0.0966122385588212,-8.24931776182297E-5,
-0.332223591688966));
#41000=CARTESIAN_POINT('Origin',(0.,0.,-0.593));
#41001=CARTESIAN_POINT('',(-0.0968321016897829,-9.30107239267841E-6,-0.286426408311032));
#41002=CARTESIAN_POINT('',(-0.096833216074716,1.13968060647145E-7,-0.292223591688966));
#41003=CARTESIAN_POINT('',(-0.096675,-1.1839272930757E-17,-0.593));
#41004=CARTESIAN_POINT('Ctrl Pts',(-0.0968321016897829,-9.30107239267841E-6,
-0.286426408311032));
#41005=CARTESIAN_POINT('Ctrl Pts',(-0.0967888706163907,0.0314831625185701,
-0.288509663928818));
#41006=CARTESIAN_POINT('Ctrl Pts',(-0.0799841734743482,0.0630152174938467,
-0.290592919546605));
#41007=CARTESIAN_POINT('Ctrl Pts',(-0.0538006019224041,0.0805119077310139,
-0.292676175164392));
#41008=CARTESIAN_POINT('Ctrl Pts',(-0.0272017497548095,0.0982861016035854,
-0.29479247194594));
#41009=CARTESIAN_POINT('Ctrl Pts',(0.00907584055141718,0.101576188530772,
-0.296908768727489));
#41010=CARTESIAN_POINT('Ctrl Pts',(0.0384383624190365,0.0888772431404299,
-0.299025065509037));
#41011=CARTESIAN_POINT('Ctrl Pts',(0.0678008842866576,0.0761782977500875,
-0.301141362290586));
#41012=CARTESIAN_POINT('Ctrl Pts',(0.0902483377156704,0.0474903200422152,
-0.303257659072134));
#41013=CARTESIAN_POINT('Ctrl Pts',(0.0955129872471203,0.0159355364149357,
-0.305373955853682));
#41014=CARTESIAN_POINT('Ctrl Pts',(0.10077763677857,-0.015619247212342,
-0.307490252635231));
#41015=CARTESIAN_POINT('Ctrl Pts',(0.0888594824124587,-0.0500408367590265,
-0.30960654941678));
#41016=CARTESIAN_POINT('Ctrl Pts',(0.0652100314468056,-0.0715843827409785,
-0.311722846198328));
#41017=CARTESIAN_POINT('Ctrl Pts',(0.0415605804811526,-0.0931279287229305,
-0.313839142979876));
#41018=CARTESIAN_POINT('Ctrl Pts',(0.00617983291595768,-0.10179343114015,
-0.315955439761424));
#41019=CARTESIAN_POINT('Ctrl Pts',(-0.0247486313390017,-0.0936171848569828,
-0.318071736542973));
#41020=CARTESIAN_POINT('Ctrl Pts',(-0.055677095593962,-0.0854409385738153,
-0.320188033324521));
#41021=CARTESIAN_POINT('Ctrl Pts',(-0.0821532765386865,-0.0604229435902602,
-0.32230433010607));
#41022=CARTESIAN_POINT('Ctrl Pts',(-0.0920666502438785,-0.0300067320208591,
-0.324420626887618));
#41023=CARTESIAN_POINT('Ctrl Pts',(-0.0951985456999085,-0.0203974508985341,
-0.325089220695423));
#41024=CARTESIAN_POINT('Ctrl Pts',(-0.0966773168755601,-0.0102493768783783,
-0.325757814503227));
#41025=CARTESIAN_POINT('Ctrl Pts',(-0.0965988706096985,-7.90725476241677E-5,
-0.326426408311032));
#41026=CARTESIAN_POINT('Ctrl Pts',(-0.0966122385588212,-8.24931776182297E-5,
-0.332223591688966));
#41027=CARTESIAN_POINT('Ctrl Pts',(-0.0966907548701079,-0.00974066922227465,
-0.331588442972898));
#41028=CARTESIAN_POINT('Ctrl Pts',(-0.0953591124199333,-0.0193776853301763,
-0.330953294256829));
#41029=CARTESIAN_POINT('Ctrl Pts',(-0.0925281198827719,-0.028552036696178,
-0.33031814554076));
#41030=CARTESIAN_POINT('Ctrl Pts',(-0.0830953362788522,-0.0591207047537023,
-0.328201848759212));
#41031=CARTESIAN_POINT('Ctrl Pts',(-0.0570167269628521,-0.0845528561806965,
-0.326085551977664));
#41032=CARTESIAN_POINT('Ctrl Pts',(-0.0262209618144473,-0.0932155187190727,
-0.323969255196115));
#41033=CARTESIAN_POINT('Ctrl Pts',(0.00457480333395574,-0.101878181257448,
-0.321852958414567));
#41034=CARTESIAN_POINT('Ctrl Pts',(0.0400877243147619,-0.0937713549072077,
-0.319736661633018));
#41035=CARTESIAN_POINT('Ctrl Pts',(0.0640737635065671,-0.0726031996446781,
-0.31762036485147));
#41036=CARTESIAN_POINT('Ctrl Pts',(0.0880598026983737,-0.0514350443821474,
-0.315504068069922));
#41037=CARTESIAN_POINT('Ctrl Pts',(0.100518960101178,-0.017205560207324,
-0.313387771288373));
#41038=CARTESIAN_POINT('Ctrl Pts',(0.0957522671144628,0.0144282747056279,
-0.311271474506825));
#41039=CARTESIAN_POINT('Ctrl Pts',(0.0909855741277478,0.0460621096185807,
-0.309155177725276));
#41040=CARTESIAN_POINT('Ctrl Pts',(0.0689930307515148,0.0751002952696631,
-0.307038880943728));
#41041=CARTESIAN_POINT('Ctrl Pts',(0.0398342911095972,0.0882604159311316,
-0.304922584162179));
#41042=CARTESIAN_POINT('Ctrl Pts',(0.0106755514676821,0.101420536592599,
-0.302806287380631));
#41043=CARTESIAN_POINT('Ctrl Pts',(-0.0256493844399152,0.0987025922644553,
-0.300689990599082));
#41044=CARTESIAN_POINT('Ctrl Pts',(-0.0525250535878632,0.0813498034056174,
-0.298573693817534));
#41045=CARTESIAN_POINT('Ctrl Pts',(-0.0794058523729649,0.0639937024986232,
-0.296456993108011));
#41046=CARTESIAN_POINT('Ctrl Pts',(-0.0968337763961882,0.0319971699547993,
-0.294340292398489));
#41047=CARTESIAN_POINT('Ctrl Pts',(-0.096833216074716,1.13968060647145E-7,
-0.292223591688966));
#41048=CARTESIAN_POINT('Origin',(0.,0.,-0.593));
#41049=CARTESIAN_POINT('',(-0.0966258978973466,8.50958607245579E-5,-0.246426408311032));
#41050=CARTESIAN_POINT('',(-0.0966119077409059,8.24194000266483E-5,-0.252223591688966));
#41051=CARTESIAN_POINT('',(-0.096675,-1.1839272930757E-17,-0.593));
#41052=CARTESIAN_POINT('Ctrl Pts',(-0.0966258978973466,8.50958607245579E-5,
-0.246426408311032));
#41053=CARTESIAN_POINT('Ctrl Pts',(-0.0967035430033851,0.0092437051732415,
-0.247028919791313));
#41054=CARTESIAN_POINT('Ctrl Pts',(-0.0955076479844384,0.0183824419548729,
-0.247631431271594));
#41055=CARTESIAN_POINT('Ctrl Pts',(-0.0929562892575429,0.0271256399218355,
-0.248233942751875));
#41056=CARTESIAN_POINT('Ctrl Pts',(-0.0839947467160028,0.0578357630041277,
-0.250350239533423));
#41057=CARTESIAN_POINT('Ctrl Pts',(-0.0583103507134378,0.0836659784968148,
-0.252466536314972));
#41058=CARTESIAN_POINT('Ctrl Pts',(-0.0276514532137634,0.0928012348455942,
-0.25458283309652));
#41059=CARTESIAN_POINT('Ctrl Pts',(0.00300744428591197,0.101936491194374,
-0.256699129878069));
#41060=CARTESIAN_POINT('Ctrl Pts',(0.0386408432826971,0.0943767883992445,
-0.258815426659617));
#41061=CARTESIAN_POINT('Ctrl Pts',(0.0629495980601638,0.0735800255352227,
-0.260931723441166));
#41062=CARTESIAN_POINT('Ctrl Pts',(0.0872583528376278,0.0527832626712033,
-0.263048020222714));
#41063=CARTESIAN_POINT('Ctrl Pts',(0.100242463395776,0.0187494397382947,
-0.265164317004262));
#41064=CARTESIAN_POINT('Ctrl Pts',(0.0959628412405606,-0.0129539628970974,
-0.267280613785811));
#41065=CARTESIAN_POINT('Ctrl Pts',(0.0916832190853444,-0.044657365532493,
-0.269396910567359));
#41066=CARTESIAN_POINT('Ctrl Pts',(0.0701398642167597,-0.0740303478703715,
-0.271513207348908));
#41067=CARTESIAN_POINT('Ctrl Pts',(0.0411869665271511,-0.0876373541475984,
-0.273629504130456));
#41068=CARTESIAN_POINT('Ctrl Pts',(0.0122340688375434,-0.101244360424825,
-0.275745800912005));
#41069=CARTESIAN_POINT('Ctrl Pts',(-0.0241283716730878,-0.0990853906414008,
-0.277862097693553));
#41070=CARTESIAN_POINT('Ctrl Pts',(-0.0512677369224376,-0.0821479835696045,
-0.279978394475101));
#41071=CARTESIAN_POINT('Ctrl Pts',(-0.0784071021717868,-0.0652105764978087,
-0.28209469125665));
#41072=CARTESIAN_POINT('Ctrl Pts',(-0.0963233921598552,-0.0334947321376415,
-0.284210988038198));
#41073=CARTESIAN_POINT('Ctrl Pts',(-0.0968214801394086,-0.00150765954857932,
-0.286327284819747));
#41074=CARTESIAN_POINT('Ctrl Pts',(-0.0968292566510225,-0.00100825411882745,
-0.286360325983508));
#41075=CARTESIAN_POINT('Ctrl Pts',(-0.0968327873497487,-0.000508782575230481,
-0.28639336714727));
#41076=CARTESIAN_POINT('Ctrl Pts',(-0.0968321016897829,-9.30107239267841E-6,
-0.286426408311032));
#41077=CARTESIAN_POINT('Ctrl Pts',(-0.096833216074716,1.13968060647145E-7,
-0.292223591688966));
#41078=CARTESIAN_POINT('Ctrl Pts',(-0.096832655967095,-0.0319847300834253,
-0.290107698835392));
#41079=CARTESIAN_POINT('Ctrl Pts',(-0.0794199518304906,-0.0639700965998081,
-0.287991805981818));
#41080=CARTESIAN_POINT('Ctrl Pts',(-0.0525560190935891,-0.0813298015832744,
-0.285875913128243));
#41081=CARTESIAN_POINT('Ctrl Pts',(-0.0256869579807819,-0.0986928205674731,
-0.283759616346695));
#41082=CARTESIAN_POINT('Ctrl Pts',(0.0106369405918268,-0.10142459335248,
-0.281643319565147));
#41083=CARTESIAN_POINT('Ctrl Pts',(0.0398006880884165,-0.088275574176717,
-0.279527022783598));
#41084=CARTESIAN_POINT('Ctrl Pts',(0.0689644355850071,-0.0751265550009541,
-0.27741072600205));
#41085=CARTESIAN_POINT('Ctrl Pts',(0.0909680320055784,-0.0460967438644211,
-0.275294429220502));
#41086=CARTESIAN_POINT('Ctrl Pts',(0.0957467674307411,-0.0144647258910801,
-0.273178132438953));
#41087=CARTESIAN_POINT('Ctrl Pts',(0.100525502855904,0.0171672920822619,
-0.271061835657405));
#41088=CARTESIAN_POINT('Ctrl Pts',(0.0880793772856569,0.0514015168924121,
-0.268945538875856));
#41089=CARTESIAN_POINT('Ctrl Pts',(0.0641013984034045,0.0725788019415346,
-0.266829242094308));
#41090=CARTESIAN_POINT('Ctrl Pts',(0.0401234195211542,0.0937560869906552,
-0.264712945312759));
#41091=CARTESIAN_POINT('Ctrl Pts',(0.00461358732690071,0.101876432278751,
-0.262596648531211));
#41092=CARTESIAN_POINT('Ctrl Pts',(-0.0261854734061089,0.093225494104555,
-0.260480351749662));
#41093=CARTESIAN_POINT('Ctrl Pts',(-0.0569845341391203,0.0845745559303588,
-0.258364054968114));
#41094=CARTESIAN_POINT('Ctrl Pts',(-0.0830728234108873,0.0591523342938697,
-0.256247758186566));
#41095=CARTESIAN_POINT('Ctrl Pts',(-0.0925172436134204,0.0285872594474463,
-0.254131461405017));
#41096=CARTESIAN_POINT('Ctrl Pts',(-0.0953553337853935,0.0194023188510939,
-0.253495504833));
#41097=CARTESIAN_POINT('Ctrl Pts',(-0.096690434039967,0.00975296361118441,
-0.252859548260983));
#41098=CARTESIAN_POINT('Ctrl Pts',(-0.0966119077409059,8.24194000266483E-5,
-0.252223591688966));
#41099=CARTESIAN_POINT('Origin',(0.,0.,-0.593));
#41100=CARTESIAN_POINT('',(-0.0965351754675536,-4.30991072692052E-5,-0.206426408311032));
#41101=CARTESIAN_POINT('',(-0.0965425912303032,-5.0224085100017E-5,-0.212223591688966));
#41102=CARTESIAN_POINT('',(-0.096675,-1.1839272930757E-17,-0.593));
#41103=CARTESIAN_POINT('Ctrl Pts',(-0.0965351754675536,-4.30991072692052E-5,
-0.206426408311032));
#41104=CARTESIAN_POINT('Ctrl Pts',(-0.0964592547998338,0.018820931113738,
-0.207664472435356));
#41105=CARTESIAN_POINT('Ctrl Pts',(-0.0911250957801962,0.0377246133573255,
-0.20890253655968));
#41106=CARTESIAN_POINT('Ctrl Pts',(-0.0808151957183313,0.0533439424371889,
-0.210140600684003));
#41107=CARTESIAN_POINT('Ctrl Pts',(-0.0631918691956234,0.0800429923589462,
-0.212256897465552));
#41108=CARTESIAN_POINT('Ctrl Pts',(-0.03102987416261,0.0971454572669495,
-0.2143731942471));
#41109=CARTESIAN_POINT('Ctrl Pts',(0.000959505631360331,0.0968284638039782,
-0.216489491028648));
#41110=CARTESIAN_POINT('Ctrl Pts',(0.0329488854253307,0.0965114703410068,
-0.218605787810197));
#41111=CARTESIAN_POINT('Ctrl Pts',(0.0647656499802579,0.078775018507061,
-0.220722084591745));
#41112=CARTESIAN_POINT('Ctrl Pts',(0.0818564281248476,0.0517319749123845,
-0.222838381373294));
#41113=CARTESIAN_POINT('Ctrl Pts',(0.0989472062694382,0.0246889313177066,
-0.224954678154842));
#41114=CARTESIAN_POINT('Ctrl Pts',(0.101311998003689,-0.0116607040377033,
-0.227070974936391));
#41115=CARTESIAN_POINT('Ctrl Pts',(0.0878691191168146,-0.0406901703036554,
-0.229187271717939));
#41116=CARTESIAN_POINT('Ctrl Pts',(0.0744262402299409,-0.0697196365696058,
-0.231303568499488));
#41117=CARTESIAN_POINT('Ctrl Pts',(0.0451756907219436,-0.0914289337460994,
-0.233419865281036));
#41118=CARTESIAN_POINT('Ctrl Pts',(0.0134970241056018,-0.0958879679312891,
-0.235536162062584));
#41119=CARTESIAN_POINT('Ctrl Pts',(-0.0181816425107408,-0.100347002116479,
-0.237652458844133));
#41120=CARTESIAN_POINT('Ctrl Pts',(-0.0522884262354281,-0.0875557733103637,
-0.239768755625681));
#41121=CARTESIAN_POINT('Ctrl Pts',(-0.0732224735575136,-0.0633651435713575,
-0.24188505240723));
#41122=CARTESIAN_POINT('Ctrl Pts',(-0.0881965799345135,-0.0460616065407357,
-0.243398837708497));
#41123=CARTESIAN_POINT('Ctrl Pts',(-0.0964308177634683,-0.0229255331664144,
-0.244912623009765));
#41124=CARTESIAN_POINT('Ctrl Pts',(-0.0966258978973466,8.50958607245579E-5,
-0.246426408311032));
#41125=CARTESIAN_POINT('Ctrl Pts',(-0.0966119077409059,8.24194000266483E-5,
-0.252223591688966));
#41126=CARTESIAN_POINT('Ctrl Pts',(-0.0964291190991639,-0.0224280727840927,
-0.250743251479435));
#41127=CARTESIAN_POINT('Ctrl Pts',(-0.0885867876710175,-0.0450533745206066,
-0.249262911269903));
#41128=CARTESIAN_POINT('Ctrl Pts',(-0.0742120116041304,-0.0622032885160329,
-0.247782571060372));
#41129=CARTESIAN_POINT('Ctrl Pts',(-0.0536618082590074,-0.0867208335767331,
-0.245666274278824));
#41130=CARTESIAN_POINT('Ctrl Pts',(-0.019760850435462,-0.100047995641777,
-0.243549977497275));
#41131=CARTESIAN_POINT('Ctrl Pts',(0.011984155600785,-0.0960887703276321,
-0.241433680715727));
#41132=CARTESIAN_POINT('Ctrl Pts',(0.043729161637033,-0.0921295450134873,
-0.239317383934178));
#41133=CARTESIAN_POINT('Ctrl Pts',(0.0733182158859835,-0.0708839323201507,
-0.23720108715263));
#41134=CARTESIAN_POINT('Ctrl Pts',(0.0872169286909223,-0.0420699312842774,
-0.235084790371081));
#41135=CARTESIAN_POINT('Ctrl Pts',(0.101115641495861,-0.0132559302484049,
-0.232968493589533));
#41136=CARTESIAN_POINT('Ctrl Pts',(0.0993240128567908,0.0231264591300049,
-0.230852196807985));
#41137=CARTESIAN_POINT('Ctrl Pts',(0.0826615552839103,0.050435493916336,
-0.228735900026436));
#41138=CARTESIAN_POINT('Ctrl Pts',(0.0659990977110294,0.0777445287026677,
-0.226619603244888));
#41139=CARTESIAN_POINT('Ctrl Pts',(0.0344658112043376,0.0959802088969194,
-0.224503306463339));
#41140=CARTESIAN_POINT('Ctrl Pts',(0.00248540066314722,0.0968013148262096,
-0.222387009681791));
#41141=CARTESIAN_POINT('Ctrl Pts',(-0.0294950098780432,0.0976224207554999,
-0.220270712900242));
#41142=CARTESIAN_POINT('Ctrl Pts',(-0.0619225444537312,0.0810289524198287,
-0.218154416118694));
#41143=CARTESIAN_POINT('Ctrl Pts',(-0.079964458331246,0.0546109620162111,
-0.216038119337145));
#41144=CARTESIAN_POINT('Ctrl Pts',(-0.0908043650828087,0.0387385576536239,
-0.214766610121085));
#41145=CARTESIAN_POINT('Ctrl Pts',(-0.096451317698328,0.0193196749306095,
-0.213495100905026));
#41146=CARTESIAN_POINT('Ctrl Pts',(-0.0965425912303032,-5.0224085100017E-5,
-0.212223591688966));
#41147=CARTESIAN_POINT('Origin',(0.,0.,-0.593));
#41148=CARTESIAN_POINT('',(-0.0967832346277187,-6.11107174333103E-5,-0.166426408311032));
#41149=CARTESIAN_POINT('',(-0.0967948658423725,-5.42027044862851E-5,-0.172223591688967));
#41150=CARTESIAN_POINT('',(-0.096675,-1.1839272930757E-17,-0.593));
#41151=CARTESIAN_POINT('Ctrl Pts',(-0.0967832346277187,-6.11107174333103E-5,
-0.166426408311032));
#41152=CARTESIAN_POINT('Ctrl Pts',(-0.0965738675467705,0.0283001656582659,
-0.168300025079399));
#41153=CARTESIAN_POINT('Ctrl Pts',(-0.0833609810550404,0.0568311707808718,
-0.170173641847765));
#41154=CARTESIAN_POINT('Ctrl Pts',(-0.0614791216390247,0.0748130313352698,
-0.172047258616132));
#41155=CARTESIAN_POINT('Ctrl Pts',(-0.0367630167032322,0.0951239904705796,
-0.17416355539768));
#41156=CARTESIAN_POINT('Ctrl Pts',(-0.000986806504219694,0.101976071561127,
-0.176279852179229));
#41157=CARTESIAN_POINT('Ctrl Pts',(0.0294850396506297,0.09223505022771,
-0.178396148960777));
#41158=CARTESIAN_POINT('Ctrl Pts',(0.0599568858054783,0.0824940288942931,
-0.180512445742326));
#41159=CARTESIAN_POINT('Ctrl Pts',(0.085124367916164,0.0561599051369124,
-0.182628742523874));
#41160=CARTESIAN_POINT('Ctrl Pts',(0.0934755766709938,0.0252782242125185,
-0.184745039305422));
#41161=CARTESIAN_POINT('Ctrl Pts',(0.101826785425824,-0.00560345671187625,
-0.186861336086971));
#41162=CARTESIAN_POINT('Ctrl Pts',(0.0933617208247971,-0.0410326948032845,
-0.188977632868519));
#41163=CARTESIAN_POINT('Ctrl Pts',(0.0719524053255447,-0.0648037299990389,
-0.191093929650068));
#41164=CARTESIAN_POINT('Ctrl Pts',(0.0505430898262929,-0.0885747651947925,
-0.193210226431616));
#41165=CARTESIAN_POINT('Ctrl Pts',(0.0161895234288162,-0.100687597494893,
-0.195326523213164));
#41166=CARTESIAN_POINT('Ctrl Pts',(-0.015394558986119,-0.0956016715717106,
-0.197442819994713));
#41167=CARTESIAN_POINT('Ctrl Pts',(-0.0469786414010552,-0.0905157456485279,
-0.199559116776261));
#41168=CARTESIAN_POINT('Ctrl Pts',(-0.0757932398334497,-0.0682310615020615,
-0.20167541355781));
#41169=CARTESIAN_POINT('Ctrl Pts',(-0.0886582100434459,-0.0389409019610718,
-0.203791710339358));
#41170=CARTESIAN_POINT('Ctrl Pts',(-0.0939969872277939,-0.026785907978898,
-0.204669942996583));
#41171=CARTESIAN_POINT('Ctrl Pts',(-0.0965890305211326,-0.0134244798140298,
-0.205548175653807));
#41172=CARTESIAN_POINT('Ctrl Pts',(-0.0965351754675536,-4.30991072692052E-5,
-0.206426408311032));
#41173=CARTESIAN_POINT('Ctrl Pts',(-0.0965425912303032,-5.0224085100017E-5,
-0.212223591688966));
#41174=CARTESIAN_POINT('Ctrl Pts',(-0.0966032331382791,-0.0129195368879978,
-0.211378804123477));
#41175=CARTESIAN_POINT('Ctrl Pts',(-0.0942114646287571,-0.0257672271039402,
-0.210534016557989));
#41176=CARTESIAN_POINT('Ctrl Pts',(-0.0892609053485345,-0.0375388138450597,
-0.2096892289925));
#41177=CARTESIAN_POINT('Ctrl Pts',(-0.0768591453089668,-0.0670280868311531,
-0.207572932210952));
#41178=CARTESIAN_POINT('Ctrl Pts',(-0.0483993320504909,-0.0897641203317749,
-0.205456635429404));
#41179=CARTESIAN_POINT('Ctrl Pts',(-0.0168993268047482,-0.0953471788889501,
-0.203340338647855));
#41180=CARTESIAN_POINT('Ctrl Pts',(0.0146006784409936,-0.100930237446125,
-0.201224041866307));
#41181=CARTESIAN_POINT('Ctrl Pts',(0.049140875674001,-0.0893603210598525,
-0.199107745084758));
#41182=CARTESIAN_POINT('Ctrl Pts',(0.0709221628258518,-0.0659296487832139,
-0.19699144830321));
#41183=CARTESIAN_POINT('Ctrl Pts',(0.0927034499777021,-0.0424989765065759,
-0.194875151521661));
#41184=CARTESIAN_POINT('Ctrl Pts',(0.101725827048397,-0.00720754833957142,
-0.192758854740113));
#41185=CARTESIAN_POINT('Ctrl Pts',(0.093862350140176,0.0238019115755997,
-0.190642557958565));
#41186=CARTESIAN_POINT('Ctrl Pts',(0.0859988732319544,0.0548113714907725,
-0.188526261177016));
#41187=CARTESIAN_POINT('Ctrl Pts',(0.0612495423448144,0.0815388631541128,
-0.186409964395468));
#41188=CARTESIAN_POINT('Ctrl Pts',(0.0309349993989626,0.0917589100889316,
-0.184293667613919));
#41189=CARTESIAN_POINT('Ctrl Pts',(0.000620456453112605,0.10197895702375,
-0.182177370832371));
#41190=CARTESIAN_POINT('Ctrl Pts',(-0.0352592985514467,0.0956915592300501,
-0.180061074050823));
#41191=CARTESIAN_POINT('Ctrl Pts',(-0.0602924336904824,0.075772648155117,
-0.177944777269274));
#41192=CARTESIAN_POINT('Ctrl Pts',(-0.0828505822822485,0.0578230883689023,
-0.176037715409172));
#41193=CARTESIAN_POINT('Ctrl Pts',(-0.0966008620437373,0.0288042201319593,
-0.174130653549069));
#41194=CARTESIAN_POINT('Ctrl Pts',(-0.0967948658423725,-5.42027044862851E-5,
-0.172223591688967));
#41195=CARTESIAN_POINT('Origin',(0.,0.,-0.593));
#41196=CARTESIAN_POINT('',(-0.0967207250391251,8.29397659327311E-5,-0.126426408311032));
#41197=CARTESIAN_POINT('',(-0.0967054797063448,8.55434351395205E-5,-0.132223591688966));
#41198=CARTESIAN_POINT('',(-0.096675,-1.1839272930757E-17,-0.593));
#41199=CARTESIAN_POINT('Ctrl Pts',(-0.0967207250391251,8.29397659327311E-5,
-0.126426408311032));
#41200=CARTESIAN_POINT('Ctrl Pts',(-0.0967748071718798,0.0060399254137226,
-0.126819280941893));
#41201=CARTESIAN_POINT('Ctrl Pts',(-0.0962716703858991,0.0119878001314283,
-0.127212153572754));
#41202=CARTESIAN_POINT('Ctrl Pts',(-0.0951784404822581,0.0178251613315098,
-0.127605026203615));
#41203=CARTESIAN_POINT('Ctrl Pts',(-0.0892895117434499,0.0492694202339371,
-0.129721322985163));
#41204=CARTESIAN_POINT('Ctrl Pts',(-0.0662779660166628,0.0775069299341794,
-0.131837619766712));
#41205=CARTESIAN_POINT('Ctrl Pts',(-0.0366695589289991,0.0896215127660818,
-0.13395391654826));
#41206=CARTESIAN_POINT('Ctrl Pts',(-0.00706115184133365,0.101736095597985,
-0.136070213329808));
#41207=CARTESIAN_POINT('Ctrl Pts',(0.0291441166072093,0.0977277515615458,
-0.138186510111357));
#41208=CARTESIAN_POINT('Ctrl Pts',(0.055385519441118,0.0794299458780596,
-0.140302806892906));
#41209=CARTESIAN_POINT('Ctrl Pts',(0.0816269222750259,0.0611321401945739,
-0.142419103674454));
#41210=CARTESIAN_POINT('Ctrl Pts',(0.0979044594943001,0.028544872864042,
-0.144535400456002));
#41211=CARTESIAN_POINT('Ctrl Pts',(0.0967725902766724,-0.00342604790653714,
-0.146651697237551));
#41212=CARTESIAN_POINT('Ctrl Pts',(0.0956407210590447,-0.0353969686771154,
-0.148767994019099));
#41213=CARTESIAN_POINT('Ctrl Pts',(0.0770994454045165,-0.0667515428877409,
-0.150884290800648));
#41214=CARTESIAN_POINT('Ctrl Pts',(0.0496297656710845,-0.0831478106837788,
-0.153000587582196));
#41215=CARTESIAN_POINT('Ctrl Pts',(0.0221600859376509,-0.0995440784798177,
-0.155116884363744));
#41216=CARTESIAN_POINT('Ctrl Pts',(-0.0142379978746874,-0.100982039861267,
-0.157233181145293));
#41217=CARTESIAN_POINT('Ctrl Pts',(-0.0429155638196797,-0.0868039540382351,
-0.159349477926842));
#41218=CARTESIAN_POINT('Ctrl Pts',(-0.0715931297646696,-0.0726258682152039,
-0.16146577470839));
#41219=CARTESIAN_POINT('Ctrl Pts',(-0.0925501778423148,-0.0428317351876939,
-0.163582071489938));
#41220=CARTESIAN_POINT('Ctrl Pts',(-0.0962007020448521,-0.0110497500839039,
-0.165698368271487));
#41221=CARTESIAN_POINT('Ctrl Pts',(-0.0966193150056223,-0.00740524585785208,
-0.165941048284668));
#41222=CARTESIAN_POINT('Ctrl Pts',(-0.0968103528766703,-0.00373460203161953,
-0.16618372829785));
#41223=CARTESIAN_POINT('Ctrl Pts',(-0.0967832346277187,-6.11107174333103E-5,
-0.166426408311032));
#41224=CARTESIAN_POINT('Ctrl Pts',(-0.0967948658423725,-5.42027044862851E-5,
-0.172223591688967));
#41225=CARTESIAN_POINT('Ctrl Pts',(-0.0968161511349039,-0.00322042922370149,
-0.172014356767521));
#41226=CARTESIAN_POINT('Ctrl Pts',(-0.096674251824014,-0.00638472437038313,
-0.171805121846075));
#41227=CARTESIAN_POINT('Ctrl Pts',(-0.0963628966307718,-0.00953225687232562,
-0.171595886924629));
#41228=CARTESIAN_POINT('Ctrl Pts',(-0.093213709158514,-0.0413678264686656,
-0.16947959014308));
#41229=CARTESIAN_POINT('Ctrl Pts',(-0.0727288189404871,-0.0714885413051794,
-0.167363293361532));
#41230=CARTESIAN_POINT('Ctrl Pts',(-0.0442782613806259,-0.0861168237782632,
-0.165246996579984));
#41231=CARTESIAN_POINT('Ctrl Pts',(-0.0158277038207638,-0.100745106251347,
-0.163130699798435));
#41232=CARTESIAN_POINT('Ctrl Pts',(0.0205885210809334,-0.099880956361003,
-0.161014403016887));
#41233=CARTESIAN_POINT('Ctrl Pts',(0.0483131935882508,-0.0839196466581255,
-0.158898106235338));
#41234=CARTESIAN_POINT('Ctrl Pts',(0.0760378660955673,-0.0679583369552484,
-0.15678180945379));
#41235=CARTESIAN_POINT('Ctrl Pts',(0.0950709862085039,-0.0368998674398402,
-0.154665512672241));
#41236=CARTESIAN_POINT('Ctrl Pts',(0.0967065756835142,-0.00495075602753841,
-0.152549215890693));
#41237=CARTESIAN_POINT('Ctrl Pts',(0.0983421651585245,0.0269983553847643,
-0.150432919109144));
#41238=CARTESIAN_POINT('Ctrl Pts',(0.0825802239956075,0.0598381086939593,
-0.148316622327596));
#41239=CARTESIAN_POINT('Ctrl Pts',(0.0566304537585547,0.078547205402699,
-0.146200325546048));
#41240=CARTESIAN_POINT('Ctrl Pts',(0.0306806835215034,0.0972563021114377,
-0.144084028764499));
#41241=CARTESIAN_POINT('Ctrl Pts',(-0.00545691578968455,0.101834742219722,
-0.141967731982951));
#41242=CARTESIAN_POINT('Ctrl Pts',(-0.0352525709877608,0.0901882920099803,
-0.139851435201403));
#41243=CARTESIAN_POINT('Ctrl Pts',(-0.0650482261858388,0.0785418418002379,
-0.137735138419854));
#41244=CARTESIAN_POINT('Ctrl Pts',(-0.0885019372708057,0.0506705012724692,
-0.135618841638306));
#41245=CARTESIAN_POINT('Ctrl Pts',(-0.0948856947517297,0.0193229573153638,
-0.133502544856757));
#41246=CARTESIAN_POINT('Ctrl Pts',(-0.0961716717350178,0.0130081466208925,
-0.13307622713416));
#41247=CARTESIAN_POINT('Ctrl Pts',(-0.0967649474668955,0.00655227107519142,
-0.132649909411563));
#41248=CARTESIAN_POINT('Ctrl Pts',(-0.0967054797063448,8.55434351395205E-5,
-0.132223591688966));
#41249=CARTESIAN_POINT('Origin',(0.,0.,-0.593));
#41250=CARTESIAN_POINT('',(-0.0965170586776495,7.4335118630045E-6,-0.0864264083110323));
#41251=CARTESIAN_POINT('',(-0.096516496468341,-9.27006410983469E-7,-0.0922235916889666));
#41252=CARTESIAN_POINT('',(-0.096675,-1.1839272930757E-17,-0.593));
#41253=CARTESIAN_POINT('Ctrl Pts',(-0.0965170586776495,7.4335118630045E-6,
-0.0864264083110323));
#41254=CARTESIAN_POINT('Ctrl Pts',(-0.0965277726618348,0.0156846135208846,
-0.087454833585936));
#41255=CARTESIAN_POINT('Ctrl Pts',(-0.0929251385372256,0.0313571364771244,
-0.0884832588608397));
#41256=CARTESIAN_POINT('Ctrl Pts',(-0.0856824059907095,0.0451130878663906,
-0.0895116841357433));
#41257=CARTESIAN_POINT('Ctrl Pts',(-0.0707782880622152,0.0734201281177776,
-0.0916279809172917));
#41258=CARTESIAN_POINT('Ctrl Pts',(-0.0404599773489722,0.093611342862549,
-0.0937442776988399));
#41259=CARTESIAN_POINT('Ctrl Pts',(-0.00859532061802182,0.0964509920919599,
-0.0958605744803884));
#41260=CARTESIAN_POINT('Ctrl Pts',(0.0232693361129286,0.0992906413213708,
-0.0979768712619368));
#41261=CARTESIAN_POINT('Ctrl Pts',(0.056680338861587,0.0847787250354175,
-0.100093168043486));
#41262=CARTESIAN_POINT('Ctrl Pts',(0.0763550328277099,0.0595531870686323,
-0.102209464825034));
#41263=CARTESIAN_POINT('Ctrl Pts',(0.0960297267938328,0.034327649101847,
-0.104325761606582));
#41264=CARTESIAN_POINT('Ctrl Pts',(0.101968111977424,-0.00161151054576864,
-0.106442058388131));
#41265=CARTESIAN_POINT('Ctrl Pts',(0.0914539310741352,-0.031825297365229,
-0.108558355169679));
#41266=CARTESIAN_POINT('Ctrl Pts',(0.0809397501708469,-0.0620390841846885,
-0.110674651951227));
#41267=CARTESIAN_POINT('Ctrl Pts',(0.0539730031806786,-0.0865274981759914,
-0.112790948732776));
#41268=CARTESIAN_POINT('Ctrl Pts',(0.0228885882000559,-0.0940892387737843,
-0.114907245514324));
#41269=CARTESIAN_POINT('Ctrl Pts',(-0.0081958267805677,-0.101650979371577,
-0.117023542295873));
#41270=CARTESIAN_POINT('Ctrl Pts',(-0.0433979097516469,-0.0922860465758598,
-0.119139839077421));
#41271=CARTESIAN_POINT('Ctrl Pts',(-0.0666157953617716,-0.0702780761256944,
-0.12125613585897));
#41272=CARTESIAN_POINT('Ctrl Pts',(-0.0855234765231589,-0.0523556995894131,
-0.122979560009657));
#41273=CARTESIAN_POINT('Ctrl Pts',(-0.0964834816009508,-0.0260487174793249,
-0.124702984160345));
#41274=CARTESIAN_POINT('Ctrl Pts',(-0.0967207250391251,8.29397659327311E-5,
-0.126426408311032));
#41275=CARTESIAN_POINT('Ctrl Pts',(-0.0967054797063448,8.55434351395205E-5,
-0.132223591688966));
#41276=CARTESIAN_POINT('Ctrl Pts',(-0.0964697417468685,-0.0255494084150007,
-0.130533612630015));
#41277=CARTESIAN_POINT('Ctrl Pts',(-0.0859765770751443,-0.0513548936580699,
-0.128843633571063));
#41278=CARTESIAN_POINT('Ctrl Pts',(-0.0677151005125275,-0.0692194838422052,
-0.127153654512112));
#41279=CARTESIAN_POINT('Ctrl Pts',(-0.0448469449155209,-0.0915906336562278,
-0.125037357730563));
#41280=CARTESIAN_POINT('Ctrl Pts',(-0.00979682984462658,-0.101509185897832,
-0.122921060949015));
#41281=CARTESIAN_POINT('Ctrl Pts',(0.021402898869499,-0.0944382747481939,
-0.120804764167466));
#41282=CARTESIAN_POINT('Ctrl Pts',(0.0526026275836238,-0.087367363598556,
-0.118688467385918));
#41283=CARTESIAN_POINT('Ctrl Pts',(0.0799519699409812,-0.0633069890576768,
-0.11657217060437));
#41284=CARTESIAN_POINT('Ctrl Pts',(0.0909410097538229,-0.0332626572716202,
-0.114455873822821));
#41285=CARTESIAN_POINT('Ctrl Pts',(0.101930049566665,-0.00321832548556278,
-0.112339577041273));
#41286=CARTESIAN_POINT('Ctrl Pts',(0.0965587868349915,0.0328099635456709,
-0.110223280259724));
#41287=CARTESIAN_POINT('Ctrl Pts',(0.0772840974685356,0.0583424388332644,
-0.108106983478176));
#41288=CARTESIAN_POINT('Ctrl Pts',(0.0580094081020797,0.0838749141208579,
-0.105990686696628));
#41289=CARTESIAN_POINT('Ctrl Pts',(0.0248312921008405,0.0989115756648094,
-0.103874389915079));
#41290=CARTESIAN_POINT('Ctrl Pts',(-0.00707417260600754,0.0965744692966754,
-0.101758093133531));
#41291=CARTESIAN_POINT('Ctrl Pts',(-0.0389796373128547,0.0942373629285415,
-0.0996417963519824));
#41292=CARTESIAN_POINT('Ctrl Pts',(-0.0696124507253119,0.0745264886483231,
-0.0975254995704338));
#41293=CARTESIAN_POINT('Ctrl Pts',(-0.084960810759801,0.0464578455188266,
-0.0954092027888854));
#41294=CARTESIAN_POINT('Ctrl Pts',(-0.0926619842621373,0.0323741590383376,
-0.0943473324222458));
#41295=CARTESIAN_POINT('Ctrl Pts',(-0.0965151160525341,0.0161863055094454,
-0.0932854620556062));
#41296=CARTESIAN_POINT('Ctrl Pts',(-0.0965165097454088,-9.26928760177416E-7,
-0.0922235916889666));
#41297=CARTESIAN_POINT('Origin',(0.,0.,-0.593));
#41298=CARTESIAN_POINT('',(-0.0966970977580488,-8.58596968723868E-5,-0.0464264083110326));
#41299=CARTESIAN_POINT('',(-0.0967093838725941,-8.47898118814712E-5,-0.0522235916889671));
#41300=CARTESIAN_POINT('',(-0.096675,-1.1839272930757E-17,-0.593));
#41301=CARTESIAN_POINT('Ctrl Pts',(-0.0966970977580488,-8.58596968723868E-5,
-0.0464264083110326));
#41302=CARTESIAN_POINT('Ctrl Pts',(-0.096463819312519,0.0251626158010124,
-0.048090386229979));
#41303=CARTESIAN_POINT('Ctrl Pts',(-0.0863212822535982,0.0505757410207625,
-0.0497543641489254));
#41304=CARTESIAN_POINT('Ctrl Pts',(-0.0685565717469939,0.0683841308472504,
-0.0514183420678718));
#41305=CARTESIAN_POINT('Ctrl Pts',(-0.0459628827068936,0.0910333725500618,
-0.0535346388494203));
#41306=CARTESIAN_POINT('Ctrl Pts',(-0.0110399381729231,0.101381565704142,
-0.0556509356309688));
#41307=CARTESIAN_POINT('Ctrl Pts',(0.0202433730968924,0.0946936795329476,
-0.0577672324125173));
#41308=CARTESIAN_POINT('Ctrl Pts',(0.0515266843667053,0.0880057933617542,
-0.0598835291940656));
#41309=CARTESIAN_POINT('Ctrl Pts',(0.0791703623723638,0.06428182786529,
-0.061999825975614));
#41310=CARTESIAN_POINT('Ctrl Pts',(0.0905270688129109,0.0343742764785263,
-0.0641161227571623));
#41311=CARTESIAN_POINT('Ctrl Pts',(0.101883775253459,0.00446672509176077,
-0.0662324195387107));
#41312=CARTESIAN_POINT('Ctrl Pts',(0.0969535101288935,-0.031624412185305,
-0.0683487163202591));
#41313=CARTESIAN_POINT('Ctrl Pts',(0.0779929056047911,-0.0573910712254237,
-0.0704650131018076));
#41314=CARTESIAN_POINT('Ctrl Pts',(0.0590323010806893,-0.0831577302655415,
-0.072581309883356));
#41315=CARTESIAN_POINT('Ctrl Pts',(0.0260413571570511,-0.0985999110687128,
-0.0746976066649044));
#41316=CARTESIAN_POINT('Ctrl Pts',(-0.00589024604478475,-0.0966539334751514,
-0.0768139034464528));
#41317=CARTESIAN_POINT('Ctrl Pts',(-0.0378218492466215,-0.09470795588159,
-0.0789302002280012));
#41318=CARTESIAN_POINT('Ctrl Pts',(-0.068694111726656,-0.0753738198912948,
-0.0810464970095495));
#41319=CARTESIAN_POINT('Ctrl Pts',(-0.0843852803948016,-0.0474953190171464,
-0.0831627937910979));
#41320=CARTESIAN_POINT('Ctrl Pts',(-0.0924512451729286,-0.0331645186240334,
-0.0842506652977427));
#41321=CARTESIAN_POINT('Ctrl Pts',(-0.0965057253913115,-0.0165759370572375,
-0.0853385368043875));
#41322=CARTESIAN_POINT('Ctrl Pts',(-0.0965170586776495,7.4335118630045E-6,
-0.0864264083110323));
#41323=CARTESIAN_POINT('Ctrl Pts',(-0.0965165097454088,-9.26928760177416E-7,
-0.0922235916889666));
#41324=CARTESIAN_POINT('Ctrl Pts',(-0.096517893668181,-0.0160746832019732,
-0.0911691652740578));
#41325=CARTESIAN_POINT('Ctrl Pts',(-0.0927213533189873,-0.0321478270619503,
-0.090114738859149));
#41326=CARTESIAN_POINT('Ctrl Pts',(-0.0851232695060613,-0.0461595259106198,
-0.0890603124442402));
#41327=CARTESIAN_POINT('Ctrl Pts',(-0.0698734615613114,-0.0742818422317921,
-0.0869440156626918));
#41328=CARTESIAN_POINT('Ctrl Pts',(-0.0393099390152905,-0.0941000628953607,
-0.0848277188811432));
#41329=CARTESIAN_POINT('Ctrl Pts',(-0.00741288109560678,-0.0965490669160594,
-0.0827114220995947));
#41330=CARTESIAN_POINT('Ctrl Pts',(0.0244841768240779,-0.0989980709367582,
-0.0805951253180463));
#41331=CARTESIAN_POINT('Ctrl Pts',(0.0577147701174238,-0.0840778583145879,
-0.0784788285364981));
#41332=CARTESIAN_POINT('Ctrl Pts',(0.0770789316037844,-0.0586131675103347,
-0.0763625317549496));
#41333=CARTESIAN_POINT('Ctrl Pts',(0.0964430930901439,-0.033148476706083,
-0.0742462349734013));
#41334=CARTESIAN_POINT('Ctrl Pts',(0.101940822769517,0.00286069228024984,
-0.0721299381918529));
#41335=CARTESIAN_POINT('Ctrl Pts',(0.0910571913412267,0.0329434136143151,
-0.0700136414103045));
#41336=CARTESIAN_POINT('Ctrl Pts',(0.0801735599129361,0.0630261349483812,
-0.0678973446287561));
#41337=CARTESIAN_POINT('Ctrl Pts',(0.0529085673769804,0.0871824086301804,
-0.0657810478472076));
#41338=CARTESIAN_POINT('Ctrl Pts',(0.0217339318258845,0.0943626715618018,
-0.0636647510656592));
#41339=CARTESIAN_POINT('Ctrl Pts',(-0.00944070372521155,0.101542934493423,
-0.0615484542841107));
#41340=CARTESIAN_POINT('Ctrl Pts',(-0.0445249822914489,0.0917471866748669,
-0.0594321575025622));
#41341=CARTESIAN_POINT('Ctrl Pts',(-0.0674716573729478,0.0694564865140366,
-0.0573158607210138));
#41342=CARTESIAN_POINT('Ctrl Pts',(-0.085876549655346,0.0515777335399252,
-0.0556184377103316));
#41343=CARTESIAN_POINT('Ctrl Pts',(-0.0964730793250058,0.0256607282996191,
-0.0539210146996493));
#41344=CARTESIAN_POINT('Ctrl Pts',(-0.0967093838725941,-8.47898118814713E-5,
-0.0522235916889671));
#41345=CARTESIAN_POINT('Origin',(0.,0.,-1.25327725593024));
#41346=CARTESIAN_POINT('',(-0.0739168918988343,-6.56325999296408E-5,-0.0332772559302393));
#41347=CARTESIAN_POINT('',(-0.0739977701941128,4.64298677421305E-5,-0.0253727440697618));
#41348=CARTESIAN_POINT('',(-0.0739,1.16448635408261E-14,-1.25327725593024));
#41349=CARTESIAN_POINT('',(0.0740196805984139,-0.000529251440437712,-0.0133250000000002));
#41350=CARTESIAN_POINT('Ctrl Pts',(-0.0739168918988343,-6.56325999296619E-5,
-0.0332772559302393));
#41351=CARTESIAN_POINT('Ctrl Pts',(-0.0739653651344989,-0.00531204660183527,
-0.0328249370676371));
#41352=CARTESIAN_POINT('Ctrl Pts',(-0.0710621488839631,-0.0350524220873821,
-0.0302563214234866));
#41353=CARTESIAN_POINT('Ctrl Pts',(-0.0307802095667008,-0.0817325634071313,
-0.0255714089977876));
#41354=CARTESIAN_POINT('Ctrl Pts',(0.0499505858280116,-0.0704769373222424,
-0.0193729758836433));
#41355=CARTESIAN_POINT('Ctrl Pts',(0.0737375927583184,-0.0232593978427314,
-0.0152908395510475));
#41356=CARTESIAN_POINT('Ctrl Pts',(0.0740200992814442,-0.000529165593930002,
-0.0133250000000002));
#41357=CARTESIAN_POINT('',(0.0233628051714112,-0.0701098376443897,-0.013325));
#41358=CARTESIAN_POINT('Origin',(0.,0.,-0.013325));
#41359=CARTESIAN_POINT('Ctrl Pts',(-0.0739977701941128,4.64298677421305E-5,
-0.0253727440697618));
#41360=CARTESIAN_POINT('Ctrl Pts',(-0.0738275065859486,-0.0219387793141415,
-0.0234731261613896));
#41361=CARTESIAN_POINT('Ctrl Pts',(-0.0517129071029879,-0.0687047144129353,
-0.019457211471469));
#41362=CARTESIAN_POINT('Ctrl Pts',(5.63936834513772E-5,-0.0778762677080245,
-0.0154412967815484));
#41363=CARTESIAN_POINT('Ctrl Pts',(0.0233628051714112,-0.0701098376443897,
-0.013325));
#41364=CARTESIAN_POINT('Origin',(0.,0.,-1.25327725593024));
#41365=CARTESIAN_POINT('',(-0.0737792669902074,5.68230181076675E-6,-0.0732772559302393));
#41366=CARTESIAN_POINT('',(-0.073926283611944,-6.48147617952552E-5,-0.0653727440697618));
#41367=CARTESIAN_POINT('',(-0.0739,1.16448635408261E-14,-1.25327725593024));
#41368=CARTESIAN_POINT('Ctrl Pts',(-0.0737792669902074,5.68230181076119E-6,
-0.0732772559302393));
#41369=CARTESIAN_POINT('Ctrl Pts',(-0.0737706036350459,-0.012670925767046,
-0.0721893844235943));
#41370=CARTESIAN_POINT('Ctrl Pts',(-0.0646420250325405,-0.0500197750844117,
-0.0689852161354008));
#41371=CARTESIAN_POINT('Ctrl Pts',(-0.00531238129869321,-0.0871756978467261,
-0.0636647510656592));
#41372=CARTESIAN_POINT('Ctrl Pts',(0.0703441200498545,-0.0517629077348786,
-0.057315860721014));
#41373=CARTESIAN_POINT('Ctrl Pts',(0.0816504534154235,0.0310031138252487,
-0.0509669703763687));
#41374=CARTESIAN_POINT('Ctrl Pts',(0.018256572744571,0.0854081115037233,
-0.0446180800317234));
#41375=CARTESIAN_POINT('Ctrl Pts',(-0.0561247861037155,0.0633677973579271,
-0.0387215085496804));
#41376=CARTESIAN_POINT('Ctrl Pts',(-0.0737385699218513,0.0192347277754885,
-0.0349412338491856));
#41377=CARTESIAN_POINT('Ctrl Pts',(-0.0739168918988343,-6.56325999296619E-5,
-0.0332772559302393));
#41378=CARTESIAN_POINT('Ctrl Pts',(-0.073926283611944,-6.48147617952535E-5,
-0.0653727440697618));
#41379=CARTESIAN_POINT('Ctrl Pts',(-0.0739708590293254,-0.0049213324513921,
-0.0649538702988953));
#41380=CARTESIAN_POINT('Ctrl Pts',(-0.0713218094908637,-0.0342663620749641,
-0.0624186997464803));
#41381=CARTESIAN_POINT('Ctrl Pts',(-0.0320784659707213,-0.081233120284334,
-0.0577672324125169));
#41382=CARTESIAN_POINT('Ctrl Pts',(0.0508239621622661,-0.0710211228679567,
-0.0514183420678718));
#41383=CARTESIAN_POINT('Ctrl Pts',(0.0872462569835861,0.00415522130723803,
-0.0450694517232264));
#41384=CARTESIAN_POINT('Ctrl Pts',(0.0438253963339189,0.0755444771434547,
-0.0387205613785811));
#41385=CARTESIAN_POINT('Ctrl Pts',(-0.0396344344718481,0.0777967966107338,
-0.0323716710339359));
#41386=CARTESIAN_POINT('Ctrl Pts',(-0.0727847520006691,0.0295357616972233,
-0.0279223985976627));
#41387=CARTESIAN_POINT('Ctrl Pts',(-0.0740171912190449,0.0025541606756479,
-0.025589422942938));
#41388=CARTESIAN_POINT('Ctrl Pts',(-0.0739977701941128,4.64298677421305E-5,
-0.0253727440697618));
#41389=CARTESIAN_POINT('Origin',(0.,0.,-1.25327725593024));
#41390=CARTESIAN_POINT('',(-0.0739349529908596,6.34005555056232E-5,-0.113277255930239));
#41391=CARTESIAN_POINT('',(-0.0737787977284999,-7.08850327115771E-7,-0.105372744069761));
#41392=CARTESIAN_POINT('',(-0.0739,1.16448635408261E-14,-1.25327725593024));
#41393=CARTESIAN_POINT('Ctrl Pts',(-0.0739349529908596,6.3400555505621E-5,
-0.113277255930239));
#41394=CARTESIAN_POINT('Ctrl Pts',(-0.0737536001066518,-0.0199120788385964,
-0.111553831779551));
#41395=CARTESIAN_POINT('Ctrl Pts',(-0.055087718801892,-0.0647152520185491,
-0.107714110847315));
#41396=CARTESIAN_POINT('Ctrl Pts',(0.0206440375741234,-0.0848624350572862,
-0.101758093133531));
#41397=CARTESIAN_POINT('Ctrl Pts',(0.082485545799834,-0.0287043654232375,
-0.0954092027888854));
#41398=CARTESIAN_POINT('Ctrl Pts',(0.0688673405223371,0.0537131333497329,
-0.0890603124442403));
#41399=CARTESIAN_POINT('Ctrl Pts',(-0.00775246097108719,0.0869925938161997,
-0.0827114220995948));
#41400=CARTESIAN_POINT('Ctrl Pts',(-0.0653665291881379,0.0486231069838693,
-0.0774504032615947));
#41401=CARTESIAN_POINT('Ctrl Pts',(-0.0737874569403616,0.0119895830276085,
-0.0743056812051428));
#41402=CARTESIAN_POINT('Ctrl Pts',(-0.0737792669902074,5.68230181076119E-6,
-0.0732772559302393));
#41403=CARTESIAN_POINT('Ctrl Pts',(-0.0737788473771473,-7.08559957466985E-7,
-0.105372744069761));
#41404=CARTESIAN_POINT('Ctrl Pts',(-0.0737799052710505,-0.0122877588686294,
-0.104318317654852));
#41405=CARTESIAN_POINT('Ctrl Pts',(-0.065052998623995,-0.0492342451664978,
-0.101147594458394));
#41406=CARTESIAN_POINT('Ctrl Pts',(-0.00668590821907806,-0.0870810566848186,
-0.0958605744803883));
#41407=CARTESIAN_POINT('Ctrl Pts',(0.0695201691859918,-0.0528652704077562,
-0.0895116841357433));
#41408=CARTESIAN_POINT('Ctrl Pts',(0.0821278409720519,0.0297127773219571,
-0.0831627937910981));
#41409=CARTESIAN_POINT('Ctrl Pts',(0.0196023809749374,0.0851091659979851,
-0.0768139034464528));
#41410=CARTESIAN_POINT('Ctrl Pts',(-0.0555464352803673,0.0641271511758735,
-0.070883886872674));
#41411=CARTESIAN_POINT('Ctrl Pts',(-0.0737456484315234,0.0196154933679126,
-0.0670701670804437));
#41412=CARTESIAN_POINT('Ctrl Pts',(-0.073926283611944,-6.48147617952535E-5,
-0.0653727440697618));
#41413=CARTESIAN_POINT('Origin',(0.,0.,-1.25327725593024));
#41414=CARTESIAN_POINT('',(-0.0739827363743306,-4.67140627613241E-5,-0.153277255930239));
#41415=CARTESIAN_POINT('',(-0.0739232992014367,6.5390844150956E-5,-0.145372744069761));
#41416=CARTESIAN_POINT('',(-0.0739,1.16448635408261E-14,-1.25327725593024));
#41417=CARTESIAN_POINT('Ctrl Pts',(-0.0739827363743306,-4.67140627613194E-5,
-0.153277255930239));
#41418=CARTESIAN_POINT('Ctrl Pts',(-0.0740034660210599,-0.00285479276065182,
-0.153034575917057));
#41419=CARTESIAN_POINT('Ctrl Pts',(-0.0725839529818503,-0.0301296296558551,
-0.150675599122327));
#41420=CARTESIAN_POINT('Ctrl Pts',(-0.0387070745970641,-0.0782915758141884,
-0.146200325546048));
#41421=CARTESIAN_POINT('Ctrl Pts',(0.0447628522836712,-0.0749939700395087,
-0.139851435201402));
#41422=CARTESIAN_POINT('Ctrl Pts',(0.087282643466595,-0.00309007448744508,
-0.133502544856757));
#41423=CARTESIAN_POINT('Ctrl Pts',(0.0499541717674709,0.071640695279081,
-0.127153654512112));
#41424=CARTESIAN_POINT('Ctrl Pts',(-0.0330735811680512,0.0808328325728891,
-0.120804764167467));
#41425=CARTESIAN_POINT('Ctrl Pts',(-0.0715199200215679,0.0336552600966897,
-0.116179297973509));
#41426=CARTESIAN_POINT('Ctrl Pts',(-0.0739762942849946,0.00461702082311773,
-0.1136701285611));
#41427=CARTESIAN_POINT('Ctrl Pts',(-0.0739349529908596,6.3400555505621E-5,
-0.113277255930239));
#41428=CARTESIAN_POINT('Ctrl Pts',(-0.0739232992014367,6.53908441509508E-5,
-0.145372744069761));
#41429=CARTESIAN_POINT('Ctrl Pts',(-0.07374309713053,-0.0195303985711661,
-0.143682765010809));
#41430=CARTESIAN_POINT('Ctrl Pts',(-0.0556773602240881,-0.0639588547833093,
-0.139876489170309));
#41431=CARTESIAN_POINT('Ctrl Pts',(0.019304037012885,-0.0851772417740305,
-0.13395391654826));
#41432=CARTESIAN_POINT('Ctrl Pts',(0.0820229322870143,-0.03000077385872,
-0.127605026203615));
#41433=CARTESIAN_POINT('Ctrl Pts',(0.0697052809023569,0.0526211209250912,
-0.12125613585897));
#41434=CARTESIAN_POINT('Ctrl Pts',(-0.00638045292204925,0.0871039537597873,
-0.114907245514324));
#41435=CARTESIAN_POINT('Ctrl Pts',(-0.0649622332078741,0.0494091429444137,
-0.109612781584588));
#41436=CARTESIAN_POINT('Ctrl Pts',(-0.0737777820148128,0.0123730848425035,
-0.1064346144364));
#41437=CARTESIAN_POINT('Ctrl Pts',(-0.0737788473771473,-7.08559957466985E-7,
-0.105372744069761));
#41438=CARTESIAN_POINT('Origin',(0.,0.,-1.25327725593024));
#41439=CARTESIAN_POINT('',(-0.0737931157698702,-3.29456842671063E-5,-0.193277255930239));
#41440=CARTESIAN_POINT('',(-0.0739916274709214,-4.14334611891637E-5,-0.185372744069761));
#41441=CARTESIAN_POINT('',(-0.0739,1.16448635408261E-14,-1.25327725593024));
#41442=CARTESIAN_POINT('Ctrl Pts',(-0.0737931157698702,-3.29456842671078E-5,
-0.193277255930238));
#41443=CARTESIAN_POINT('Ctrl Pts',(-0.0738342834808563,-0.0102618987148308,
-0.192399023273014));
#41444=CARTESIAN_POINT('Ctrl Pts',(-0.0670782543545674,-0.0450877822495248,
-0.189404493834241));
#41445=CARTESIAN_POINT('Ctrl Pts',(-0.0138849007021918,-0.0862265504199637,
-0.184293667613919));
#41446=CARTESIAN_POINT('Ctrl Pts',(0.0648964354273228,-0.058448790699953,
-0.177944777269274));
#41447=CARTESIAN_POINT('Ctrl Pts',(0.0843089497489975,0.0227993301675411,
-0.171595886924629));
#41448=CARTESIAN_POINT('Ctrl Pts',(0.0265936067550599,0.0831900747965725,
-0.165246996579983));
#41449=CARTESIAN_POINT('Ctrl Pts',(-0.0523141649508524,0.0680771702324626,
-0.15914078624852));
#41450=CARTESIAN_POINT('Ctrl Pts',(-0.0738226926475932,0.0216331237873961,
-0.155150872698605));
#41451=CARTESIAN_POINT('Ctrl Pts',(-0.0739827363743306,-4.67140627613194E-5,
-0.153277255930239));
#41452=CARTESIAN_POINT('Ctrl Pts',(-0.0739916274709214,-4.14334611891758E-5,
-0.185372744069761));
#41453=CARTESIAN_POINT('Ctrl Pts',(-0.0740078983074159,-0.00246175039700786,
-0.185163509148315));
#41454=CARTESIAN_POINT('Ctrl Pts',(-0.0728023110800164,-0.0293458401691555,
-0.18283797744532));
#41455=CARTESIAN_POINT('Ctrl Pts',(-0.0399361399802455,-0.0776718285893026,
-0.178396148960777));
#41456=CARTESIAN_POINT('Ctrl Pts',(0.0435753889642203,-0.0756901163504716,
-0.172047258616132));
#41457=CARTESIAN_POINT('Ctrl Pts',(0.0872231027375695,-0.00446526306300281,
-0.165698368271486));
#41458=CARTESIAN_POINT('Ctrl Pts',(0.0510770219946841,0.0708445203210023,
-0.159349477926841));
#41459=CARTESIAN_POINT('Ctrl Pts',(-0.031795548652228,0.0813440307632768,
-0.153000587582196));
#41460=CARTESIAN_POINT('Ctrl Pts',(-0.0712639647312324,0.0344415315961151,
-0.148341676296503));
#41461=CARTESIAN_POINT('Ctrl Pts',(-0.0739687573602636,0.00500866648521042,
-0.145799061792358));
#41462=CARTESIAN_POINT('Ctrl Pts',(-0.0739232992014367,6.53908441509508E-5,
-0.145372744069761));
#41463=CARTESIAN_POINT('Origin',(0.,0.,-1.25327725593024));
#41464=CARTESIAN_POINT('',(-0.0738624655248401,6.50487107154854E-5,-0.233277255930239));
#41465=CARTESIAN_POINT('',(-0.0737987845039503,-3.83921374419449E-5,-0.225372744069761));
#41466=CARTESIAN_POINT('',(-0.0739,1.16448635408261E-14,-1.25327725593024));
#41467=CARTESIAN_POINT('Ctrl Pts',(-0.0738624655248401,6.50487107154811E-5,
-0.233277255930239));
#41468=CARTESIAN_POINT('Ctrl Pts',(-0.0737133429813345,-0.0175246640909993,
-0.231763470628971));
#41469=CARTESIAN_POINT('Ctrl Pts',(-0.058619291546274,-0.0599350351261229,
-0.228133388546155));
#41470=CARTESIAN_POINT('Ctrl Pts',(0.0121734464516189,-0.0864847712974369,
-0.222387009681791));
#41471=CARTESIAN_POINT('Ctrl Pts',(0.0792522861301636,-0.0366999129159682,
-0.216038119337145));
#41472=CARTESIAN_POINT('Ctrl Pts',(0.0738292261096514,0.046658909512726,
-0.2096892289925));
#41473=CARTESIAN_POINT('Ctrl Pts',(0.000865412281594935,0.0873330380008177,
-0.203340338647855));
#41474=CARTESIAN_POINT('Ctrl Pts',(-0.0626876098657592,0.0535380781434799,
-0.197869680960434));
#41475=CARTESIAN_POINT('Ctrl Pts',(-0.0737350807313948,0.0143870370758291,
-0.194515320054562));
#41476=CARTESIAN_POINT('Ctrl Pts',(-0.0737931157698702,-3.29456842671078E-5,
-0.193277255930238));
#41477=CARTESIAN_POINT('Ctrl Pts',(-0.0737987845039503,-3.83921374419458E-5,
-0.225372744069761));
#41478=CARTESIAN_POINT('Ctrl Pts',(-0.0738451402008693,-0.00987591182851651,
-0.224527956504272));
#41479=CARTESIAN_POINT('Ctrl Pts',(-0.0674366951185759,-0.0442996935847633,
-0.221566872157234));
#41480=CARTESIAN_POINT('Ctrl Pts',(-0.015242104357177,-0.0859970144113175,
-0.216489491028649));
#41481=CARTESIAN_POINT('Ctrl Pts',(0.0639672230445058,-0.0594642969265874,
-0.210140600684003));
#41482=CARTESIAN_POINT('Ctrl Pts',(0.0846577945115181,0.0214677912515853,
-0.203791710339358));
#41483=CARTESIAN_POINT('Ctrl Pts',(0.0279013770542819,0.0827606270598339,
-0.197442819994713));
#41484=CARTESIAN_POINT('Ctrl Pts',(-0.0516682189334046,0.0688172291131411,
-0.191303164571514));
#41485=CARTESIAN_POINT('Ctrl Pts',(-0.0738433276962178,0.0220184315257577,
-0.187279805929863));
#41486=CARTESIAN_POINT('Ctrl Pts',(-0.0739916274709214,-4.14334611891758E-5,
-0.185372744069761));
#41487=CARTESIAN_POINT('Origin',(0.,0.,-1.25327725593024));
#41488=CARTESIAN_POINT('',(-0.0740200911805013,-7.10989654978704E-6,-0.273277255930238));
#41489=CARTESIAN_POINT('',(-0.0738517712133742,6.30027790375354E-5,-0.265372744069761));
#41490=CARTESIAN_POINT('',(-0.0739,1.16448635408261E-14,-1.25327725593024));
#41491=CARTESIAN_POINT('Ctrl Pts',(-0.0740200911805012,-7.10989654978785E-6,
-0.273277255930238));
#41492=CARTESIAN_POINT('Ctrl Pts',(-0.0740206153105398,-0.000388921978886646,
-0.273244214766476));
#41493=CARTESIAN_POINT('Ctrl Pts',(-0.0738450493612621,-0.0252254210660426,
-0.271094876821166));
#41494=CARTESIAN_POINT('Ctrl Pts',(-0.04624019674556,-0.074092190342946,
-0.266829242094308));
#41495=CARTESIAN_POINT('Ctrl Pts',(0.0371479911127987,-0.0790432490549754,
-0.260480351749662));
#41496=CARTESIAN_POINT('Ctrl Pts',(0.0865523022001051,-0.0116836402180771,
-0.254131461405018));
#41497=CARTESIAN_POINT('Ctrl Pts',(0.0567764831078735,0.0663644440252806,
-0.247782571060372));
#41498=CARTESIAN_POINT('Ctrl Pts',(-0.0249398298746646,0.083700736858798,
-0.241433680715727));
#41499=CARTESIAN_POINT('Ctrl Pts',(-0.0697966989192059,0.0385891993466075,
-0.236598575672349));
#41500=CARTESIAN_POINT('Ctrl Pts',(-0.0739218187530394,0.00706604408899114,
-0.23387976741052));
#41501=CARTESIAN_POINT('Ctrl Pts',(-0.0738624655248401,6.50487107154811E-5,
-0.233277255930239));
#41502=CARTESIAN_POINT('Ctrl Pts',(-0.0738517712133742,6.30027790375388E-5,
-0.265372744069761));
#41503=CARTESIAN_POINT('Ctrl Pts',(-0.0737120444937011,-0.01714439698726,
-0.263892403860229));
#41504=CARTESIAN_POINT('Ctrl Pts',(-0.0591470434262601,-0.0591647511335928,
-0.260295766869149));
#41505=CARTESIAN_POINT('Ctrl Pts',(0.0108089364983639,-0.086665882126032,
-0.25458283309652));
#41506=CARTESIAN_POINT('Ctrl Pts',(0.0786640523710499,-0.0379443684553606,
-0.248233942751875));
#41507=CARTESIAN_POINT('Ctrl Pts',(0.0745553989520529,0.045489567155642,
-0.24188505240723));
#41508=CARTESIAN_POINT('Ctrl Pts',(0.00224167132305463,0.087308551371477,
-0.235536162062585));
#41509=CARTESIAN_POINT('Ctrl Pts',(-0.0622278064411262,0.0543189253670649,
-0.230032059283428));
#41510=CARTESIAN_POINT('Ctrl Pts',(-0.0737290134771772,0.0147682852585804,
-0.22664425328582));
#41511=CARTESIAN_POINT('Ctrl Pts',(-0.0737987845039503,-3.83921374419458E-5,
-0.225372744069761));
#41512=CARTESIAN_POINT('Origin',(0.,0.,-1.25327725593024));
#41513=CARTESIAN_POINT('',(-0.0738418054104652,-6.0444388606692E-5,-0.313277255930238));
#41514=CARTESIAN_POINT('',(-0.0740209430351333,8.71191224640759E-8,-0.305372744069761));
#41515=CARTESIAN_POINT('',(-0.0739,1.16448635408261E-14,-1.25327725593024));
#41516=CARTESIAN_POINT('Ctrl Pts',(-0.0738418054104652,-6.04443886067091E-5,
-0.313277255930238));
#41517=CARTESIAN_POINT('Ctrl Pts',(-0.073901771058743,-0.00783479649662774,
-0.312608662122434));
#41518=CARTESIAN_POINT('Ctrl Pts',(-0.0691933312609605,-0.0401464863470307,
-0.309823771533081));
#41519=CARTESIAN_POINT('Ctrl Pts',(-0.0223216715032739,-0.0844366712168558,
-0.304922584162179));
#41520=CARTESIAN_POINT('Ctrl Pts',(0.0588152484367718,-0.0645645027565787,
-0.298573693817534));
#41521=CARTESIAN_POINT('Ctrl Pts',(0.0861465628713941,0.0143728274994348,
-0.292224803472889));
#41522=CARTESIAN_POINT('Ctrl Pts',(0.0346689272343444,0.0801615490700074,
-0.285875913128243));
#41523=CARTESIAN_POINT('Ctrl Pts',(-0.0480917181638159,0.0726558212856807,
-0.27956006394736));
#41524=CARTESIAN_POINT('Ctrl Pts',(-0.0739870446190946,0.0240662602546987,
-0.275360511548025));
#41525=CARTESIAN_POINT('Ctrl Pts',(-0.0740200911805012,-7.10989654978785E-6,
-0.273277255930238));
#41526=CARTESIAN_POINT('Ctrl Pts',(-0.0740209430351333,8.71191224682221E-8,
-0.305372744069761));
#41527=CARTESIAN_POINT('Ctrl Pts',(-0.0740205148794295,-0.0244496669579938,
-0.303256851216186));
#41528=CARTESIAN_POINT('Ctrl Pts',(-0.0473968446054434,-0.0733546414550255,
-0.299024661581064));
#41529=CARTESIAN_POINT('Ctrl Pts',(0.0358976572459432,-0.0796188824159332,
-0.292676175164391));
#41530=CARTESIAN_POINT('Ctrl Pts',(0.0863574175401337,-0.0130462511361909,
-0.286327284819747));
#41531=CARTESIAN_POINT('Ctrl Pts',(0.0578153328344367,0.0654614048287443,
-0.279978394475101));
#41532=CARTESIAN_POINT('Ctrl Pts',(-0.0236176105063063,0.0840833913854678,
-0.273629504130456));
#41533=CARTESIAN_POINT('Ctrl Pts',(-0.0694950249696135,0.039377286418387,
-0.268760953995342));
#41534=CARTESIAN_POINT('Ctrl Pts',(-0.0739117980403768,0.00745532982536957,
-0.266008700641778));
#41535=CARTESIAN_POINT('Ctrl Pts',(-0.0738517712133742,6.30027790375388E-5,
-0.265372744069761));
#41536=CARTESIAN_POINT('Origin',(0.,0.,-1.25327725593024));
#41537=CARTESIAN_POINT('',(-0.073805155490977,4.33812301120649E-5,-0.353277255930238));
#41538=CARTESIAN_POINT('',(-0.0738520240961663,-6.3059175845967E-5,-0.345372744069761));
#41539=CARTESIAN_POINT('',(-0.0739,1.16448635408261E-14,-1.25327725593024));
#41540=CARTESIAN_POINT('Ctrl Pts',(-0.073805155490977,4.33812301120651E-5,
-0.353277255930238));
#41541=CARTESIAN_POINT('Ctrl Pts',(-0.0737238735552172,-0.0151400725974492,
-0.351973109478391));
#41542=CARTESIAN_POINT('Ctrl Pts',(-0.0617703018698818,-0.0550798102599285,
-0.348552666244995));
#41543=CARTESIAN_POINT('Ctrl Pts',(0.00358415316748011,-0.0872637514146367,
-0.343015926230051));
#41544=CARTESIAN_POINT('Ctrl Pts',(0.0752461815192336,-0.0443375758432733,
-0.336667035885405));
#41545=CARTESIAN_POINT('Ctrl Pts',(0.0780711911348368,0.0391496817314182,
-0.330318145540761));
#41546=CARTESIAN_POINT('Ctrl Pts',(0.00947479519341831,0.0868218677576465,
-0.323969255196115));
#41547=CARTESIAN_POINT('Ctrl Pts',(-0.0596527774820103,0.0584113509348891,
-0.318288958659274));
#41548=CARTESIAN_POINT('Ctrl Pts',(-0.0737119620791017,0.0167733230413832,
-0.314724958903982));
#41549=CARTESIAN_POINT('Ctrl Pts',(-0.0738418054104652,-6.04443886067091E-5,
-0.313277255930238));
#41550=CARTESIAN_POINT('Ctrl Pts',(-0.0738520240961663,-6.30591758459618E-5,
-0.345372744069761));
#41551=CARTESIAN_POINT('Ctrl Pts',(-0.0739120432883483,-0.00744593178717649,
-0.344737595353692));
#41552=CARTESIAN_POINT('Ctrl Pts',(-0.0695024008175162,-0.0393582484273959,
-0.341986149856075));
#41553=CARTESIAN_POINT('Ctrl Pts',(-0.0236496187649619,-0.0840743942302376,
-0.337118407576909));
#41554=CARTESIAN_POINT('Ctrl Pts',(0.0577904079373426,-0.0654834099856214,
-0.330769517232263));
#41555=CARTESIAN_POINT('Ctrl Pts',(0.086362377900638,0.0130133745145877,
-0.324420626887618));
#41556=CARTESIAN_POINT('Ctrl Pts',(0.0359279650068146,0.0796052106546962,
-0.318071736542973));
#41557=CARTESIAN_POINT('Ctrl Pts',(-0.0473742153988214,0.073372283242758,
-0.311722846198328));
#41558=CARTESIAN_POINT('Ctrl Pts',(-0.074018829535515,0.0244638436337662,
-0.307489848707257));
#41559=CARTESIAN_POINT('Ctrl Pts',(-0.074020943116869,4.75462372219806E-6,
-0.305373147997735));
#41560=CARTESIAN_POINT('Ctrl Pts',(-0.0740209430351333,8.71191224682221E-8,
-0.305372744069761));
#41561=CARTESIAN_POINT('Origin',(0.,0.,-1.25327725593024));
#41562=CARTESIAN_POINT('',(-0.0739994218128981,3.58154130656329E-5,-0.393277255930239));
#41563=CARTESIAN_POINT('',(-0.0737986371542887,3.82643731348629E-5,-0.385372744069761));
#41564=CARTESIAN_POINT('',(-0.0739,1.16448635408261E-14,-1.25327725593024));
#41565=CARTESIAN_POINT('Ctrl Pts',(-0.0739994218128981,3.58154130656275E-5,
-0.393277255930239));
#41566=CARTESIAN_POINT('Ctrl Pts',(-0.0738654336872465,-0.0223953451531454,
-0.391337556834348));
#41567=CARTESIAN_POINT('Ctrl Pts',(-0.0510278128527495,-0.0695361071795467,
-0.387281560956909));
#41568=CARTESIAN_POINT('Ctrl Pts',(0.0291708805188321,-0.082321735857788,
-0.381109268297923));
#41569=CARTESIAN_POINT('Ctrl Pts',(0.0849779436410596,-0.0201632725374741,
-0.374760377953277));
#41570=CARTESIAN_POINT('Ctrl Pts',(0.0630451377031669,0.0604410380194803,
-0.368411487608632));
#41571=CARTESIAN_POINT('Ctrl Pts',(-0.0165628782942129,0.0857524316127216,
-0.362062597263987));
#41572=CARTESIAN_POINT('Ctrl Pts',(-0.0677786767413996,0.0435304809960098,
-0.357017853371189));
#41573=CARTESIAN_POINT('Ctrl Pts',(-0.0738557733880947,0.00949879708052387,
-0.35408940625994));
#41574=CARTESIAN_POINT('Ctrl Pts',(-0.073805155490977,4.33812301120651E-5,
-0.353277255930238));
#41575=CARTESIAN_POINT('Ctrl Pts',(-0.0737986371542887,3.82643731348673E-5,
-0.385372744069761));
#41576=CARTESIAN_POINT('Ctrl Pts',(-0.0737291507439404,-0.0147590795369847,
-0.384102042709649));
#41577=CARTESIAN_POINT('Ctrl Pts',(-0.0622390202126849,-0.0543000773339284,
-0.380715044567989));
#41578=CARTESIAN_POINT('Ctrl Pts',(0.00220843339423072,-0.0873093984336892,
-0.375211749644781));
#41579=CARTESIAN_POINT('Ctrl Pts',(0.0745380759834756,-0.0455179465880336,
-0.368862859300135));
#41580=CARTESIAN_POINT('Ctrl Pts',(0.0786784918314324,0.0379144188408675,
-0.36251396895549));
#41581=CARTESIAN_POINT('Ctrl Pts',(0.0108419288216904,0.0866617609579614,
-0.356165078610845));
#41582=CARTESIAN_POINT('Ctrl Pts',(-0.0591344093577337,0.0591833785993506,
-0.350451336982268));
#41583=CARTESIAN_POINT('Ctrl Pts',(-0.0737120611108954,0.0171535819182837,
-0.34685389213524));
#41584=CARTESIAN_POINT('Ctrl Pts',(-0.0738520240961663,-6.30591758459618E-5,
-0.345372744069761));
#41585=CARTESIAN_POINT('Origin',(0.,0.,-1.25327725593024));
#41586=CARTESIAN_POINT('',(-0.0739118163224249,-6.66974575854458E-5,-0.433277255930238));
#41587=CARTESIAN_POINT('',(-0.0739914229668183,4.15668966620335E-5,-0.42537274406976));
#41588=CARTESIAN_POINT('',(-0.0739,1.16448635408261E-14,-1.25327725593024));
#41589=CARTESIAN_POINT('Ctrl Pts',(-0.0739118163224248,-6.66974575854462E-5,
-0.433277255930238));
#41590=CARTESIAN_POINT('Ctrl Pts',(-0.0739609375286694,-0.00539053570481102,
-0.432818300971854));
#41591=CARTESIAN_POINT('Ctrl Pts',(-0.0710073599783538,-0.0352091741461071,
-0.430243049231921));
#41592=CARTESIAN_POINT('Ctrl Pts',(-0.0305407719561762,-0.0818234056563543,
-0.425551500710439));
#41593=CARTESIAN_POINT('Ctrl Pts',(0.0521605230517608,-0.0700506124159539,
-0.419202610365794));
#41594=CARTESIAN_POINT('Ctrl Pts',(0.0871441155782282,0.00580616783876835,
-0.412853720021149));
#41595=CARTESIAN_POINT('Ctrl Pts',(0.0424061727963488,0.0763513259455898,
-0.406504829676504));
#41596=CARTESIAN_POINT('Ctrl Pts',(-0.0411259579745188,0.0770484525838227,
-0.400155939331858));
#41597=CARTESIAN_POINT('Ctrl Pts',(-0.0730090199367733,0.0285814762061514,
-0.395746748083104));
#41598=CARTESIAN_POINT('Ctrl Pts',(-0.0740116206085493,0.00207803477121929,
-0.393453853615897));
#41599=CARTESIAN_POINT('Ctrl Pts',(-0.0739994218128981,3.58154130656275E-5,
-0.393277255930239));
#41600=CARTESIAN_POINT('Ctrl Pts',(-0.0739914229668183,4.15668966620296E-5,
-0.42537274406976));
#41601=CARTESIAN_POINT('Ctrl Pts',(-0.0738428054161868,-0.0220091137494347,
-0.423466490065606));
#41602=CARTESIAN_POINT('Ctrl Pts',(-0.0516839443637501,-0.068799393046605,
-0.419443939279904));
#41603=CARTESIAN_POINT('Ctrl Pts',(0.0278698686279614,-0.0827712429263309,
-0.413305091712652));
#41604=CARTESIAN_POINT('Ctrl Pts',(0.0846496157370046,-0.0215000183368973,
-0.406956201368007));
#41605=CARTESIAN_POINT('Ctrl Pts',(0.0639898560584943,0.0594399407345146,
-0.400607311023361));
#41606=CARTESIAN_POINT('Ctrl Pts',(-0.0152093647792003,0.0860028107443161,
-0.394258420678717));
#41607=CARTESIAN_POINT('Ctrl Pts',(-0.0674281327856323,0.0443187318135554,
-0.389180231694183));
#41608=CARTESIAN_POINT('Ctrl Pts',(-0.0738448772798502,0.00988524073800117,
-0.386218339491197));
#41609=CARTESIAN_POINT('Ctrl Pts',(-0.0737986371542887,3.82643731348673E-5,
-0.385372744069761));
#41610=CARTESIAN_POINT('Origin',(0.,0.,-1.25327725593024));
#41611=CARTESIAN_POINT('',(-0.0737794295953435,6.93418815541041E-6,-0.473277255930238));
#41612=CARTESIAN_POINT('',(-0.0739235825009513,-6.53505266424922E-5,-0.46537274406976));
#41613=CARTESIAN_POINT('',(-0.0739,1.16448635408261E-14,-1.25327725593024));
#41614=CARTESIAN_POINT('Ctrl Pts',(-0.0737794295953435,6.9341881554115E-6,
-0.473277255930238));
#41615=CARTESIAN_POINT('Ctrl Pts',(-0.0737687447719428,-0.0127469243178594,
-0.472182748327811));
#41616=CARTESIAN_POINT('Ctrl Pts',(-0.0645593346287235,-0.0501755960073792,
-0.468971943943835));
#41617=CARTESIAN_POINT('Ctrl Pts',(-0.0050400910778892,-0.0871917768302152,
-0.463644842778311));
#41618=CARTESIAN_POINT('Ctrl Pts',(0.070506311846667,-0.0515428797668893,
-0.457295952433666));
#41619=CARTESIAN_POINT('Ctrl Pts',(0.0815518429447203,0.0312586848284312,
-0.45094706208902));
#41620=CARTESIAN_POINT('Ctrl Pts',(0.0179917843980893,0.0854640518525547,
-0.444598171744375));
#41621=CARTESIAN_POINT('Ctrl Pts',(-0.0562430707592223,0.0632182791999014,
-0.438708236358114));
#41622=CARTESIAN_POINT('Ctrl Pts',(-0.0737344337099786,0.0191583258822792,
-0.434934597753402));
#41623=CARTESIAN_POINT('Ctrl Pts',(-0.0739118163224248,-6.66974575854462E-5,
-0.433277255930238));
#41624=CARTESIAN_POINT('Ctrl Pts',(-0.0739235825009513,-6.53505266424888E-5,
-0.46537274406976));
#41625=CARTESIAN_POINT('Ctrl Pts',(-0.0739689452559117,-0.00499921021186099,
-0.464947234203111));
#41626=CARTESIAN_POINT('Ctrl Pts',(-0.0712702306590702,-0.0344225349892039,
-0.462405427554914));
#41627=CARTESIAN_POINT('Ctrl Pts',(-0.0318265133113365,-0.0813319204454977,
-0.45774732412517));
#41628=CARTESIAN_POINT('Ctrl Pts',(0.0510500481910435,-0.070863959899244,
-0.451398433780523));
#41629=CARTESIAN_POINT('Ctrl Pts',(0.0872247963540974,0.00443205752395941,
-0.445049543435879));
#41630=CARTESIAN_POINT('Ctrl Pts',(0.0436042004922963,0.0756735220029905,
-0.438700653091233));
#41631=CARTESIAN_POINT('Ctrl Pts',(-0.0399065679425262,0.0776870263812308,
-0.432351762746588));
#41632=CARTESIAN_POINT('Ctrl Pts',(-0.0727971149138888,0.0293647663870503,
-0.427909126406097));
#41633=CARTESIAN_POINT('Ctrl Pts',(-0.0740077985615901,0.00247124636028123,
-0.425582786847154));
#41634=CARTESIAN_POINT('Ctrl Pts',(-0.0739914229668183,4.15668966620296E-5,
-0.42537274406976));
#41635=CARTESIAN_POINT('Origin',(0.,0.,-1.25327725593024));
#41636=CARTESIAN_POINT('',(-0.0739372416732134,6.29279406287392E-5,-0.513277255930238));
#41637=CARTESIAN_POINT('',(-0.0737788291172461,5.56757125268528E-7,-0.505372744069761));
#41638=CARTESIAN_POINT('',(-0.0739,1.16448635408261E-14,-1.25327725593024));
#41639=CARTESIAN_POINT('Ctrl Pts',(-0.0739372416732135,6.29279406287363E-5,
-0.513277255930238));
#41640=CARTESIAN_POINT('Ctrl Pts',(-0.0737558839958198,-0.0199878652888913,
-0.511547195683768));
#41641=CARTESIAN_POINT('Ctrl Pts',(-0.0549695186936256,-0.0648650221978919,
-0.50770083865575));
#41642=CARTESIAN_POINT('Ctrl Pts',(0.0209093093381367,-0.0847974601499693,
-0.501738184846182));
#41643=CARTESIAN_POINT('Ctrl Pts',(0.0825749204933152,-0.0284462821895266,
-0.495389294501537));
#41644=CARTESIAN_POINT('Ctrl Pts',(0.0686990060272686,0.0539282396870952,
-0.489040404156892));
#41645=CARTESIAN_POINT('Ctrl Pts',(-0.00802441338286892,0.0869679093386998,
-0.482691513812247));
#41646=CARTESIAN_POINT('Ctrl Pts',(-0.0654458135203799,0.0484671034431539,
-0.477437131070029));
#41647=CARTESIAN_POINT('Ctrl Pts',(-0.0737894045255381,0.0119134340467115,
-0.474299045109359));
#41648=CARTESIAN_POINT('Ctrl Pts',(-0.0737794295953435,6.9341881554115E-6,
-0.473277255930238));
#41649=CARTESIAN_POINT('Ctrl Pts',(-0.0737788400683315,5.56706807122026E-7,
-0.505372744069761));
#41650=CARTESIAN_POINT('Ctrl Pts',(-0.0737780088266581,-0.0123638253439393,
-0.504311681559069));
#41651=CARTESIAN_POINT('Ctrl Pts',(-0.0649721116611022,-0.0493901687656836,
-0.501134322266829));
#41652=CARTESIAN_POINT('Ctrl Pts',(-0.00641360530457873,-0.0871015149116623,
-0.49584066619304));
#41653=CARTESIAN_POINT('Ctrl Pts',(0.0696852396434252,-0.0526476553015217,
-0.489491775848395));
#41654=CARTESIAN_POINT('Ctrl Pts',(0.0820343493873717,0.0299695471020194,
-0.48314288550375));
#41655=CARTESIAN_POINT('Ctrl Pts',(0.0193364609744337,0.0851698861681384,
-0.476793995159104));
#41656=CARTESIAN_POINT('Ctrl Pts',(-0.0556632358337177,0.0639771560029762,
-0.470870614681109));
#41657=CARTESIAN_POINT('Ctrl Pts',(-0.0737433310931167,0.01953961295263,
-0.46706353098466));
#41658=CARTESIAN_POINT('Ctrl Pts',(-0.0739235825009513,-6.53505266424888E-5,
-0.46537274406976));
#41659=CARTESIAN_POINT('Origin',(0.,0.,-1.25327725593024));
#41660=CARTESIAN_POINT('',(-0.073980874458951,-4.77002733273939E-5,-0.553277255930238));
#41661=CARTESIAN_POINT('',(-0.0739256241017582,6.50482031668356E-5,-0.545372744069761));
#41662=CARTESIAN_POINT('',(-0.0739,1.16448635408261E-14,-1.25327725593024));
#41663=CARTESIAN_POINT('Ctrl Pts',(-0.0739808744589511,-4.77002733273914E-5,
-0.553277255930238));
#41664=CARTESIAN_POINT('Ctrl Pts',(-0.0740025130732811,-0.0029327564029972,
-0.553027939821274));
#41665=CARTESIAN_POINT('Ctrl Pts',(-0.0725398341957257,-0.0302852066985371,
-0.550662326930761));
#41666=CARTESIAN_POINT('Ctrl Pts',(-0.0384620532909962,-0.0784122370649128,
-0.5461804172587));
#41667=CARTESIAN_POINT('Ctrl Pts',(0.0449971529934493,-0.0748536217384812,
-0.539831526914054));
#41668=CARTESIAN_POINT('Ctrl Pts',(0.0872918802153685,-0.00281711081593204,
-0.533482636569409));
#41669=CARTESIAN_POINT('Ctrl Pts',(0.0497298934808031,0.0717965609153495,
-0.527133746224764));
#41670=CARTESIAN_POINT('Ctrl Pts',(-0.0333261972756367,0.0807290099036824,
-0.520784855880119));
#41671=CARTESIAN_POINT('Ctrl Pts',(-0.0715698711116002,0.0334992973532661,
-0.516166025781943));
#41672=CARTESIAN_POINT('Ctrl Pts',(-0.0739777298360213,0.00453927430968902,
-0.513663492465317));
#41673=CARTESIAN_POINT('Ctrl Pts',(-0.0739372416732135,6.29279406287363E-5,
-0.513277255930238));
#41674=CARTESIAN_POINT('Ctrl Pts',(-0.0739256241017582,6.50482031668361E-5,
-0.545372744069761));
#41675=CARTESIAN_POINT('Ctrl Pts',(-0.0737450480884514,-0.0196060964085107,
-0.543676128915026));
#41676=CARTESIAN_POINT('Ctrl Pts',(-0.0555611653360301,-0.064109143640121,
-0.539863216978743));
#41677=CARTESIAN_POINT('Ctrl Pts',(0.0195703062739464,-0.085116457546431,
-0.533934008260913));
#41678=CARTESIAN_POINT('Ctrl Pts',(0.0821163510431211,-0.0297441275594417,
-0.527585117916266));
#41679=CARTESIAN_POINT('Ctrl Pts',(0.0695403805661829,0.052838846539454,
-0.521236227571622));
#41680=CARTESIAN_POINT('Ctrl Pts',(-0.00665280454283421,0.0870835714967197,
-0.514887337226976));
#41681=CARTESIAN_POINT('Ctrl Pts',(-0.0650431584057082,0.0492532338086213,
-0.509599509393023));
#41682=CARTESIAN_POINT('Ctrl Pts',(-0.0737796667441326,0.0122970232640985,
-0.506427978340618));
#41683=CARTESIAN_POINT('Ctrl Pts',(-0.0737788400683315,5.56706807122026E-7,
-0.505372744069761));
#41684=CARTESIAN_POINT('Origin',(0.,0.,-1.25327725593024));
#41685=CARTESIAN_POINT('',(-0.0737920974294479,-3.18290494924771E-5,-0.593277255930238));
#41686=CARTESIAN_POINT('',(-0.0739899318680459,-4.25211598454808E-5,-0.585372744069761));
#41687=CARTESIAN_POINT('',(-0.0739,1.16448635408261E-14,-1.25327725593024));
#41688=CARTESIAN_POINT('Ctrl Pts',(-0.0737920974294479,-3.18290494924836E-5,
-0.593277255930238));
#41689=CARTESIAN_POINT('Ctrl Pts',(-0.0738321381747954,-0.0103384296985671,
-0.592392387177231));
#41690=CARTESIAN_POINT('Ctrl Pts',(-0.06700616371982,-0.0452441277251543,
-0.589391221642675));
#41691=CARTESIAN_POINT('Ctrl Pts',(-0.0136151867463331,-0.0862695494061835,
-0.584273759326571));
#41692=CARTESIAN_POINT('Ctrl Pts',(0.06507889807261,-0.058245561981479,
-0.577924868981926));
#41693=CARTESIAN_POINT('Ctrl Pts',(0.0842372398743852,0.0230628680616442,
-0.57157597863728));
#41694=CARTESIAN_POINT('Ctrl Pts',(0.0263333262574912,0.083272831062118,
-0.565227088292636));
#41695=CARTESIAN_POINT('Ctrl Pts',(-0.0524410953307806,0.0679299339365414,
-0.559127514056954));
#41696=CARTESIAN_POINT('Ctrl Pts',(-0.0738188356925693,0.0215567762917269,
-0.555144236602822));
#41697=CARTESIAN_POINT('Ctrl Pts',(-0.0739808744589511,-4.77002733273914E-5,
-0.553277255930238));
#41698=CARTESIAN_POINT('Ctrl Pts',(-0.0739899318680459,-4.25211598455012E-5,
-0.585372744069761));
#41699=CARTESIAN_POINT('Ctrl Pts',(-0.0740070680983731,-0.0025397515316431,
-0.585156873052532));
#41700=CARTESIAN_POINT('Ctrl Pts',(-0.0727595129678202,-0.0295013175423853,
-0.582824705253755));
#41701=CARTESIAN_POINT('Ctrl Pts',(-0.0396930507999507,-0.0777963363604095,
-0.578376240673428));
#41702=CARTESIAN_POINT('Ctrl Pts',(0.0438118725954223,-0.0755534780972525,
-0.572027350328785));
#41703=CARTESIAN_POINT('Ctrl Pts',(0.0872366399772161,-0.00419247878885715,
-0.565678459984137));
#41704=CARTESIAN_POINT('Ctrl Pts',(0.0508552285025388,0.0710039010679274,
-0.559329569639494));
#41705=CARTESIAN_POINT('Ctrl Pts',(-0.0320497705692809,0.0812442024969535,
-0.552980679294847));
#41706=CARTESIAN_POINT('Ctrl Pts',(-0.0713153122300141,0.0342854907512878,
-0.548328404104937));
#41707=CARTESIAN_POINT('Ctrl Pts',(-0.0739702921190258,0.00493098256010466,
-0.545792425696575));
#41708=CARTESIAN_POINT('Ctrl Pts',(-0.0739256241017582,6.50482031668361E-5,
-0.545372744069761));
#41709=CARTESIAN_POINT('Origin',(0.,0.,-1.25327725593024));
#41710=CARTESIAN_POINT('',(-0.0738646379472932,6.53830851695627E-5,-0.633277255930239));
#41711=CARTESIAN_POINT('',(-0.0737975891722939,-3.73368331001503E-5,-0.625372744069761));
#41712=CARTESIAN_POINT('',(-0.0739,1.16448635408261E-14,-1.25327725593024));
#41713=CARTESIAN_POINT('Ctrl Pts',(-0.0738646379472931,6.53830851695594E-5,
-0.633277255930239));
#41714=CARTESIAN_POINT('Ctrl Pts',(-0.0737137520287097,-0.0176001212798387,
-0.631756834533189));
#41715=CARTESIAN_POINT('Ctrl Pts',(-0.0585134263150157,-0.0600876505745179,
-0.62812011635459));
#41716=CARTESIAN_POINT('Ctrl Pts',(0.0124438404931729,-0.0864462798428249,
-0.622367101394442));
#41717=CARTESIAN_POINT('Ctrl Pts',(0.0793666658984961,-0.0364518971939734,
-0.616018211049798));
#41718=CARTESIAN_POINT('Ctrl Pts',(0.073682954238757,0.0468895587474729,
-0.609669320705152));
#41719=CARTESIAN_POINT('Ctrl Pts',(0.000592301800611145,0.087335317274631,
-0.603320430360507));
#41720=CARTESIAN_POINT('Ctrl Pts',(-0.0627777631997439,0.053383016163664,
-0.59785640876887));
#41721=CARTESIAN_POINT('Ctrl Pts',(-0.0737363747067989,0.0143113567338424,
-0.59450868395878));
#41722=CARTESIAN_POINT('Ctrl Pts',(-0.0737920974294479,-3.18290494924836E-5,
-0.593277255930238));
#41723=CARTESIAN_POINT('Ctrl Pts',(-0.0737975891722939,-3.73368331001503E-5,
-0.625372744069761));
#41724=CARTESIAN_POINT('Ctrl Pts',(-0.0738429811604534,-0.00995253562942452,
-0.624521320408489));
#41725=CARTESIAN_POINT('Ctrl Pts',(-0.0673662201976671,-0.0444560792889662,
-0.62155359996567));
#41726=CARTESIAN_POINT('Ctrl Pts',(-0.0149731015673857,-0.0860442587414302,
-0.6164695827413));
#41727=CARTESIAN_POINT('Ctrl Pts',(0.0641528659084539,-0.0592639690591287,
-0.610120692396656));
#41728=CARTESIAN_POINT('Ctrl Pts',(0.0845902468891876,0.0217324265588487,
-0.60377180205201));
#41729=CARTESIAN_POINT('Ctrl Pts',(0.027642433133917,0.0828474750571577,
-0.597422911707366));
#41730=CARTESIAN_POINT('Ctrl Pts',(-0.0517972143618181,0.0686706564364598,
-0.591289892379948));
#41731=CARTESIAN_POINT('Ctrl Pts',(-0.0738390726464825,0.0219419073147564,
-0.58727316983408));
#41732=CARTESIAN_POINT('Ctrl Pts',(-0.0739899318680459,-4.25211598455012E-5,
-0.585372744069761));
#41733=CARTESIAN_POINT('Origin',(0.,0.,-1.25327725593024));
#41734=CARTESIAN_POINT('',(-0.0740197207812738,-8.52928078186594E-6,-0.673277255930238));
#41735=CARTESIAN_POINT('',(-0.0738538568161215,6.34559343100465E-5,-0.665372744069761));
#41736=CARTESIAN_POINT('',(-0.0739,1.16448635408261E-14,-1.25327725593024));
#41737=CARTESIAN_POINT('Ctrl Pts',(-0.0740197207812738,-8.5292807818521E-6,
-0.673277255930238));
#41738=CARTESIAN_POINT('Ctrl Pts',(-0.0740204699529474,-0.00046703193262174,
-0.673237578670693));
#41739=CARTESIAN_POINT('Ctrl Pts',(-0.073808986523765,-0.0253803366732234,
-0.671081604629601));
#41740=CARTESIAN_POINT('Ctrl Pts',(-0.0460082709303986,-0.0742364295402099,
-0.66680933380696));
#41741=CARTESIAN_POINT('Ctrl Pts',(0.037394992047993,-0.0789266940560291,
-0.660460443462315));
#41742=CARTESIAN_POINT('Ctrl Pts',(0.0865884158521809,-0.0114129183425305,
-0.654111553117668));
#41743=CARTESIAN_POINT('Ctrl Pts',(0.0565686718383231,0.0665416698868583,
-0.647762662773025));
#41744=CARTESIAN_POINT('Ctrl Pts',(-0.0252014553124982,0.0836223362207471,
-0.641413772428377));
#41745=CARTESIAN_POINT('Ctrl Pts',(-0.0698556617272321,0.0384328507297029,
-0.636585303480784));
#41746=CARTESIAN_POINT('Ctrl Pts',(-0.0739237723457736,0.00698875263671575,
-0.633873131314737));
#41747=CARTESIAN_POINT('Ctrl Pts',(-0.0738646379472931,6.53830851695594E-5,
-0.633277255930239));
#41748=CARTESIAN_POINT('Ctrl Pts',(-0.0738538568161215,6.34559343100473E-5,
-0.665372744069761));
#41749=CARTESIAN_POINT('Ctrl Pts',(-0.0737122022775332,-0.0172198463724857,
-0.663885767764447));
#41750=CARTESIAN_POINT('Ctrl Pts',(-0.0590430950891427,-0.0593177345607098,
-0.660282494677584));
#41751=CARTESIAN_POINT('Ctrl Pts',(0.011079903578258,-0.0866316568559436,
-0.654562924809171));
#41752=CARTESIAN_POINT('Ctrl Pts',(0.0787823266538737,-0.0376981861620926,
-0.648214034464528));
#41753=CARTESIAN_POINT('Ctrl Pts',(0.0744127802759426,0.0457224929822708,
-0.641865144119881));
#41754=CARTESIAN_POINT('Ctrl Pts',(0.00196863068701841,0.0873151345765873,
-0.635516253775237));
#41755=CARTESIAN_POINT('Ctrl Pts',(-0.0623197635665918,0.0541640793943838,
-0.630018787091862));
#41756=CARTESIAN_POINT('Ctrl Pts',(-0.0737301549344281,0.0146926607111806,
-0.626637617190037));
#41757=CARTESIAN_POINT('Ctrl Pts',(-0.0737975891722939,-3.73368331001503E-5,
-0.625372744069761));
#41758=CARTESIAN_POINT('Origin',(0.,0.,-1.25327725593024));
#41759=CARTESIAN_POINT('',(-0.0738398419805284,-5.98587458514904E-5,-0.713277255930238));
#41760=CARTESIAN_POINT('',(-0.0740209121467327,-1.34404130546634E-6,-0.705372744069761));
#41761=CARTESIAN_POINT('',(-0.0739,1.16448635408261E-14,-1.25327725593024));
#41762=CARTESIAN_POINT('Ctrl Pts',(-0.0738398419805284,-5.98587458514712E-5,
-0.713277255930238));
#41763=CARTESIAN_POINT('Ctrl Pts',(-0.0738997053742793,-0.00791190180289649,
-0.712602026026651));
#41764=CARTESIAN_POINT('Ctrl Pts',(-0.0691310979633685,-0.0403029009963255,
-0.709810499341516));
#41765=CARTESIAN_POINT('Ctrl Pts',(-0.0220575135733365,-0.0845060622668312,
-0.704902675874831));
#41766=CARTESIAN_POINT('Ctrl Pts',(0.0590168657611575,-0.064380261110165,
-0.698553785530186));
#41767=CARTESIAN_POINT('Ctrl Pts',(0.0861011952070565,0.0146421531476717,
-0.692204895185541));
#41768=CARTESIAN_POINT('Ctrl Pts',(0.0344180780130461,0.080269573131862,
-0.685856004840895));
#41769=CARTESIAN_POINT('Ctrl Pts',(-0.0482317589869109,0.0725132326990022,
-0.679546791755795));
#41770=CARTESIAN_POINT('Ctrl Pts',(-0.0739805108020415,0.0239884798028173,
-0.675353875452242));
#41771=CARTESIAN_POINT('Ctrl Pts',(-0.0740197207812738,-8.5292807818521E-6,
-0.673277255930238));
#41772=CARTESIAN_POINT('Ctrl Pts',(-0.0740209121467327,-1.34404130547942E-6,
-0.705372744069761));
#41773=CARTESIAN_POINT('Ctrl Pts',(-0.0740209314587002,-7.33586246526099E-5,
-0.705366511901952));
#41774=CARTESIAN_POINT('Ctrl Pts',(-0.0739882313484256,-0.0245998043267833,
-0.703243982952595));
#41775=CARTESIAN_POINT('Ctrl Pts',(-0.047172520489486,-0.0735021193135168,
-0.699005157221689));
#41776=CARTESIAN_POINT('Ctrl Pts',(0.0361464644047429,-0.0795062346231174,
-0.692656266877045));
#41777=CARTESIAN_POINT('Ctrl Pts',(0.0863977932766005,-0.0127761320376415,
-0.686307376532398));
#41778=CARTESIAN_POINT('Ctrl Pts',(0.0576103404526291,0.065641883777369,
-0.679958486187753));
#41779=CARTESIAN_POINT('Ctrl Pts',(-0.0238804390394198,0.0840091236961439,
-0.673609595843108));
#41780=CARTESIAN_POINT('Ctrl Pts',(-0.0695554825620404,0.0392209024120294,
-0.668747681803777));
#41781=CARTESIAN_POINT('Ctrl Pts',(-0.0739138080751741,0.00737812261711985,
-0.666002064545995));
#41782=CARTESIAN_POINT('Ctrl Pts',(-0.0738538568161215,6.34559343100473E-5,
-0.665372744069761));
#41783=CARTESIAN_POINT('Origin',(0.,0.,-1.25327725593024));
#41784=CARTESIAN_POINT('',(-0.0738065481177383,4.4352265423165E-5,-0.753277255930239));
#41785=CARTESIAN_POINT('',(-0.0738499552817868,-6.25858527072351E-5,-0.745372744069761));
#41786=CARTESIAN_POINT('',(-0.0739,1.16448635408261E-14,-1.25327725593024));
#41787=CARTESIAN_POINT('Ctrl Pts',(-0.0738065481177383,4.43522654231662E-5,
-0.753277255930239));
#41788=CARTESIAN_POINT('Ctrl Pts',(-0.0737229278950059,-0.0152156401028241,
-0.751966473382609));
#41789=CARTESIAN_POINT('Ctrl Pts',(-0.06167620653198,-0.0552343787480568,
-0.74853939405343));
#41790=CARTESIAN_POINT('Ctrl Pts',(0.00385702521968538,-0.0872521164289911,
-0.742996017942701));
#41791=CARTESIAN_POINT('Ctrl Pts',(0.0753844652332581,-0.0441020505915453,
-0.736647127598059));
#41792=CARTESIAN_POINT('Ctrl Pts',(0.0779483812393019,0.0393936330776424,
-0.730298237253411));
#41793=CARTESIAN_POINT('Ctrl Pts',(0.00920324113794826,0.086851072632641,
-0.723949346908768));
#41794=CARTESIAN_POINT('Ctrl Pts',(-0.059754493504533,0.0582579636900757,
-0.718275686467709));
#41795=CARTESIAN_POINT('Ctrl Pts',(-0.0737120823041892,0.0166978694200925,
-0.714718322808199));
#41796=CARTESIAN_POINT('Ctrl Pts',(-0.0738398419805284,-5.98587458514712E-5,
-0.713277255930238));
#41797=CARTESIAN_POINT('Ctrl Pts',(-0.0738499552817868,-6.25858527072334E-5,
-0.745372744069761));
#41798=CARTESIAN_POINT('Ctrl Pts',(-0.0739100242568725,-0.00752312406464893,
-0.74473095925791));
#41799=CARTESIAN_POINT('Ctrl Pts',(-0.0694416811052649,-0.0395146377430722,
-0.74197287766451));
#41800=CARTESIAN_POINT('Ctrl Pts',(-0.0233865872476794,-0.084147939783551,
-0.737098499289559));
#41801=CARTESIAN_POINT('Ctrl Pts',(0.0579949038623966,-0.0653023687081939,
-0.730749608944917));
#41802=CARTESIAN_POINT('Ctrl Pts',(0.0863212604370854,0.0132833817028017,
-0.724400718600269));
#41803=CARTESIAN_POINT('Ctrl Pts',(0.035678849400398,0.079717174676309,
-0.718051828255625));
#41804=CARTESIAN_POINT('Ctrl Pts',(-0.0475216810321705,0.0732301507334676,
-0.711709170078789));
#41805=CARTESIAN_POINT('Ctrl Pts',(-0.0740143735713409,0.0243810905554448,
-0.707482808683501));
#41806=CARTESIAN_POINT('Ctrl Pts',(-0.0740209121467327,-1.34404130547942E-6,
-0.705372744069761));
#41807=CARTESIAN_POINT('Origin',(0.,0.,-1.25327725593024));
#41808=CARTESIAN_POINT('',(-0.074000888164484,3.46214213901279E-5,-0.793277255930238));
#41809=CARTESIAN_POINT('',(-0.0737998625275067,3.93079929045179E-5,-0.785372744069761));
#41810=CARTESIAN_POINT('',(-0.0739,1.16448635408261E-14,-1.25327725593024));
#41811=CARTESIAN_POINT('Ctrl Pts',(-0.074000888164484,3.46214213901347E-5,
-0.793277255930238));
#41812=CARTESIAN_POINT('Ctrl Pts',(-0.0738701707844107,-0.0224721008728551,
-0.791330920738565));
#41813=CARTESIAN_POINT('Ctrl Pts',(-0.0508963789367996,-0.0696818637307418,
-0.787268288765345));
#41814=CARTESIAN_POINT('Ctrl Pts',(0.0294281728820954,-0.0822301106998219,
-0.781089360010573));
#41815=CARTESIAN_POINT('Ctrl Pts',(0.0850405823393773,-0.0198974325042983,
-0.77474046966593));
#41816=CARTESIAN_POINT('Ctrl Pts',(0.0628558193470167,0.0606378960642491,
-0.768391579321283));
#41817=CARTESIAN_POINT('Ctrl Pts',(-0.0168309607139535,0.0857002171895078,
-0.762042688976639));
#41818=CARTESIAN_POINT('Ctrl Pts',(-0.0678472753579036,0.0433740631041454,
-0.757004581179623));
#41819=CARTESIAN_POINT('Ctrl Pts',(-0.0738579351916478,0.00942206414016046,
-0.754082770164157));
#41820=CARTESIAN_POINT('Ctrl Pts',(-0.0738065481177383,4.43522654231662E-5,
-0.753277255930239));
#41821=CARTESIAN_POINT('Ctrl Pts',(-0.0737998625275067,3.93079929045092E-5,
-0.785372744069761));
#41822=CARTESIAN_POINT('Ctrl Pts',(-0.0737280372000447,-0.014834695020822,
-0.784095406613867));
#41823=CARTESIAN_POINT('Ctrl Pts',(-0.0621467471385402,-0.0544548837730268,
-0.780701772376424));
#41824=CARTESIAN_POINT('Ctrl Pts',(0.00248145491972144,-0.0873020653500868,
-0.775191841357431));
#41825=CARTESIAN_POINT('Ctrl Pts',(0.0746800543932818,-0.0452846299391521,
-0.768842951012788));
#41826=CARTESIAN_POINT('Ctrl Pts',(0.0785595418575094,0.0381602753665082,
-0.762494060668141));
#41827=CARTESIAN_POINT('Ctrl Pts',(0.0105708687644261,0.0866952418906293,
-0.756145170323498));
#41828=CARTESIAN_POINT('Ctrl Pts',(-0.0592380251362248,0.0590303333329511,
-0.750438064790702));
#41829=CARTESIAN_POINT('Ctrl Pts',(-0.0737119457478501,0.0170781327974444,
-0.746847256039458));
#41830=CARTESIAN_POINT('Ctrl Pts',(-0.0738499552817868,-6.25858527072334E-5,
-0.745372744069761));
#41831=CARTESIAN_POINT('Origin',(0.,0.,-1.25327725593024));
#41832=CARTESIAN_POINT('',(-0.0739094769521497,-6.68860282600848E-5,-0.833277255930239));
#41833=CARTESIAN_POINT('',(-0.0739930868845781,4.0462490936608E-5,-0.825372744069761));
#41834=CARTESIAN_POINT('',(-0.0739,1.16448635408261E-14,-1.25327725593024));
#41835=CARTESIAN_POINT('Ctrl Pts',(-0.0739094769521496,-6.68860282600822E-5,
-0.833277255930239));
#41836=CARTESIAN_POINT('Ctrl Pts',(-0.0739592933962805,-0.005468140800202,
-0.832811664876072));
#41837=CARTESIAN_POINT('Ctrl Pts',(-0.0709543523443195,-0.0353652993575146,
-0.830229777040356));
#41838=CARTESIAN_POINT('Ctrl Pts',(-0.0302847459931343,-0.081918512102057,
-0.825531592423091));
#41839=CARTESIAN_POINT('Ctrl Pts',(0.0523793289752858,-0.0698871544776452,
-0.819182702078447));
#41840=CARTESIAN_POINT('Ctrl Pts',(0.0871255325346814,0.00607865490315511,
-0.812833811733801));
#41841=CARTESIAN_POINT('Ctrl Pts',(0.0421672010014363,0.0764835644082308,
-0.806484921389155));
#41842=CARTESIAN_POINT('Ctrl Pts',(-0.041366701368516,0.0769194675148722,
-0.800136031044511));
#41843=CARTESIAN_POINT('Ctrl Pts',(-0.0730502848478739,0.0284261194000154,
-0.795733475891537));
#41844=CARTESIAN_POINT('Ctrl Pts',(-0.074012302916597,0.00199999630665251,
-0.793447217520114));
#41845=CARTESIAN_POINT('Ctrl Pts',(-0.074000888164484,3.46214213901347E-5,
-0.793277255930238));
#41846=CARTESIAN_POINT('Ctrl Pts',(-0.0739930868845781,4.04624909366076E-5,
-0.825372744069761));
#41847=CARTESIAN_POINT('Ctrl Pts',(-0.0738471310185028,-0.0220856706569688,
-0.823459853969824));
#41848=CARTESIAN_POINT('Ctrl Pts',(-0.0515545879708975,-0.0689458471408334,
-0.819430667088338));
#41849=CARTESIAN_POINT('Ctrl Pts',(0.0281285730428364,-0.0826836840705789,
-0.813285183425303));
#41850=CARTESIAN_POINT('Ctrl Pts',(0.0847164362872849,-0.0212351985084165,
-0.80693629308066));
#41851=CARTESIAN_POINT('Ctrl Pts',(0.0638036636957854,0.0596397579799298,
-0.800587402736013));
#41852=CARTESIAN_POINT('Ctrl Pts',(-0.015478236798094,0.0859548277790816,
-0.794238512391369));
#41853=CARTESIAN_POINT('Ctrl Pts',(-0.0674983278290557,0.0441623403232539,
-0.789166959502617));
#41854=CARTESIAN_POINT('Ctrl Pts',(-0.0738470376322641,0.00980860073585892,
-0.786211703395415));
#41855=CARTESIAN_POINT('Ctrl Pts',(-0.0737998625275067,3.93079929045092E-5,
-0.785372744069761));
#41856=CARTESIAN_POINT('Origin',(0.,0.,-1.25327725593024));
#41857=CARTESIAN_POINT('',(-0.0737796652821541,8.19419257115589E-6,-0.873277255930239));
#41858=CARTESIAN_POINT('',(-0.0739212535704956,-6.56703637913897E-5,-0.865372744069761));
#41859=CARTESIAN_POINT('',(-0.0739,1.16448635408261E-14,-1.25327725593024));
#41860=CARTESIAN_POINT('Ctrl Pts',(-0.0737796652821541,8.1941925711617E-6,
-0.873277255930239));
#41861=CARTESIAN_POINT('Ctrl Pts',(-0.0737669601095564,-0.0128228898212472,
-0.872176112232029));
#41862=CARTESIAN_POINT('Ctrl Pts',(-0.0644763991334308,-0.0503313595727542,
-0.868958671752271));
#41863=CARTESIAN_POINT('Ctrl Pts',(-0.00476740193378281,-0.087207111772408,
-0.863624934490961));
#41864=CARTESIAN_POINT('Ctrl Pts',(0.0706671510291381,-0.0513221417159152,
-0.857276044146319));
#41865=CARTESIAN_POINT('Ctrl Pts',(0.0814536926085207,0.0315135593883026,
-0.850927153801671));
#41866=CARTESIAN_POINT('Ctrl Pts',(0.0177244348341756,0.0855198975367287,
-0.844578263457028));
#41867=CARTESIAN_POINT('Ctrl Pts',(-0.0563569303426115,0.063067413190051,
-0.838694964166549));
#41868=CARTESIAN_POINT('Ctrl Pts',(-0.0737328578163039,0.0190827134051602,
-0.83492796165762));
#41869=CARTESIAN_POINT('Ctrl Pts',(-0.0739094769521496,-6.68860282600822E-5,
-0.833277255930239));
#41870=CARTESIAN_POINT('Ctrl Pts',(-0.0739212535704956,-6.56703637913767E-5,
-0.865372744069761));
#41871=CARTESIAN_POINT('Ctrl Pts',(-0.0739673937800244,-0.00507688280706297,
-0.864940598107329));
#41872=CARTESIAN_POINT('Ctrl Pts',(-0.0712186382622782,-0.0345785889264521,
-0.862392155363349));
#41873=CARTESIAN_POINT('Ctrl Pts',(-0.0315720180248721,-0.081431050040796,
-0.857727415837822));
#41874=CARTESIAN_POINT('Ctrl Pts',(0.0512714030294883,-0.0707039706402494,
-0.851378525493174));
#41875=CARTESIAN_POINT('Ctrl Pts',(0.0872105100082235,0.00470480361067377,
-0.845029635148532));
#41876=CARTESIAN_POINT('Ctrl Pts',(0.0433673424553154,0.0758095102297389,
-0.838680744803884));
#41877=CARTESIAN_POINT('Ctrl Pts',(-0.040149314234986,0.0775618514436692,
-0.832331854459241));
#41878=CARTESIAN_POINT('Ctrl Pts',(-0.0728396843020035,0.0292093066790861,
-0.827895854214532));
#41879=CARTESIAN_POINT('Ctrl Pts',(-0.0740086070644259,0.0023932392242425,
-0.825576150751372));
#41880=CARTESIAN_POINT('Ctrl Pts',(-0.0739930868845781,4.04624909366076E-5,
-0.825372744069761));
#41881=CARTESIAN_POINT('Origin',(0.,0.,-1.25327725593024));
#41882=CARTESIAN_POINT('',(-0.07393952028251,6.24297301232157E-5,-0.913277255930239));
#41883=CARTESIAN_POINT('',(-0.073778853988547,1.82460500730459E-6,-0.905372744069761));
#41884=CARTESIAN_POINT('',(-0.0739,1.16448635408261E-14,-1.25327725593024));
#41885=CARTESIAN_POINT('Ctrl Pts',(-0.07393952028251,6.24297301232151E-5,
-0.913277255930239));
#41886=CARTESIAN_POINT('Ctrl Pts',(-0.0737582361283602,-0.0200636709074026,
-0.911540559587986));
#41887=CARTESIAN_POINT('Ctrl Pts',(-0.0548509230184253,-0.0650146852071005,
-0.907687566464185));
#41888=CARTESIAN_POINT('Ctrl Pts',(0.0211743841364114,-0.0847316583180511,
-0.901718276558834));
#41889=CARTESIAN_POINT('Ctrl Pts',(0.0826634734150078,-0.0281879163445984,
-0.89536938621419));
#41890=CARTESIAN_POINT('Ctrl Pts',(0.0685300267273087,0.0541428102488016,
-0.889020495869544));
#41891=CARTESIAN_POINT('Ctrl Pts',(-0.00829633857195642,0.0869423903006062,
-0.882671605524899));
#41892=CARTESIAN_POINT('Ctrl Pts',(-0.0655246901945275,0.0483110572051783,
-0.877423858878463));
#41893=CARTESIAN_POINT('Ctrl Pts',(-0.0737913782812458,0.011837272014451,
-0.874292409013577));
#41894=CARTESIAN_POINT('Ctrl Pts',(-0.0737796652821541,8.1941925711617E-6,
-0.873277255930239));
#41895=CARTESIAN_POINT('Ctrl Pts',(-0.0737788771442885,1.82425625390881E-6,
-0.905372744069761));
#41896=CARTESIAN_POINT('Ctrl Pts',(-0.0737761361603925,-0.0124398715006289,
-0.904305045463286));
#41897=CARTESIAN_POINT('Ctrl Pts',(-0.0648908980282674,-0.0495460619161376,
-0.901121050075263));
#41898=CARTESIAN_POINT('Ctrl Pts',(-0.00614119170986879,-0.0871211455233005,
-0.895820757905693));
#41899=CARTESIAN_POINT('Ctrl Pts',(0.0698495376741126,-0.0524294794902851,
-0.889471867561047));
#41900=CARTESIAN_POINT('Ctrl Pts',(0.0819402280593655,0.0302259368504705,
-0.883122977216402));
#41901=CARTESIAN_POINT('Ctrl Pts',(0.0190700247449796,0.0852299383382114,
-0.876774086871756));
#41902=CARTESIAN_POINT('Ctrl Pts',(-0.0557790826493524,0.0638267794753937,
-0.870857342489544));
#41903=CARTESIAN_POINT('Ctrl Pts',(-0.0737414368455285,0.0194639290651083,
-0.867056894888878));
#41904=CARTESIAN_POINT('Ctrl Pts',(-0.0739212535704956,-6.56703637913767E-5,
-0.865372744069761));
#41905=CARTESIAN_POINT('Origin',(0.,0.,-1.25327725593024));
#41906=CARTESIAN_POINT('',(-0.0739789826382999,-4.8665297793311E-5,-0.953277255930239));
#41907=CARTESIAN_POINT('',(-0.0739279435619739,6.46796249051864E-5,-0.94537274406976));
#41908=CARTESIAN_POINT('',(-0.0739,1.16448635408261E-14,-1.25327725593024));
#41909=CARTESIAN_POINT('Ctrl Pts',(-0.0739789826382999,-4.86652977933102E-5,
-0.953277255930239));
#41910=CARTESIAN_POINT('Ctrl Pts',(-0.0740015361495537,-0.00301071199880904,
-0.953021303725492));
#41911=CARTESIAN_POINT('Ctrl Pts',(-0.0724954516939983,-0.0304408031514225,
-0.950649054739196));
#41912=CARTESIAN_POINT('Ctrl Pts',(-0.0382166559382933,-0.0785321314734518,
-0.946160508971351));
#41913=CARTESIAN_POINT('Ctrl Pts',(0.0452310138244137,-0.0747125414725162,
-0.939811618626707));
#41914=CARTESIAN_POINT('Ctrl Pts',(0.087300263005714,-0.00254411949997818,
-0.933462728282061));
#41915=CARTESIAN_POINT('Ctrl Pts',(0.0495051294517987,0.0719517242520363,
-0.927113837937416));
#41916=CARTESIAN_POINT('Ctrl Pts',(-0.0335784885779334,0.0806243981044391,
-0.920764947592771));
#41917=CARTESIAN_POINT('Ctrl Pts',(-0.0716195454802255,0.0333433502862432,
-0.916152753590378));
#41918=CARTESIAN_POINT('Ctrl Pts',(-0.0739791446790601,0.00446151577495216,
-0.913656856369534));
#41919=CARTESIAN_POINT('Ctrl Pts',(-0.07393952028251,6.24297301232151E-5,
-0.913277255930239));
#41920=CARTESIAN_POINT('Ctrl Pts',(-0.0739279435619739,6.4679624905186E-5,
-0.94537274406976));
#41921=CARTESIAN_POINT('Ctrl Pts',(-0.0737470642738756,-0.019681810576853,
-0.943669492819243));
#41922=CARTESIAN_POINT('Ctrl Pts',(-0.0554445745886888,-0.0642593312559459,
-0.939849944787179));
#41923=CARTESIAN_POINT('Ctrl Pts',(0.0198363851821647,-0.085054841460156,
-0.933914099973564));
#41924=CARTESIAN_POINT('Ctrl Pts',(0.0822089648049221,-0.0294871893983564,
-0.927565209628919));
#41925=CARTESIAN_POINT('Ctrl Pts',(0.0693748038821494,0.0530560535586862,
-0.921216319284275));
#41926=CARTESIAN_POINT('Ctrl Pts',(-0.00692509813514159,0.0870623411626859,
-0.914867428939627));
#41927=CARTESIAN_POINT('Ctrl Pts',(-0.0651237345087083,0.0490972963047915,
-0.909586237201459));
#41928=CARTESIAN_POINT('Ctrl Pts',(-0.0737815690937712,0.0122209461942086,
-0.906421342244835));
#41929=CARTESIAN_POINT('Ctrl Pts',(-0.0737788771442885,1.82425625390881E-6,
-0.905372744069761));
#41930=CARTESIAN_POINT('Origin',(0.,0.,-1.25327725593024));
#41931=CARTESIAN_POINT('',(-0.0737911150624599,-3.07014270853876E-5,-0.993277255930239));
#41932=CARTESIAN_POINT('',(-0.0739882011667107,-4.35894684875718E-5,-0.985372744069761));
#41933=CARTESIAN_POINT('',(-0.0739,1.16448635408261E-14,-1.25327725593024));
#41934=CARTESIAN_POINT('Ctrl Pts',(-0.0737911150624599,-3.07014270853837E-5,
-0.993277255930239));
#41935=CARTESIAN_POINT('Ctrl Pts',(-0.07382999686459,-0.0104149423206292,
-0.992385751081449));
#41936=CARTESIAN_POINT('Ctrl Pts',(-0.0669337505610335,-0.0454004637637484,
-0.989377949451111));
#41937=CARTESIAN_POINT('Ctrl Pts',(-0.0133453396325877,-0.0863117047392357,
-0.984253851039223));
#41938=CARTESIAN_POINT('Ctrl Pts',(0.0652607242893321,-0.0580417636628946,
-0.977904960694579));
#41939=CARTESIAN_POINT('Ctrl Pts',(0.0841647062166166,0.0233261804187959,
-0.971556070349931));
#41940=CARTESIAN_POINT('Ctrl Pts',(0.0260727882493475,0.0833547729751633,
-0.965207180005289));
#41941=CARTESIAN_POINT('Ctrl Pts',(-0.0525676172963071,0.0677825693615826,
-0.959114241865388));
#41942=CARTESIAN_POINT('Ctrl Pts',(-0.0738150563209228,0.0214804616808422,
-0.95513760050704));
#41943=CARTESIAN_POINT('Ctrl Pts',(-0.0739789826382999,-4.86652977933102E-5,
-0.953277255930239));
#41944=CARTESIAN_POINT('Ctrl Pts',(-0.0739882011667107,-4.35894684875739E-5,
-0.985372744069761));
#41945=CARTESIAN_POINT('Ctrl Pts',(-0.0740062132812438,-0.00261774564105659,
-0.985150236956749));
#41946=CARTESIAN_POINT('Ctrl Pts',(-0.0727164539171304,-0.0296568149264066,
-0.982811433062189));
#41947=CARTESIAN_POINT('Ctrl Pts',(-0.0394495734597775,-0.077920083333527,
-0.978356332386082));
#41948=CARTESIAN_POINT('Ctrl Pts',(0.0440479277989371,-0.075416100995714,
-0.972007442041435));
#41949=CARTESIAN_POINT('Ctrl Pts',(0.0872493240631923,-0.00391965349424783,
-0.965658551696792));
#41950=CARTESIAN_POINT('Ctrl Pts',(0.0506329377619281,0.0711625874072329,
-0.959309661352143));
#41951=CARTESIAN_POINT('Ctrl Pts',(-0.032303679213407,0.0811435797963708,
-0.952960771007503));
#41952=CARTESIAN_POINT('Ctrl Pts',(-0.0713663810806487,0.0341294648344994,
-0.948315131913371));
#41953=CARTESIAN_POINT('Ctrl Pts',(-0.073971807543628,0.00485328584428242,
-0.945785789600792));
#41954=CARTESIAN_POINT('Ctrl Pts',(-0.0739279435619739,6.4679624905186E-5,
-0.94537274406976));
#41955=CARTESIAN_POINT('Origin',(0.,0.,-1.25327725593024));
#41956=CARTESIAN_POINT('',(-0.073866824948156,6.56932150246621E-5,-1.03327725593024));
#41957=CARTESIAN_POINT('',(-0.0737964283105518,-3.62685935665213E-5,-1.02537274406976));
#41958=CARTESIAN_POINT('',(-0.0739,1.16448635408261E-14,-1.25327725593024));
#41959=CARTESIAN_POINT('Ctrl Pts',(-0.073866824948156,6.56932150246616E-5,
-1.03327725593024));
#41960=CARTESIAN_POINT('Ctrl Pts',(-0.0737142120031003,-0.0176755814077243,
-1.03175019843741));
#41961=CARTESIAN_POINT('Ctrl Pts',(-0.058407180002613,-0.0602401901634181,
-1.02810684416302));
#41962=CARTESIAN_POINT('Ctrl Pts',(0.0127141134428745,-0.0864069431030045,
-1.0223471931071));
#41963=CARTESIAN_POINT('Ctrl Pts',(0.0794802692010834,-0.0362035249468621,
-1.01599830276245));
#41964=CARTESIAN_POINT('Ctrl Pts',(0.0735359619677752,0.0471197494086118,
-1.0096494124178));
#41965=CARTESIAN_POINT('Ctrl Pts',(0.000319185439644519,0.0873367424855461,
-1.00330052207316));
#41966=CARTESIAN_POINT('Ctrl Pts',(-0.0628675604855332,0.0532279134888255,
-0.997843136577303));
#41967=CARTESIAN_POINT('Ctrl Pts',(-0.0737376973859944,0.0142356645848239,
-0.994502047862997));
#41968=CARTESIAN_POINT('Ctrl Pts',(-0.0737911150624599,-3.07014270853837E-5,
-0.993277255930239));
#41969=CARTESIAN_POINT('Ctrl Pts',(-0.0737964283105518,-3.62685935665187E-5,
-1.02537274406976));
#41970=CARTESIAN_POINT('Ctrl Pts',(-0.073840823994672,-0.0100291409910542,
-1.02451468431271));
#41971=CARTESIAN_POINT('Ctrl Pts',(-0.0672954261095734,-0.0446124579298668,
-1.0215403277741));
#41972=CARTESIAN_POINT('Ctrl Pts',(-0.0147039522670727,-0.0860906616485553,
-1.01644967445395));
#41973=CARTESIAN_POINT('Ctrl Pts',(0.0643378813590148,-0.0590630616174244,
-1.01010078410931));
#41974=CARTESIAN_POINT('Ctrl Pts',(0.0845218720571315,0.0219968493309595,
-1.00375189376466));
#41975=CARTESIAN_POINT('Ctrl Pts',(0.0273832188795813,0.0829335128685668,
-0.997403003420017));
#41976=CARTESIAN_POINT('Ctrl Pts',(-0.0519257991877054,0.0685239498085602,
-0.991276620188384));
#41977=CARTESIAN_POINT('Ctrl Pts',(-0.0738348974994724,0.0218654196361237,
-0.987266533738298));
#41978=CARTESIAN_POINT('Ctrl Pts',(-0.0739882011667107,-4.35894684875739E-5,
-0.985372744069761));
#41979=CARTESIAN_POINT('Origin',(0.,0.,-1.25327725593024));
#41980=CARTESIAN_POINT('',(-0.0740192616259655,-9.94807855793969E-6,-1.07327725593024));
#41981=CARTESIAN_POINT('',(-0.0738559566843222,6.38844806161408E-5,-1.06537274406976));
#41982=CARTESIAN_POINT('',(-0.0739,1.16448635408261E-14,-1.25327725593024));
#41983=CARTESIAN_POINT('Ctrl Pts',(-0.0740192616259655,-9.94807855795362E-6,
-1.07327725593024));
#41984=CARTESIAN_POINT('Ctrl Pts',(-0.074020272762249,-0.0005451446973743,
-1.07323094257491));
#41985=CARTESIAN_POINT('Ctrl Pts',(-0.0737726260818757,-0.0255352823793165,
-1.07106833243804));
#41986=CARTESIAN_POINT('Ctrl Pts',(-0.0457759481553394,-0.074379934125127,
-1.06678942551961));
#41987=CARTESIAN_POINT('Ctrl Pts',(0.037641655214997,-0.0788093717621258,
-1.06044053517497));
#41988=CARTESIAN_POINT('Ctrl Pts',(0.0866236680057719,-0.0111420824567537,
-1.05409164483032));
#41989=CARTESIAN_POINT('Ctrl Pts',(0.0563603151316931,0.0667182437528911,
-1.04774275448568));
#41990=CARTESIAN_POINT('Ctrl Pts',(-0.0254628383918398,0.0835431184830735,
-1.04139386414103));
#41991=CARTESIAN_POINT('Ctrl Pts',(-0.0699143291817533,0.0382765099988127,
-1.03657203128922));
#41992=CARTESIAN_POINT('Ctrl Pts',(-0.0739257130670484,0.0069114446609779,
-1.03386649521896));
#41993=CARTESIAN_POINT('Ctrl Pts',(-0.073866824948156,6.56932150246616E-5,
-1.03327725593024));
#41994=CARTESIAN_POINT('Ctrl Pts',(-0.0738559566843223,6.38844806161391E-5,
-1.06537274406976));
#41995=CARTESIAN_POINT('Ctrl Pts',(-0.0737124056741182,-0.0172952975271126,
-1.06387913166866));
#41996=CARTESIAN_POINT('Ctrl Pts',(-0.0589387738984228,-0.0594706446064186,
-1.06026922248602));
#41997=CARTESIAN_POINT('Ctrl Pts',(0.0113507662365832,-0.0865965857232952,
-1.05454301652183));
#41998=CARTESIAN_POINT('Ctrl Pts',(0.0788998284283993,-0.0374516345044027,
-1.04819412617718));
#41999=CARTESIAN_POINT('Ctrl Pts',(0.0742694349891011,0.045954971304813,
-1.04184523583253));
#42000=CARTESIAN_POINT('Ctrl Pts',(0.00169557022275755,0.087320864097371,
-1.03549634548789));
#42001=CARTESIAN_POINT('Ctrl Pts',(-0.062411361346758,0.0540091890348234,
-1.0300055149003));
#42002=CARTESIAN_POINT('Ctrl Pts',(-0.0737313276074497,0.0146170255717787,
-1.02663098109426));
#42003=CARTESIAN_POINT('Ctrl Pts',(-0.0737964283105518,-3.62685935665187E-5,
-1.02537274406976));
#42004=CARTESIAN_POINT('Origin',(0.,0.,-1.25327725593024));
#42005=CARTESIAN_POINT('',(-0.0738384445906279,-5.9163082798582E-5,-1.11327725593024));
#42006=CARTESIAN_POINT('',(-0.0740206415646085,-2.83210792082628E-6,-1.10537274406976));
#42007=CARTESIAN_POINT('',(-0.0739,1.16448635408261E-14,-1.25327725593024));
#42008=CARTESIAN_POINT('Ctrl Pts',(-0.0738384445906279,-5.91630827985745E-5,
-1.11327725593024));
#42009=CARTESIAN_POINT('Ctrl Pts',(-0.0738974492120266,-0.0079890193914202,
-1.11259538993087));
#42010=CARTESIAN_POINT('Ctrl Pts',(-0.0690655000923834,-0.0404598186853639,
-1.10979722714995));
#42011=CARTESIAN_POINT('Ctrl Pts',(-0.0217956051609413,-0.0845742251201784,
-1.10488276758748));
#42012=CARTESIAN_POINT('Ctrl Pts',(0.0592192057513427,-0.0641956017183869,
-1.09853387724284));
#42013=CARTESIAN_POINT('Ctrl Pts',(0.0860543001947688,0.0149114473055614,
-1.09218498689819));
#42014=CARTESIAN_POINT('Ctrl Pts',(0.0341672535616166,0.0803767533194929,
-1.08583609655355));
#42015=CARTESIAN_POINT('Ctrl Pts',(-0.048371565664984,0.0723705090856044,
-1.07953351956423));
#42016=CARTESIAN_POINT('Ctrl Pts',(-0.0739740687148976,0.0239107573613757,
-1.07534723935646));
#42017=CARTESIAN_POINT('Ctrl Pts',(-0.0740192616259655,-9.94807855795362E-6,
-1.07327725593024));
#42018=CARTESIAN_POINT('Ctrl Pts',(-0.0740206415646085,-2.8321079208263E-6,
-1.10537274406976));
#42019=CARTESIAN_POINT('Ctrl Pts',(-0.074020722247648,-0.000151529651826495,
-1.10535987580617));
#42020=CARTESIAN_POINT('Ctrl Pts',(-0.0739528370466597,-0.0247547414900179,
-1.10323071076103));
#42021=CARTESIAN_POINT('Ctrl Pts',(-0.0469427823151367,-0.0736491592978005,
-1.09898524893434));
#42022=CARTESIAN_POINT('Ctrl Pts',(0.0363951010157612,-0.07939287134855,
-1.09263635858969));
#42023=CARTESIAN_POINT('Ctrl Pts',(0.0864372276420334,-0.0125058552883607,
-1.08628746824505));
#42024=CARTESIAN_POINT('Ctrl Pts',(0.0574048355464994,0.0658217035478255,
-1.0799385779004));
#42025=CARTESIAN_POINT('Ctrl Pts',(-0.0241430608589063,0.0839340435518515,
-1.07358968755576));
#42026=CARTESIAN_POINT('Ctrl Pts',(-0.0696156377881968,0.0390645232381797,
-1.06873440961221));
#42027=CARTESIAN_POINT('Ctrl Pts',(-0.0739158028477489,0.00730089689808365,
-1.06599542845021));
#42028=CARTESIAN_POINT('Ctrl Pts',(-0.0738559566843223,6.38844806161391E-5,
-1.06537274406976));
#42029=CARTESIAN_POINT('Origin',(0.,0.,-1.25327725593024));
#42030=CARTESIAN_POINT('',(-0.0739,1.16448635408261E-14,-1.149325));
#42031=CARTESIAN_POINT('',(-0.0738510899558415,-6.10647340483564E-5,-1.14537274406976));
#42032=CARTESIAN_POINT('',(-0.0739,1.16448635408261E-14,-1.25327725593024));
#42033=CARTESIAN_POINT('',(-0.060110435027941,-0.0429877377952328,-1.149325));
#42034=CARTESIAN_POINT('Origin',(0.,0.,-1.149325));
#42035=CARTESIAN_POINT('Ctrl Pts',(-0.0601104350279426,-0.0429877377952305,
-1.149325));
#42036=CARTESIAN_POINT('Ctrl Pts',(-0.0458201451106566,-0.0629700766588213,
-1.14720870321845));
#42037=CARTESIAN_POINT('Ctrl Pts',(0.00400364749018219,-0.0872208216030551,
-1.14297610965536));
#42038=CARTESIAN_POINT('Ctrl Pts',(0.075583875527885,-0.0438759620050528,
-1.13662721931071));
#42039=CARTESIAN_POINT('Ctrl Pts',(0.0777927499997916,0.0396423987382078,
-1.13027832896607));
#42040=CARTESIAN_POINT('Ctrl Pts',(0.00894843417834478,0.0868766870214709,
-1.12392943862142));
#42041=CARTESIAN_POINT('Ctrl Pts',(-0.0598619431359153,0.0581055068125897,
-1.11826241427615));
#42042=CARTESIAN_POINT('Ctrl Pts',(-0.0737143174962966,0.0166227509558038,
-1.11471168671242));
#42043=CARTESIAN_POINT('Ctrl Pts',(-0.0738384445906279,-5.91630827985745E-5,
-1.11327725593024));
#42044=CARTESIAN_POINT('Ctrl Pts',(-0.0738510899558415,-6.10647340483625E-5,
-1.14537274406976));
#42045=CARTESIAN_POINT('Ctrl Pts',(-0.0739066365669056,-0.00760080692696395,
-1.14472432316213));
#42046=CARTESIAN_POINT('Ctrl Pts',(-0.0693607406337676,-0.0396777682903678,
-1.14195960547294));
#42047=CARTESIAN_POINT('Ctrl Pts',(-0.0231394877402551,-0.0842151856723098,
-1.13707859100221));
#42048=CARTESIAN_POINT('Ctrl Pts',(0.0582073462645349,-0.0651235753210661,
-1.13072970065757));
#42049=CARTESIAN_POINT('Ctrl Pts',(0.0862748105718152,0.0135547808574791,
-1.12438081031292));
#42050=CARTESIAN_POINT('Ctrl Pts',(0.0354317513839886,0.0798275566707828,
-1.11803191996827));
#42051=CARTESIAN_POINT('Ctrl Pts',(-0.0476646650497281,0.0730886637154228,
-1.11169589788723));
#42052=CARTESIAN_POINT('Ctrl Pts',(-0.0740074532268815,0.0243030621703926,
-1.10747617258772));
#42053=CARTESIAN_POINT('Ctrl Pts',(-0.0740206415646085,-2.8321079208263E-6,
-1.10537274406976));
#42054=CARTESIAN_POINT('Origin',(2.39206768658147E-17,-5.43753587379397E-18,
-0.013325));
#42055=CARTESIAN_POINT('',(-0.0452560140322605,0.0854280329804675,-0.013325));
#42056=CARTESIAN_POINT('Ctrl Pts',(0.0740200992814443,-0.000529165593927905,
-0.013325));
#42057=CARTESIAN_POINT('Ctrl Pts',(0.0743044627852839,0.00121921260606306,
-0.013325));
#42058=CARTESIAN_POINT('Ctrl Pts',(0.0745210416674805,0.00297514272191292,
-0.0133249999999998));
#42059=CARTESIAN_POINT('Ctrl Pts',(0.0746683292766584,0.00473514820652526,
-0.0133249999999998));
#42060=CARTESIAN_POINT('Ctrl Pts',(0.0750051149292103,0.00875955052345067,
-0.0133249999999999));
#42061=CARTESIAN_POINT('Ctrl Pts',(0.0749803322318632,0.0128050196487043,
-0.0133250000000001));
#42062=CARTESIAN_POINT('Ctrl Pts',(0.0746223571827205,0.0168365255250177,
-0.0133250000000001));
#42063=CARTESIAN_POINT('Ctrl Pts',(0.0743701515064359,0.0196768594209578,
-0.0133250000000001));
#42064=CARTESIAN_POINT('Ctrl Pts',(0.073951828239943,0.0225100795751238,
-0.0133250000000001));
#42065=CARTESIAN_POINT('Ctrl Pts',(0.0733791204930561,0.0253103719483463,
-0.0133250000000002));
#42066=CARTESIAN_POINT('Ctrl Pts',(0.0725805310638456,0.029215127733666,
-0.0133250000000003));
#42067=CARTESIAN_POINT('Ctrl Pts',(0.0714817005281231,0.0330626442864868,
-0.0133250000000001));
#42068=CARTESIAN_POINT('Ctrl Pts',(0.0701052438006905,0.0368218413152237,
-0.013325));
#42069=CARTESIAN_POINT('Ctrl Pts',(0.0691330418171139,0.0394769911177245,
-0.0133249999999999));
#42070=CARTESIAN_POINT('Ctrl Pts',(0.068021277102673,0.0420888634409962,
-0.0133249999999998));
#42071=CARTESIAN_POINT('Ctrl Pts',(0.0667846606791258,0.0446313284838127,
-0.0133249999999998));
#42072=CARTESIAN_POINT('Ctrl Pts',(0.063828770169334,0.0507085955720025,
-0.013325));
#42073=CARTESIAN_POINT('Ctrl Pts',(0.0601564831066114,0.0564106861323656,
-0.013325));
#42074=CARTESIAN_POINT('Ctrl Pts',(0.0558589764451619,0.061596620111266,
-0.0133249999999998));
#42075=CARTESIAN_POINT('Ctrl Pts',(0.054311387560419,0.0634641434020967,
-0.0133249999999997));
#42076=CARTESIAN_POINT('Ctrl Pts',(0.0526804759702182,0.06526640368048,
-0.0133249999999999));
#42077=CARTESIAN_POINT('Ctrl Pts',(0.0509747383512297,0.066990486897638,
-0.0133249999999999));
#42078=CARTESIAN_POINT('Ctrl Pts',(0.048133402035997,0.0698623824347133,
-0.0133249999999999));
#42079=CARTESIAN_POINT('Ctrl Pts',(0.0450946231233207,0.0725083069172221,
-0.0133250000000003));
#42080=CARTESIAN_POINT('Ctrl Pts',(0.0418777543778179,0.074900292157355,
-0.0133250000000002));
#42081=CARTESIAN_POINT('Ctrl Pts',(0.0376846139865073,0.0780182092125168,
-0.0133250000000001));
#42082=CARTESIAN_POINT('Ctrl Pts',(0.0331893030001897,0.0807054966328726,
-0.0133249999999999));
#42083=CARTESIAN_POINT('Ctrl Pts',(0.0284599480374241,0.0829678801923137,
-0.0133249999999997));
#42084=CARTESIAN_POINT('Ctrl Pts',(0.0255937901488642,0.0843389653692335,
-0.0133249999999996));
#42085=CARTESIAN_POINT('Ctrl Pts',(0.022637959968407,0.085554329703683,
-0.0133249999999998));
#42086=CARTESIAN_POINT('Ctrl Pts',(0.0196310938735226,0.0866056603112436,
-0.0133249999999998));
#42087=CARTESIAN_POINT('Ctrl Pts',(0.0144385045732225,0.0884212144103054,
-0.0133249999999999));
#42088=CARTESIAN_POINT('Ctrl Pts',(0.00908161914042202,0.0897557224136673,
-0.0133249999999999));
#42089=CARTESIAN_POINT('Ctrl Pts',(0.00363540148731718,0.0906157263666272,
-0.0133249999999999));
#42090=CARTESIAN_POINT('Ctrl Pts',(-0.000357205864503874,0.0912461929259696,
-0.0133249999999998));
#42091=CARTESIAN_POINT('Ctrl Pts',(-0.00439819318417859,0.0916213813352182,
-0.0133250000000001));
#42092=CARTESIAN_POINT('Ctrl Pts',(-0.00846098990337325,0.0917385588593169,
-0.013325));
#42093=CARTESIAN_POINT('Ctrl Pts',(-0.0113225184174696,0.0918210898963328,
-0.013325));
#42094=CARTESIAN_POINT('Ctrl Pts',(-0.0141871645686146,0.0917750525558502,
-0.0133250000000003));
#42095=CARTESIAN_POINT('Ctrl Pts',(-0.0170374024637594,0.0916013767188937,
-0.0133250000000002));
#42096=CARTESIAN_POINT('Ctrl Pts',(-0.0245300683346267,0.0911448200860685,
-0.013325));
#42097=CARTESIAN_POINT('Ctrl Pts',(-0.0319391506798941,0.0898104051975574,
-0.0133250000000003));
#42098=CARTESIAN_POINT('Ctrl Pts',(-0.0390995076077797,0.0875866732068192,
-0.0133250000000004));
#42099=CARTESIAN_POINT('Ctrl Pts',(-0.0411738518072883,0.0869424615281688,
-0.0133250000000005));
#42100=CARTESIAN_POINT('Ctrl Pts',(-0.0432273660238442,0.086223285901193,
-0.013325));
#42101=CARTESIAN_POINT('Ctrl Pts',(-0.0452560140322605,0.0854280329804675,
-0.013325));
#42102=CARTESIAN_POINT('',(-0.096675,-1.1839272930757E-17,-0.013325));
#42103=CARTESIAN_POINT('Origin',(0.,0.,-0.013325));
#42104=CARTESIAN_POINT('',(-0.0953132884602481,0.016639320268274,-0.013325));
#42105=CARTESIAN_POINT('Origin',(0.,0.,-0.013325));
#42106=CARTESIAN_POINT('Ctrl Pts',(-0.0953948120465086,0.0166363274765932,
-0.013325));
#42107=CARTESIAN_POINT('Ctrl Pts',(-0.0955400881374255,0.0143581077064726,
-0.013325));
#42108=CARTESIAN_POINT('Ctrl Pts',(-0.0955985924312004,0.0120778234632231,
-0.0133249999999999));
#42109=CARTESIAN_POINT('Ctrl Pts',(-0.0955674386515142,0.00979904378813855,
-0.0133249999999999));
#42110=CARTESIAN_POINT('Ctrl Pts',(-0.0954981213062938,0.00472874544841861,
-0.013325));
#42111=CARTESIAN_POINT('Ctrl Pts',(-0.0949855510048348,-0.000334448640519777,
-0.0133250000000001));
#42112=CARTESIAN_POINT('Ctrl Pts',(-0.0940540581382921,-0.00534172392063533,
-0.0133250000000002));
#42113=CARTESIAN_POINT('Ctrl Pts',(-0.0934623572121308,-0.00852243472069274,
-0.0133250000000003));
#42114=CARTESIAN_POINT('Ctrl Pts',(-0.0927007925980538,-0.0116809531331341,
-0.0133250000000003));
#42115=CARTESIAN_POINT('Ctrl Pts',(-0.0917795646923028,-0.0147890698658072,
-0.0133250000000002));
#42116=CARTESIAN_POINT('Ctrl Pts',(-0.0902526281395622,-0.0199407777327483,
-0.0133250000000002));
#42117=CARTESIAN_POINT('Ctrl Pts',(-0.088286029031168,-0.0249651054813939,
-0.013325));
#42118=CARTESIAN_POINT('Ctrl Pts',(-0.0859055131334032,-0.029799907615255,
-0.013325));
#42119=CARTESIAN_POINT('Ctrl Pts',(-0.0846952816011176,-0.0322578748148248,
-0.013325));
#42120=CARTESIAN_POINT('Ctrl Pts',(-0.0833776616024067,-0.0346663040964685,
-0.0133250000000004));
#42121=CARTESIAN_POINT('Ctrl Pts',(-0.0819632215061403,-0.037004905631243,
-0.0133250000000004));
#42122=CARTESIAN_POINT('Ctrl Pts',(-0.0783562873120896,-0.0429685246380169,
-0.0133250000000003));
#42123=CARTESIAN_POINT('Ctrl Pts',(-0.0741117287112331,-0.0485023320358176,
-0.0133250000000002));
#42124=CARTESIAN_POINT('Ctrl Pts',(-0.0692831287782071,-0.0534603643174138,
-0.0133250000000004));
#42125=CARTESIAN_POINT('Ctrl Pts',(-0.0675298846535145,-0.0552606047780678,
-0.0133250000000004));
#42126=CARTESIAN_POINT('Ctrl Pts',(-0.0656994071220876,-0.0569845310122871,
-0.013325));
#42127=CARTESIAN_POINT('Ctrl Pts',(-0.0637936345292532,-0.0586235633435691,
-0.013325));
#42128=CARTESIAN_POINT('Ctrl Pts',(-0.0618569431530899,-0.0602891869301303,
-0.013325));
#42129=CARTESIAN_POINT('Ctrl Pts',(-0.0598492146310193,-0.0618612346315886,
-0.013325));
#42130=CARTESIAN_POINT('Ctrl Pts',(-0.0577760214915456,-0.0633304149469573,
-0.013325));
#42131=CARTESIAN_POINT('Ctrl Pts',(-0.0562706950449255,-0.0643971732443243,
-0.0133249999999999));
#42132=CARTESIAN_POINT('Ctrl Pts',(-0.0547304006007948,-0.0654100638618711,
-0.013325));
#42133=CARTESIAN_POINT('Ctrl Pts',(-0.053156133026322,-0.0663660545506018,
-0.013325));
#42134=CARTESIAN_POINT('Ctrl Pts',(-0.0496177962615322,-0.0685147470953649,
-0.013325));
#42135=CARTESIAN_POINT('Ctrl Pts',(-0.0459078250945438,-0.0703764577179876,
-0.0133249999999997));
#42136=CARTESIAN_POINT('Ctrl Pts',(-0.0420623737642596,-0.0719462705416227,
-0.0133249999999998));
#42137=CARTESIAN_POINT('Ctrl Pts',(-0.0395974908876075,-0.0729524995681232,
-0.0133249999999998));
#42138=CARTESIAN_POINT('Ctrl Pts',(-0.0370748935076417,-0.0738392450007706,
-0.0133249999999998));
#42139=CARTESIAN_POINT('Ctrl Pts',(-0.0345107759053943,-0.0746018375885252,
-0.0133249999999998));
#42140=CARTESIAN_POINT('Ctrl Pts',(-0.0281794651533031,-0.0764848286986382,
-0.0133249999999996));
#42141=CARTESIAN_POINT('Ctrl Pts',(-0.0216430486600933,-0.0776015958572515,
-0.0133249999999997));
#42142=CARTESIAN_POINT('Ctrl Pts',(-0.0150531338947347,-0.0779342001631726,
-0.0133249999999997));
#42143=CARTESIAN_POINT('Ctrl Pts',(-0.0120753298759454,-0.0780844950416504,
-0.0133249999999997));
#42144=CARTESIAN_POINT('Ctrl Pts',(-0.00908668828005284,-0.0780739840860596,
-0.0133249999999997));
#42145=CARTESIAN_POINT('Ctrl Pts',(-0.00610252359415805,-0.0778977331119931,
-0.0133249999999997));
#42146=CARTESIAN_POINT('Ctrl Pts',(-0.00399701693690746,-0.0777733775089,
-0.0133249999999997));
#42147=CARTESIAN_POINT('Ctrl Pts',(-0.0018959538125692,-0.0775663788512026,
-0.0133249999999997));
#42148=CARTESIAN_POINT('Ctrl Pts',(0.000186776601496543,-0.0772767405557303,
-0.0133249999999997));
#42149=CARTESIAN_POINT('Ctrl Pts',(0.00624411631421537,-0.076434366747944,
-0.0133249999999998));
#42150=CARTESIAN_POINT('Ctrl Pts',(0.0121700652423237,-0.0748949340523382,
-0.0133249999999999));
#42151=CARTESIAN_POINT('Ctrl Pts',(0.0178272270255753,-0.0726202066517544,
-0.0133250000000001));
#42152=CARTESIAN_POINT('Ctrl Pts',(0.0197042518379329,-0.0718654607321863,
-0.0133250000000002));
#42153=CARTESIAN_POINT('Ctrl Pts',(0.021551428218358,-0.0710294440312932,
-0.013325));
#42154=CARTESIAN_POINT('Ctrl Pts',(0.0233628051714112,-0.0701098376443897,
-0.013325));
#42155=CARTESIAN_POINT('Ctrl Pts',(0.0663714283216862,0.032496822960703,
-1.16247415238079));
#42156=CARTESIAN_POINT('Ctrl Pts',(0.0555686030204049,0.0545604858000743,
-1.16035785559925));
#42157=CARTESIAN_POINT('Ctrl Pts',(0.0104211156604289,0.0866885407409115,
-1.15612526203615));
#42158=CARTESIAN_POINT('Ctrl Pts',(-0.0673222376269667,0.0557291632982185,
-1.1497763716915));
#42159=CARTESIAN_POINT('Ctrl Pts',(-0.0832609374865553,-0.0262839541860632,
-1.14342748134686));
#42160=CARTESIAN_POINT('Ctrl Pts',(-0.0231394877402551,-0.0842151856723098,
-1.13707859100221));
#42161=CARTESIAN_POINT('Ctrl Pts',(0.0582073462645349,-0.0651235753210661,
-1.13072970065757));
#42162=CARTESIAN_POINT('Ctrl Pts',(0.0862748105718152,0.0135547808574791,
-1.12438081031292));
#42163=CARTESIAN_POINT('Ctrl Pts',(0.0354317513839886,0.0798275566707828,
-1.11803191996827));
#42164=CARTESIAN_POINT('Ctrl Pts',(-0.0478334312845205,0.0730749772336279,
-1.11168302962363));
#42165=CARTESIAN_POINT('Ctrl Pts',(-0.0873350606334346,-0.000529835700201266,
-1.10533413927899));
#42166=CARTESIAN_POINT('Ctrl Pts',(-0.0469427823151367,-0.0736491592978005,
-1.09898524893434));
#42167=CARTESIAN_POINT('Ctrl Pts',(0.0363951010157612,-0.07939287134855,
-1.09263635858969));
#42168=CARTESIAN_POINT('Ctrl Pts',(0.0864372276420334,-0.0125058552883607,
-1.08628746824505));
#42169=CARTESIAN_POINT('Ctrl Pts',(0.0574048355464994,0.0658217035478255,
-1.0799385779004));
#42170=CARTESIAN_POINT('Ctrl Pts',(-0.0241430608589063,0.0839340435518515,
-1.07358968755576));
#42171=CARTESIAN_POINT('Ctrl Pts',(-0.0836042097301358,0.0252614675221138,
-1.06724079721112));
#42172=CARTESIAN_POINT('Ctrl Pts',(-0.0665822640251934,-0.0565208904508504,
-1.06089190686647));
#42173=CARTESIAN_POINT('Ctrl Pts',(0.0113507662365832,-0.0865965857232952,
-1.05454301652183));
#42174=CARTESIAN_POINT('Ctrl Pts',(0.0788998284283993,-0.0374516345044027,
-1.04819412617718));
#42175=CARTESIAN_POINT('Ctrl Pts',(0.0742694349891011,0.045954971304813,
-1.04184523583253));
#42176=CARTESIAN_POINT('Ctrl Pts',(0.00169557022275755,0.087320864097371,
-1.03549634548789));
#42177=CARTESIAN_POINT('Ctrl Pts',(-0.0724294409889089,0.0488035270943797,
-1.02914745514324));
#42178=CARTESIAN_POINT('Ctrl Pts',(-0.0802942565935507,-0.034360451292179,
-1.0227985647986));
#42179=CARTESIAN_POINT('Ctrl Pts',(-0.0147039522670727,-0.0860906616485553,
-1.01644967445395));
#42180=CARTESIAN_POINT('Ctrl Pts',(0.0643378813590148,-0.0590630616174244,
-1.01010078410931));
#42181=CARTESIAN_POINT('Ctrl Pts',(0.0845218720571315,0.0219968493309595,
-1.00375189376466));
#42182=CARTESIAN_POINT('Ctrl Pts',(0.0273832188795813,0.0829335128685668,
-0.997403003420017));
#42183=CARTESIAN_POINT('Ctrl Pts',(-0.0548062622568154,0.0680006018306399,
-0.991054113075372));
#42184=CARTESIAN_POINT('Ctrl Pts',(-0.086857655002089,-0.00914089716737991,
-0.984705222730726));
#42185=CARTESIAN_POINT('Ctrl Pts',(-0.0394495734597775,-0.077920083333527,
-0.978356332386082));
#42186=CARTESIAN_POINT('Ctrl Pts',(0.0440479277989371,-0.075416100995714,
-0.972007442041435));
#42187=CARTESIAN_POINT('Ctrl Pts',(0.0872493240631923,-0.00391965349424783,
-0.965658551696792));
#42188=CARTESIAN_POINT('Ctrl Pts',(0.0506329377619281,0.0711625874072329,
-0.959309661352143));
#42189=CARTESIAN_POINT('Ctrl Pts',(-0.032303679213407,0.0811435797963708,
-0.952960771007503));
#42190=CARTESIAN_POINT('Ctrl Pts',(-0.0856881125918317,0.0168924714998301,
-0.946611880662853));
#42191=CARTESIAN_POINT('Ctrl Pts',(-0.0606829972532737,-0.0628122764852983,
-0.940262990318211));
#42192=CARTESIAN_POINT('Ctrl Pts',(0.0198363851821647,-0.085054841460156,
-0.933914099973564));
#42193=CARTESIAN_POINT('Ctrl Pts',(0.0822089648049221,-0.0294871893983564,
-0.927565209628919));
#42194=CARTESIAN_POINT('Ctrl Pts',(0.0693748038821494,0.0530560535586862,
-0.921216319284275));
#42195=CARTESIAN_POINT('Ctrl Pts',(-0.00692509813514159,0.0870623411626859,
-0.914867428939627));
#42196=CARTESIAN_POINT('Ctrl Pts',(-0.0768897536262579,0.0414219026627595,
-0.908518538594985));
#42197=CARTESIAN_POINT('Ctrl Pts',(-0.0765138110414937,-0.042112289807323,
-0.902169648250337));
#42198=CARTESIAN_POINT('Ctrl Pts',(-0.00614119170986879,-0.0871211455233005,
-0.895820757905693));
#42199=CARTESIAN_POINT('Ctrl Pts',(0.0698495376741126,-0.0524294794902851,
-0.889471867561047));
#42200=CARTESIAN_POINT('Ctrl Pts',(0.0819402280593655,0.0302259368504705,
-0.883122977216402));
#42201=CARTESIAN_POINT('Ctrl Pts',(0.0190700247449796,0.0852299383382114,
-0.876774086871756));
#42202=CARTESIAN_POINT('Ctrl Pts',(-0.061245896400729,0.0622635399489994,
-0.870425196527112));
#42203=CARTESIAN_POINT('Ctrl Pts',(-0.0855325967550582,-0.0176630440537883,
-0.864076306182466));
#42204=CARTESIAN_POINT('Ctrl Pts',(-0.0315720180248721,-0.081431050040796,
-0.857727415837822));
#42205=CARTESIAN_POINT('Ctrl Pts',(0.0512714030294883,-0.0707039706402494,
-0.851378525493174));
#42206=CARTESIAN_POINT('Ctrl Pts',(0.0872105100082235,0.00470480361067377,
-0.845029635148532));
#42207=CARTESIAN_POINT('Ctrl Pts',(0.0433673424553154,0.0758095102297389,
-0.838680744803884));
#42208=CARTESIAN_POINT('Ctrl Pts',(-0.040149314234986,0.0775618514436692,
-0.832331854459241));
#42209=CARTESIAN_POINT('Ctrl Pts',(-0.0869364114920166,0.00835874331464967,
-0.825982964114595));
#42210=CARTESIAN_POINT('Ctrl Pts',(-0.0541919861401563,-0.0684911444720746,
-0.819634073769949));
#42211=CARTESIAN_POINT('Ctrl Pts',(0.0281285730428364,-0.0826836840705789,
-0.813285183425303));
#42212=CARTESIAN_POINT('Ctrl Pts',(0.0847164362872849,-0.0212351985084165,
-0.80693629308066));
#42213=CARTESIAN_POINT('Ctrl Pts',(0.0638036636957854,0.0596397579799298,
-0.800587402736013));
#42214=CARTESIAN_POINT('Ctrl Pts',(-0.015478236798094,0.0859548277790816,
-0.794238512391369));
#42215=CARTESIAN_POINT('Ctrl Pts',(-0.0806002735625345,0.033636351385875,
-0.787889622046722));
#42216=CARTESIAN_POINT('Ctrl Pts',(-0.0719872392663277,-0.0494534691980449,
-0.781540731702079));
#42217=CARTESIAN_POINT('Ctrl Pts',(0.00248145491972144,-0.0873020653500868,
-0.775191841357431));
#42218=CARTESIAN_POINT('Ctrl Pts',(0.0746800543932818,-0.0452846299391521,
-0.768842951012788));
#42219=CARTESIAN_POINT('Ctrl Pts',(0.0785595418575094,0.0381602753665082,
-0.762494060668141));
#42220=CARTESIAN_POINT('Ctrl Pts',(0.0105708687644261,0.0866952418906293,
-0.756145170323498));
#42221=CARTESIAN_POINT('Ctrl Pts',(-0.0670882896144543,0.0559193135644258,
-0.749796279978851));
#42222=CARTESIAN_POINT('Ctrl Pts',(-0.0833734652087589,-0.0260129493136267,
-0.743447389634208));
#42223=CARTESIAN_POINT('Ctrl Pts',(-0.0233865872476794,-0.084147939783551,
-0.737098499289559));
#42224=CARTESIAN_POINT('Ctrl Pts',(0.0579949038623966,-0.0653023687081939,
-0.730749608944917));
#42225=CARTESIAN_POINT('Ctrl Pts',(0.0863212604370854,0.0132833817028017,
-0.724400718600269));
#42226=CARTESIAN_POINT('Ctrl Pts',(0.035678849400398,0.079717174676309,
-0.718051828255625));
#42227=CARTESIAN_POINT('Ctrl Pts',(-0.0476034321928007,0.0732237767147732,
-0.71170293791098));
#42228=CARTESIAN_POINT('Ctrl Pts',(-0.0873369477542859,-0.00025649536951448,
-0.705354047566334));
#42229=CARTESIAN_POINT('Ctrl Pts',(-0.047172520489486,-0.0735021193135168,
-0.699005157221689));
#42230=CARTESIAN_POINT('Ctrl Pts',(0.0361464644047429,-0.0795062346231174,
-0.692656266877045));
#42231=CARTESIAN_POINT('Ctrl Pts',(0.0863977932766005,-0.0127761320376415,
-0.686307376532398));
#42232=CARTESIAN_POINT('Ctrl Pts',(0.0576103404526291,0.065641883777369,
-0.679958486187753));
#42233=CARTESIAN_POINT('Ctrl Pts',(-0.0238804390394198,0.0840091236961439,
-0.673609595843108));
#42234=CARTESIAN_POINT('Ctrl Pts',(-0.0835248178717377,0.0255227943690046,
-0.667260705498462));
#42235=CARTESIAN_POINT('Ctrl Pts',(-0.0667586820880982,-0.0563124018202895,
-0.660911815153819));
#42236=CARTESIAN_POINT('Ctrl Pts',(0.011079903578258,-0.0866316568559436,
-0.654562924809171));
#42237=CARTESIAN_POINT('Ctrl Pts',(0.0787823266538737,-0.0376981861620926,
-0.648214034464528));
#42238=CARTESIAN_POINT('Ctrl Pts',(0.0744127802759426,0.0457224929822708,
-0.641865144119881));
#42239=CARTESIAN_POINT('Ctrl Pts',(0.00196863068701841,0.0873151345765873,
-0.635516253775237));
#42240=CARTESIAN_POINT('Ctrl Pts',(-0.0722764696578212,0.0490297885648256,
-0.62916736343059));
#42241=CARTESIAN_POINT('Ctrl Pts',(-0.0804013151861886,-0.0341091886335733,
-0.622818473085947));
#42242=CARTESIAN_POINT('Ctrl Pts',(-0.0149731015673857,-0.0860442587414302,
-0.6164695827413));
#42243=CARTESIAN_POINT('Ctrl Pts',(0.0641528659084539,-0.0592639690591287,
-0.610120692396656));
#42244=CARTESIAN_POINT('Ctrl Pts',(0.0845902468891876,0.0217324265588487,
-0.60377180205201));
#42245=CARTESIAN_POINT('Ctrl Pts',(0.027642433133917,0.0828474750571577,
-0.597422911707366));
#42246=CARTESIAN_POINT('Ctrl Pts',(-0.0545933440652645,0.0681716584562908,
-0.591074021362719));
#42247=CARTESIAN_POINT('Ctrl Pts',(-0.0868858155389696,-0.0088692328325284,
-0.584725131018075));
#42248=CARTESIAN_POINT('Ctrl Pts',(-0.0396930507999507,-0.0777963363604095,
-0.578376240673428));
#42249=CARTESIAN_POINT('Ctrl Pts',(0.0438118725954223,-0.0755534780972525,
-0.572027350328785));
#42250=CARTESIAN_POINT('Ctrl Pts',(0.0872366399772161,-0.00419247878885715,
-0.565678459984137));
#42251=CARTESIAN_POINT('Ctrl Pts',(0.0508552285025388,0.0710039010679274,
-0.559329569639494));
#42252=CARTESIAN_POINT('Ctrl Pts',(-0.0320497705692809,0.0812442024969535,
-0.552980679294847));
#42253=CARTESIAN_POINT('Ctrl Pts',(-0.0856348677853095,0.017160351170707,
-0.546631788950203));
#42254=CARTESIAN_POINT('Ctrl Pts',(-0.0608791259157248,-0.0626222026173367,
-0.540282898605557));
#42255=CARTESIAN_POINT('Ctrl Pts',(0.0195703062739464,-0.085116457546431,
-0.533934008260913));
#42256=CARTESIAN_POINT('Ctrl Pts',(0.0821163510431211,-0.0297441275594417,
-0.527585117916266));
#42257=CARTESIAN_POINT('Ctrl Pts',(0.0695403805661829,0.052838846539454,
-0.521236227571622));
#42258=CARTESIAN_POINT('Ctrl Pts',(-0.00665280454283421,0.0870835714967197,
-0.514887337226976));
#42259=CARTESIAN_POINT('Ctrl Pts',(-0.0767598438605726,0.0416621483292682,
-0.508538446882331));
#42260=CARTESIAN_POINT('Ctrl Pts',(-0.0766451296842338,-0.0418728113290297,
-0.502189556537686));
#42261=CARTESIAN_POINT('Ctrl Pts',(-0.00641360530457873,-0.0871015149116623,
-0.49584066619304));
#42262=CARTESIAN_POINT('Ctrl Pts',(0.0696852396434252,-0.0526476553015217,
-0.489491775848395));
#42263=CARTESIAN_POINT('Ctrl Pts',(0.0820343493873717,0.0299695471020194,
-0.48314288550375));
#42264=CARTESIAN_POINT('Ctrl Pts',(0.0193364609744337,0.0851698861681384,
-0.476793995159104));
#42265=CARTESIAN_POINT('Ctrl Pts',(-0.0610508875481533,0.0624547625285068,
-0.47044510481446));
#42266=CARTESIAN_POINT('Ctrl Pts',(-0.0855874140733924,-0.0173954817449568,
-0.464096214469814));
#42267=CARTESIAN_POINT('Ctrl Pts',(-0.0318265133113365,-0.0813319204454977,
-0.45774732412517));
#42268=CARTESIAN_POINT('Ctrl Pts',(0.0510500481910435,-0.070863959899244,
-0.451398433780523));
#42269=CARTESIAN_POINT('Ctrl Pts',(0.0872247963540974,0.00443205752395941,
-0.445049543435879));
#42270=CARTESIAN_POINT('Ctrl Pts',(0.0436042004922963,0.0756735220029905,
-0.438700653091233));
#42271=CARTESIAN_POINT('Ctrl Pts',(-0.0399065679425262,0.0776870263812308,
-0.432351762746588));
#42272=CARTESIAN_POINT('Ctrl Pts',(-0.0869098470976033,0.00863056836950265,
-0.426002872401942));
#42273=CARTESIAN_POINT('Ctrl Pts',(-0.054405905391453,-0.0683213414054914,
-0.419653982057298));
#42274=CARTESIAN_POINT('Ctrl Pts',(0.0278698686279614,-0.0827712429263309,
-0.413305091712652));
#42275=CARTESIAN_POINT('Ctrl Pts',(0.0846496157370046,-0.0215000183368973,
-0.406956201368007));
#42276=CARTESIAN_POINT('Ctrl Pts',(0.0639898560584943,0.0594399407345146,
-0.400607311023361));
#42277=CARTESIAN_POINT('Ctrl Pts',(-0.0152093647792003,0.0860028107443161,
-0.394258420678717));
#42278=CARTESIAN_POINT('Ctrl Pts',(-0.0804946924846155,0.0338882385897622,
-0.387909530334071));
#42279=CARTESIAN_POINT('Ctrl Pts',(-0.0721415372417917,-0.0492281102349125,
-0.381560639989426));
#42280=CARTESIAN_POINT('Ctrl Pts',(0.00220843339423072,-0.0873093984336892,
-0.375211749644781));
#42281=CARTESIAN_POINT('Ctrl Pts',(0.0745380759834756,-0.0455179465880336,
-0.368862859300135));
#42282=CARTESIAN_POINT('Ctrl Pts',(0.0786784918314324,0.0379144188408675,
-0.36251396895549));
#42283=CARTESIAN_POINT('Ctrl Pts',(0.0108419288216904,0.0866617609579614,
-0.356165078610845));
#42284=CARTESIAN_POINT('Ctrl Pts',(-0.0669130917411956,0.0561288373881358,
-0.349816188266199));
#42285=CARTESIAN_POINT('Ctrl Pts',(-0.0834544047526216,-0.0257520981726755,
-0.343467297921554));
#42286=CARTESIAN_POINT('Ctrl Pts',(-0.0236496187649619,-0.0840743942302376,
-0.337118407576909));
#42287=CARTESIAN_POINT('Ctrl Pts',(0.0577904079373426,-0.0654834099856214,
-0.330769517232263));
#42288=CARTESIAN_POINT('Ctrl Pts',(0.086362377900638,0.0130133745145877,
-0.324420626887618));
#42289=CARTESIAN_POINT('Ctrl Pts',(0.0359279650068146,0.0796052106546962,
-0.318071736542973));
#42290=CARTESIAN_POINT('Ctrl Pts',(-0.0473742153988214,0.073372283242758,
-0.311722846198328));
#42291=CARTESIAN_POINT('Ctrl Pts',(-0.0873373228152785,1.66243603213149E-5,
-0.305373955853682));
#42292=CARTESIAN_POINT('Ctrl Pts',(-0.0474021442906221,-0.073354242887242,
-0.299025065509037));
#42293=CARTESIAN_POINT('Ctrl Pts',(0.0358976572459432,-0.0796188824159332,
-0.292676175164391));
#42294=CARTESIAN_POINT('Ctrl Pts',(0.0863574175401337,-0.0130462511361909,
-0.286327284819747));
#42295=CARTESIAN_POINT('Ctrl Pts',(0.0578153328344367,0.0654614048287443,
-0.279978394475101));
#42296=CARTESIAN_POINT('Ctrl Pts',(-0.0236176105063063,0.0840833913854678,
-0.273629504130456));
#42297=CARTESIAN_POINT('Ctrl Pts',(-0.083444595058164,0.0257838668257644,
-0.267280613785811));
#42298=CARTESIAN_POINT('Ctrl Pts',(-0.0669344547556335,-0.0561033599660063,
-0.260931723441166));
#42299=CARTESIAN_POINT('Ctrl Pts',(0.0108089364983639,-0.086665882126032,
-0.25458283309652));
#42300=CARTESIAN_POINT('Ctrl Pts',(0.0786640523710499,-0.0379443684553606,
-0.248233942751875));
#42301=CARTESIAN_POINT('Ctrl Pts',(0.0745553989520529,0.045489567155642,
-0.24188505240723));
#42302=CARTESIAN_POINT('Ctrl Pts',(0.00224167132305463,0.087308551371477,
-0.235536162062585));
#42303=CARTESIAN_POINT('Ctrl Pts',(-0.0721227912104874,0.0492555704558522,
-0.229187271717939));
#42304=CARTESIAN_POINT('Ctrl Pts',(-0.0805075876714163,-0.0338575923571341,
-0.222838381373294));
#42305=CARTESIAN_POINT('Ctrl Pts',(-0.015242104357177,-0.0859970144113175,
-0.216489491028649));
#42306=CARTESIAN_POINT('Ctrl Pts',(0.0639672230445058,-0.0594642969265874,
-0.210140600684003));
#42307=CARTESIAN_POINT('Ctrl Pts',(0.0846577945115181,0.0214677912515853,
-0.203791710339358));
#42308=CARTESIAN_POINT('Ctrl Pts',(0.0279013770542819,0.0827606270598339,
-0.197442819994713));
#42309=CARTESIAN_POINT('Ctrl Pts',(-0.0543798919864373,0.0683420484111352,
-0.191093929650068));
#42310=CARTESIAN_POINT('Ctrl Pts',(-0.0869131263917905,-0.00859748176483909,
-0.184745039305422));
#42311=CARTESIAN_POINT('Ctrl Pts',(-0.0399361399802455,-0.0776718285893026,
-0.178396148960777));
#42312=CARTESIAN_POINT('Ctrl Pts',(0.0435753889642203,-0.0756901163504716,
-0.172047258616132));
#42313=CARTESIAN_POINT('Ctrl Pts',(0.0872231027375695,-0.00446526306300281,
-0.165698368271486));
#42314=CARTESIAN_POINT('Ctrl Pts',(0.0510770219946841,0.0708445203210023,
-0.159349477926841));
#42315=CARTESIAN_POINT('Ctrl Pts',(-0.031795548652228,0.0813440307632768,
-0.153000587582196));
#42316=CARTESIAN_POINT('Ctrl Pts',(-0.0855807852442883,0.0174280628811339,
-0.146651697237551));
#42317=CARTESIAN_POINT('Ctrl Pts',(-0.0610746597672231,-0.0624315160748942,
-0.140302806892905));
#42318=CARTESIAN_POINT('Ctrl Pts',(0.019304037012885,-0.0851772417740305,
-0.13395391654826));
#42319=CARTESIAN_POINT('Ctrl Pts',(0.0820229322870143,-0.03000077385872,
-0.127605026203615));
#42320=CARTESIAN_POINT('Ctrl Pts',(0.0697052809023569,0.0526211209250912,
-0.12125613585897));
#42321=CARTESIAN_POINT('Ctrl Pts',(-0.00638045292204925,0.0871039537597873,
-0.114907245514324));
#42322=CARTESIAN_POINT('Ctrl Pts',(-0.0766291701037609,0.0419019798479763,
-0.108558355169679));
#42323=CARTESIAN_POINT('Ctrl Pts',(-0.0767757240810127,-0.0416329106169278,
-0.102209464825034));
#42324=CARTESIAN_POINT('Ctrl Pts',(-0.00668590821907806,-0.0870810566848186,
-0.0958605744803883));
#42325=CARTESIAN_POINT('Ctrl Pts',(0.0695201691859918,-0.0528652704077562,
-0.0895116841357433));
#42326=CARTESIAN_POINT('Ctrl Pts',(0.0821278409720519,0.0297127773219571,
-0.0831627937910981));
#42327=CARTESIAN_POINT('Ctrl Pts',(0.0196023809749374,0.0851091659979851,
-0.0768139034464528));
#42328=CARTESIAN_POINT('Ctrl Pts',(-0.0608546612607467,0.0626450616134637,
-0.0704650131018075));
#42329=CARTESIAN_POINT('Ctrl Pts',(-0.0856425709892414,-0.0171271562291846,
-0.0641161227571622));
#42330=CARTESIAN_POINT('Ctrl Pts',(-0.0320784659707213,-0.081233120284334,
-0.0577672324125169));
#42331=CARTESIAN_POINT('Ctrl Pts',(0.0508239621622661,-0.0710211228679567,
-0.0514183420678718));
#42332=CARTESIAN_POINT('Ctrl Pts',(0.0872462569835861,0.00415522130723803,
-0.0450694517232264));
#42333=CARTESIAN_POINT('Ctrl Pts',(0.0438253963339189,0.0755444771434547,
-0.0387205613785811));
#42334=CARTESIAN_POINT('Ctrl Pts',(-0.0396344344718481,0.0777967966107338,
-0.0323716710339359));
#42335=CARTESIAN_POINT('Ctrl Pts',(-0.0869382878310626,0.00893070154157359,
-0.0260227806892905));
#42336=CARTESIAN_POINT('Ctrl Pts',(-0.0545061222546148,-0.0682098628070873,
-0.0196738903446452));
#42337=CARTESIAN_POINT('Ctrl Pts',(5.63936834513772E-5,-0.0778762677080245,
-0.0154412967815484));
#42338=CARTESIAN_POINT('Ctrl Pts',(0.0233628051714112,-0.0701098376443897,
-0.013325));
#42339=CARTESIAN_POINT('Ctrl Pts',(0.0731896930038075,0.0358351862576369,
-1.1580911015872));
#42340=CARTESIAN_POINT('Ctrl Pts',(0.0612771052025858,0.0601654251960909,
-1.15597480480565));
#42341=CARTESIAN_POINT('Ctrl Pts',(0.0114916655439019,0.0955939602960504,
-1.15174221124255));
#42342=CARTESIAN_POINT('Ctrl Pts',(-0.0742381779154394,0.0614541596632013,
-1.14539332089791));
#42343=CARTESIAN_POINT('Ctrl Pts',(-0.0918142430853653,-0.0289840762275061,
-1.13904443055326));
#42344=CARTESIAN_POINT('Ctrl Pts',(-0.0255165821619241,-0.0928665201499235,
-1.13269554020862));
#42345=CARTESIAN_POINT('Ctrl Pts',(0.0641869236717294,-0.0718136494209175,
-1.12634664986397));
#42346=CARTESIAN_POINT('Ctrl Pts',(0.0951377280764297,0.0149472487601828,
-1.11999775951933));
#42347=CARTESIAN_POINT('Ctrl Pts',(0.0390716166874169,0.0880281547906619,
-1.11364886917468));
#42348=CARTESIAN_POINT('Ctrl Pts',(-0.05274730768283,0.0805818902083492,
-1.10729997883004));
#42349=CARTESIAN_POINT('Ctrl Pts',(-0.0963068964743298,-0.000584265145724099,
-1.10095108848539));
#42350=CARTESIAN_POINT('Ctrl Pts',(-0.051765163313003,-0.0812150573718085,
-1.09460219814075));
#42351=CARTESIAN_POINT('Ctrl Pts',(0.0401339301796505,-0.0875488147178018,
-1.0882533077961));
#42352=CARTESIAN_POINT('Ctrl Pts',(0.0953168300757157,-0.0137905682075853,
-1.08190441745145));
#42353=CARTESIAN_POINT('Ctrl Pts',(0.063301971900001,0.0725834956015103,
-1.07555552710681));
#42354=CARTESIAN_POINT('Ctrl Pts',(-0.0266232512561183,0.0925564966050465,
-1.06920663676216));
#42355=CARTESIAN_POINT('Ctrl Pts',(-0.092192779313374,0.0278565506200653,
-1.06285774641752));
#42356=CARTESIAN_POINT('Ctrl Pts',(-0.0734221876299457,-0.0623272200855746,
-1.05650885607287));
#42357=CARTESIAN_POINT('Ctrl Pts',(0.0125168181131665,-0.0954925588394342,
-1.05015996572822));
#42358=CARTESIAN_POINT('Ctrl Pts',(0.0870051220344295,-0.041299000205068,
-1.04381107538358));
#42359=CARTESIAN_POINT('Ctrl Pts',(0.0818990533106015,0.0506758755513958,
-1.03746218503893));
#42360=CARTESIAN_POINT('Ctrl Pts',(0.00186975430856264,0.0962912415435487,
-1.03111329469429));
#42361=CARTESIAN_POINT('Ctrl Pts',(-0.0798700387269449,0.0538170603806867,
-1.02476440434965));
#42362=CARTESIAN_POINT('Ctrl Pts',(-0.0885427982891663,-0.03789026310174,
-1.018415514005));
#42363=CARTESIAN_POINT('Ctrl Pts',(-0.0162144732994691,-0.0949346617344636,
-1.01206662366035));
#42364=CARTESIAN_POINT('Ctrl Pts',(0.0709472419722389,-0.06513054573261,
-1.00571773331571));
#42365=CARTESIAN_POINT('Ctrl Pts',(0.0932047120936722,0.0242565617509546,
-0.999368842971063));
#42366=CARTESIAN_POINT('Ctrl Pts',(0.030196267188026,0.0914531824923003,
-0.993019952626421));
#42367=CARTESIAN_POINT('Ctrl Pts',(-0.060436450001061,0.0749862297363351,
-0.986671062281772));
#42368=CARTESIAN_POINT('Ctrl Pts',(-0.0957804474814418,-0.0100799315967322,
-0.98032217193713));
#42369=CARTESIAN_POINT('Ctrl Pts',(-0.0435021852574599,-0.0859247287909974,
-0.973973281592482));
#42370=CARTESIAN_POINT('Ctrl Pts',(0.0485729235392217,-0.0831635150695851,
-0.967624391247839));
#42371=CARTESIAN_POINT('Ctrl Pts',(0.0962123522794268,-0.00432231523683321,
-0.961275500903193));
#42372=CARTESIAN_POINT('Ctrl Pts',(0.0558344044174431,0.0784730426539623,
-0.954926610558547));
#42373=CARTESIAN_POINT('Ctrl Pts',(-0.0356222010631393,0.0894793715413515,
-0.948577720213903));
#42374=CARTESIAN_POINT('Ctrl Pts',(-0.0944907592507357,0.0186278167339679,
-0.942228829869257));
#42375=CARTESIAN_POINT('Ctrl Pts',(-0.0669168955953715,-0.0692649133682613,
-0.935879939524612));
#42376=CARTESIAN_POINT('Ctrl Pts',(0.0218741554686966,-0.0937924328641027,
-0.929531049179966));
#42377=CARTESIAN_POINT('Ctrl Pts',(0.0906542023937006,-0.032516376311064,
-0.923182158835321));
#42378=CARTESIAN_POINT('Ctrl Pts',(0.0765016020707636,0.0585064442659452,
-0.916833268490676));
#42379=CARTESIAN_POINT('Ctrl Pts',(-0.00763650593860646,0.096006160828812,
-0.910484378146031));
#42380=CARTESIAN_POINT('Ctrl Pts',(-0.0847885544329253,0.0456771296954345,
-0.904135487801385));
#42381=CARTESIAN_POINT('Ctrl Pts',(-0.0843739916750971,-0.046438439560873,
-0.897786597456739));
#42382=CARTESIAN_POINT('Ctrl Pts',(-0.00677206965841167,-0.0960710060974691,
-0.891437707112095));
#42383=CARTESIAN_POINT('Ctrl Pts',(0.0770251047491154,-0.0578155029246153,
-0.885088816767449));
#42384=CARTESIAN_POINT('Ctrl Pts',(0.0903578586144035,0.0333310144858777,
-0.878739926422805));
#42385=CARTESIAN_POINT('Ctrl Pts',(0.0210290676568723,0.0939855172541015,
-0.872391036078158));
#42386=CARTESIAN_POINT('Ctrl Pts',(-0.0675376207603448,0.068659805724093,
-0.866042145733514));
#42387=CARTESIAN_POINT('Ctrl Pts',(-0.0943192674411041,-0.0194775493687425,
-0.859693255388868));
#42388=CARTESIAN_POINT('Ctrl Pts',(-0.0348153771160591,-0.0897963732914918,
-0.853344365044223));
#42389=CARTESIAN_POINT('Ctrl Pts',(0.0565384585278954,-0.0779673126850463,
-0.846995474699577));
#42390=CARTESIAN_POINT('Ctrl Pts',(0.0961695508987841,0.00518812297122139,
-0.840646584354933));
#42391=CARTESIAN_POINT('Ctrl Pts',(0.0478224224030806,0.0835973388065655,
-0.834297694010287));
#42392=CARTESIAN_POINT('Ctrl Pts',(-0.0442738096418514,0.085529696128511,
-0.827948803665642));
#42393=CARTESIAN_POINT('Ctrl Pts',(-0.0958672945399675,0.00921742792895202,
-0.821599913320997));
#42394=CARTESIAN_POINT('Ctrl Pts',(-0.0597590699666867,-0.0755271652900795,
-0.81525102297635));
#42395=CARTESIAN_POINT('Ctrl Pts',(0.0310181907742342,-0.0911776890534718,
-0.808902132631707));
#42396=CARTESIAN_POINT('Ctrl Pts',(0.0934192636956881,-0.0234166673673649,
-0.80255324228706));
#42397=CARTESIAN_POINT('Ctrl Pts',(0.0703581447091877,0.065766485485537,
-0.796204351942415));
#42398=CARTESIAN_POINT('Ctrl Pts',(-0.0170682992386754,0.0947848737992373,
-0.78985546159777));
#42399=CARTESIAN_POINT('Ctrl Pts',(-0.0888802520487178,0.037091777199195,
-0.783506571253126));
#42400=CARTESIAN_POINT('Ctrl Pts',(-0.0793824101020987,-0.0545337703301412,
-0.777157680908479));
#42401=CARTESIAN_POINT('Ctrl Pts',(0.00273637208614892,-0.0962705116213914,
-0.770808790563835));
#42402=CARTESIAN_POINT('Ctrl Pts',(0.0823518551998093,-0.0499366707459357,
-0.764459900219189));
#42403=CARTESIAN_POINT('Ctrl Pts',(0.086629878194021,0.0420804389726088,
-0.758111009874544));
#42404=CARTESIAN_POINT('Ctrl Pts',(0.011656802621483,0.0956013498475942,
-0.751762119529899));
#42405=CARTESIAN_POINT('Ctrl Pts',(-0.0739801966779158,0.0616638438595523,
-0.745413229185254));
#42406=CARTESIAN_POINT('Ctrl Pts',(-0.0919383306581472,-0.0286852313191213,
-0.739064338840609));
#42407=CARTESIAN_POINT('Ctrl Pts',(-0.0257890659331354,-0.0927923661641124,
-0.732715448495962));
#42408=CARTESIAN_POINT('Ctrl Pts',(0.0639526572925559,-0.0720108100583468,
-0.726366558151318));
#42409=CARTESIAN_POINT('Ctrl Pts',(0.0951889496858655,0.0146479690653711,
-0.720017667806673));
#42410=CARTESIAN_POINT('Ctrl Pts',(0.039344098814443,0.0879064333738871,
-0.713668777462027));
#42411=CARTESIAN_POINT('Ctrl Pts',(-0.0524936810344394,0.0807459756984393,
-0.707319887117383));
#42412=CARTESIAN_POINT('Ctrl Pts',(-0.0963089774570548,-0.000282844860001636,
-0.700970996772735));
#42413=CARTESIAN_POINT('Ctrl Pts',(-0.0520185022402654,-0.0810529121297798,
-0.694622106428093));
#42414=CARTESIAN_POINT('Ctrl Pts',(0.0398597513998638,-0.0876738236783333,
-0.688273216083445));
#42415=CARTESIAN_POINT('Ctrl Pts',(0.095273344660789,-0.0140886101935142,
-0.681924325738802));
#42416=CARTESIAN_POINT('Ctrl Pts',(0.0635285881017423,0.0723852031415087,
-0.675575435394155));
#42417=CARTESIAN_POINT('Ctrl Pts',(-0.0263336505826002,0.0926392896509459,
-0.669226545049511));
#42418=CARTESIAN_POINT('Ctrl Pts',(-0.092105231615666,0.0281447232898606,
-0.662877654704864));
#42419=CARTESIAN_POINT('Ctrl Pts',(-0.0736167289286767,-0.0620973136446348,
-0.656528764360221));
#42420=CARTESIAN_POINT('Ctrl Pts',(0.012218130028394,-0.0955312327914153,
-0.650179874015573));
#42421=CARTESIAN_POINT('Ctrl Pts',(0.0868755494303378,-0.0415708798465372,
-0.64383098367093));
#42422=CARTESIAN_POINT('Ctrl Pts',(0.0820571243029361,0.0504195149834954,
-0.637482093326283));
#42423=CARTESIAN_POINT('Ctrl Pts',(0.00217086597748532,0.0962849234353234,
-0.63113320298164));
#42424=CARTESIAN_POINT('Ctrl Pts',(-0.0797013528173027,0.0540665654460328,
-0.624784312636992));
#42425=CARTESIAN_POINT('Ctrl Pts',(-0.0886608548946474,-0.0376131885033519,
-0.618435422292349));
#42426=CARTESIAN_POINT('Ctrl Pts',(-0.0165112720148233,-0.0948834919071322,
-0.612086531947702));
#42427=CARTESIAN_POINT('Ctrl Pts',(0.0707432200855638,-0.0653520921774031,
-0.605737641603058));
#42428=CARTESIAN_POINT('Ctrl Pts',(0.0932801109978982,0.0239649751149068,
-0.599388751258413));
#42429=CARTESIAN_POINT('Ctrl Pts',(0.0304821102409294,0.091358306110053,
-0.593039860913766));
#42430=CARTESIAN_POINT('Ctrl Pts',(-0.0602016589551456,0.0751748588231912,
-0.586690970569124));
#42431=CARTESIAN_POINT('Ctrl Pts',(-0.0958115009196643,-0.00978035948007525,
-0.580342080224475));
#42432=CARTESIAN_POINT('Ctrl Pts',(-0.0437706747601158,-0.0857882694258514,
-0.573993189879833));
#42433=CARTESIAN_POINT('Ctrl Pts',(0.0483126186412545,-0.0833150047714283,
-0.567644299535184));
#42434=CARTESIAN_POINT('Ctrl Pts',(0.0961983651710867,-0.00462316757738183,
-0.561295409190541));
#42435=CARTESIAN_POINT('Ctrl Pts',(0.0560795308441945,0.0782980546395207,
-0.554946518845895));
#42436=CARTESIAN_POINT('Ctrl Pts',(-0.0353422086600146,0.0895903311025827,
-0.54859762850125));
#42437=CARTESIAN_POINT('Ctrl Pts',(-0.0944320446631196,0.0189232153922341,
-0.542248738156605));
#42438=CARTESIAN_POINT('Ctrl Pts',(-0.0671331723421136,-0.0690553134184647,
-0.53589984781196));
#42439=CARTESIAN_POINT('Ctrl Pts',(0.0215807425634793,-0.0938603787039407,
-0.529550957467314));
#42440=CARTESIAN_POINT('Ctrl Pts',(0.090552074520826,-0.0327997094501317,
-0.52320206712267));
#42441=CARTESIAN_POINT('Ctrl Pts',(0.0766841882675571,0.0582669238057431,
-0.516853176778024));
#42442=CARTESIAN_POINT('Ctrl Pts',(-0.00733623992155941,0.0960295721319826,
-0.510504286433379));
#42443=CARTESIAN_POINT('Ctrl Pts',(-0.0846452991782301,0.0459420555381036,
-0.504155396088733));
#42444=CARTESIAN_POINT('Ctrl Pts',(-0.0845188005392554,-0.0461743597188309,
-0.497806505744088));
#42445=CARTESIAN_POINT('Ctrl Pts',(-0.00707246800557763,-0.0960493588544368,
-0.491457615399443));
#42446=CARTESIAN_POINT('Ctrl Pts',(0.0768439285603362,-0.0580560916997712,
-0.485108725054797));
#42447=CARTESIAN_POINT('Ctrl Pts',(0.0904616489241209,0.0330482860972778,
-0.478759834710152));
#42448=CARTESIAN_POINT('Ctrl Pts',(0.0213228745905474,0.0939192959898768,
-0.472410944365507));
#42449=CARTESIAN_POINT('Ctrl Pts',(-0.0673225788603292,0.0688706723913238,
-0.466062054020862));
#42450=CARTESIAN_POINT('Ctrl Pts',(-0.0943797160829615,-0.0191825006747795,
-0.459713163676217));
#42451=CARTESIAN_POINT('Ctrl Pts',(-0.0350960164266517,-0.0896870602206277,
-0.453364273331571));
#42452=CARTESIAN_POINT('Ctrl Pts',(0.0562943641475219,-0.0781437374667004,
-0.447015382986926));
#42453=CARTESIAN_POINT('Ctrl Pts',(0.0961853048654396,0.00488735797550875,
-0.440666492642281));
#42454=CARTESIAN_POINT('Ctrl Pts',(0.0480836126087228,0.0834473806571098,
-0.434317602297635));
#42455=CARTESIAN_POINT('Ctrl Pts',(-0.0440061262866458,0.0856677301513364,
-0.42796871195299));
#42456=CARTESIAN_POINT('Ctrl Pts',(-0.0958380012141929,0.00951717727620129,
-0.421619821608344));
#42457=CARTESIAN_POINT('Ctrl Pts',(-0.0599949649101275,-0.0753399185390514,
-0.4152709312637));
#42458=CARTESIAN_POINT('Ctrl Pts',(0.030732909936045,-0.091274242735294,
-0.408922040919054));
#42459=CARTESIAN_POINT('Ctrl Pts',(0.0933455787429149,-0.023708691848952,
-0.402573150574409));
#42460=CARTESIAN_POINT('Ctrl Pts',(0.0705634644109166,0.0655461412317127,
-0.396224260229763));
#42461=CARTESIAN_POINT('Ctrl Pts',(-0.0167718062895594,0.0948377860023304,
-0.389875369885119));
#42462=CARTESIAN_POINT('Ctrl Pts',(-0.0887638247414365,0.0373695405017222,
-0.383526479540473));
#42463=CARTESIAN_POINT('Ctrl Pts',(-0.0795525589408519,-0.0542852604857035,
-0.377177589195828));
#42464=CARTESIAN_POINT('Ctrl Pts',(0.00243530335613392,-0.0962785980247009,
-0.370828698851183));
#42465=CARTESIAN_POINT('Ctrl Pts',(0.0821952915023019,-0.0501939557605288,
-0.364479808506538));
#42466=CARTESIAN_POINT('Ctrl Pts',(0.0867610477694602,0.0418093258733485,
-0.358130918161892));
#42467=CARTESIAN_POINT('Ctrl Pts',(0.0119557083837728,0.0955644294551089,
-0.351782027817247));
#42468=CARTESIAN_POINT('Ctrl Pts',(-0.0737870009175868,0.0618948918379082,
-0.345433137472602));
#42469=CARTESIAN_POINT('Ctrl Pts',(-0.0920275850333652,-0.0283975832240196,
-0.339084247127956));
#42470=CARTESIAN_POINT('Ctrl Pts',(-0.0260791183922587,-0.0927112653560552,
-0.332735356783311));
#42471=CARTESIAN_POINT('Ctrl Pts',(0.0637271537234194,-0.0722104495094026,
-0.326386466438666));
#42472=CARTESIAN_POINT('Ctrl Pts',(0.095234291101752,0.0143502243322243,
-0.32003757609402));
#42473=CARTESIAN_POINT('Ctrl Pts',(0.0396188057963046,0.087782967410045,
-0.313688685749375));
#42474=CARTESIAN_POINT('Ctrl Pts',(-0.0522409170483859,0.0809097381406094,
-0.30733979540473));
#42475=CARTESIAN_POINT('Ctrl Pts',(-0.0963093910476554,1.83321627840156E-5,
-0.300990905060085));
#42476=CARTESIAN_POINT('Ctrl Pts',(-0.0522717150448785,-0.0808898445189835,
-0.294642014715439));
#42477=CARTESIAN_POINT('Ctrl Pts',(0.0395853845521076,-0.087798043656451,
-0.288293124370794));
#42478=CARTESIAN_POINT('Ctrl Pts',(0.0952288211688058,-0.0143864783334232,
-0.281944234026149));
#42479=CARTESIAN_POINT('Ctrl Pts',(0.063754639128095,0.0721861837866822,
-0.275595343681504));
#42480=CARTESIAN_POINT('Ctrl Pts',(-0.0260438219599888,0.092721186779261,
-0.269246453336858));
#42481=CARTESIAN_POINT('Ctrl Pts',(-0.0920167675996606,0.0284326154363034,
-0.262897562992213));
#42482=CARTESIAN_POINT('Ctrl Pts',(-0.0738105585312733,-0.061866797147901,
-0.256548672647567));
#42483=CARTESIAN_POINT('Ctrl Pts',(0.0119193267949383,-0.0955689739862951,
-0.250199782302923));
#42484=CARTESIAN_POINT('Ctrl Pts',(0.0867451249590103,-0.041842352179179,
-0.243850891958277));
#42485=CARTESIAN_POINT('Ctrl Pts',(0.0822143940406088,0.0501626609399,-0.237502001613632));
#42486=CARTESIAN_POINT('Ctrl Pts',(0.00247195578125156,0.0962776639447085,
-0.231153111268987));
#42487=CARTESIAN_POINT('Ctrl Pts',(-0.0795318871501312,0.0543155416652873,
-0.224804220924341));
#42488=CARTESIAN_POINT('Ctrl Pts',(-0.0887780446367585,-0.0373357460149329,
-0.218455330579696));
#42489=CARTESIAN_POINT('Ctrl Pts',(-0.0168079091687892,-0.0948313942183441,
-0.212106440235051));
#42490=CARTESIAN_POINT('Ctrl Pts',(0.0705385063320063,-0.0655729995089186,
-0.205757549890406));
#42491=CARTESIAN_POINT('Ctrl Pts',(0.0933545977140429,0.0236731541102014,
-0.19940865954576));
#42492=CARTESIAN_POINT('Ctrl Pts',(0.0307676551887473,0.0912625363123725,
-0.193059769201115));
#42493=CARTESIAN_POINT('Ctrl Pts',(-0.0599662791762946,0.0753627527528736,
-0.18671087885647));
#42494=CARTESIAN_POINT('Ctrl Pts',(-0.0958416173867071,-0.00948069172061055,
-0.180361988511825));
#42495=CARTESIAN_POINT('Ctrl Pts',(-0.044038736227651,-0.0856509711067653,
-0.174013098167179));
#42496=CARTESIAN_POINT('Ctrl Pts',(0.0480518413036898,-0.0834656797238674,
-0.167664207822534));
#42497=CARTESIAN_POINT('Ctrl Pts',(0.0961834372655269,-0.00492397468347903,
-0.161315317477889));
#42498=CARTESIAN_POINT('Ctrl Pts',(0.0563241089406863,0.0781223008817196,
-0.154966427133243));
#42499=CARTESIAN_POINT('Ctrl Pts',(-0.0350618708017759,0.0897004146181866,
-0.148617536788598));
#42500=CARTESIAN_POINT('Ctrl Pts',(-0.0943724062814499,0.0192184288356559,
-0.142268646443953));
#42501=CARTESIAN_POINT('Ctrl Pts',(-0.0673487931736204,-0.0688450378548037,
-0.135919756099307));
#42502=CARTESIAN_POINT('Ctrl Pts',(0.0212871197506783,-0.0939274072291657,
-0.129570865754662));
#42503=CARTESIAN_POINT('Ctrl Pts',(0.0904490589574556,-0.0330827207447464,
-0.123221975410017));
#42504=CARTESIAN_POINT('Ctrl Pts',(0.0768660286360105,0.0580268314756966,
-0.116873085065372));
#42505=CARTESIAN_POINT('Ctrl Pts',(-0.00703590991483225,0.0960520482427784,
-0.110524194720726));
#42506=CARTESIAN_POINT('Ctrl Pts',(-0.0845012014484307,0.0462065246880186,
-0.104175304376081));
#42507=CARTESIAN_POINT('Ctrl Pts',(-0.0846628107564522,-0.04590981426736,
-0.0978264140314358));
#42508=CARTESIAN_POINT('Ctrl Pts',(-0.00737274430247539,-0.0960267989761889,
-0.0914775236867905));
#42509=CARTESIAN_POINT('Ctrl Pts',(0.0766619005942514,-0.0582960621693097,
-0.0851286333421456));
#42510=CARTESIAN_POINT('Ctrl Pts',(0.0905647447976647,0.0327651386368324,
-0.0787797429975001));
#42511=CARTESIAN_POINT('Ctrl Pts',(0.0216161122636334,0.0938523381026498,
-0.072430852652855));
#42512=CARTESIAN_POINT('Ctrl Pts',(-0.0671061944597261,0.0690805206944129,
-0.0660819623082095));
#42513=CARTESIAN_POINT('Ctrl Pts',(-0.094440539208817,-0.0188866103704566,
-0.0597330719635644));
#42514=CARTESIAN_POINT('Ctrl Pts',(-0.0353738519088489,-0.0895781104263087,
-0.0533841816189191));
#42515=CARTESIAN_POINT('Ctrl Pts',(0.0560450525467761,-0.0783170456163444,
-0.0470352912742739));
#42516=CARTESIAN_POINT('Ctrl Pts',(0.0962089701220667,0.00458208267517972,
-0.0406864009296285));
#42517=CARTESIAN_POINT('Ctrl Pts',(0.0483275316587034,0.0833050791594327,
-0.0343375105849833));
#42518=CARTESIAN_POINT('Ctrl Pts',(-0.0437060368403489,0.08578877695719,
-0.027988620240338));
#42519=CARTESIAN_POINT('Ctrl Pts',(-0.095869363633284,0.00984814280277796,
-0.0216397298956927));
#42520=CARTESIAN_POINT('Ctrl Pts',(-0.0601054769427006,-0.0752169878654165,
-0.0152908395510473));
#42521=CARTESIAN_POINT('Ctrl Pts',(6.21869452505711E-5,-0.0858764120339165,
-0.0110582459879505));
#42522=CARTESIAN_POINT('Ctrl Pts',(0.0257628407500271,-0.0773121450523775,
-0.00894194920640216));
#42523=CARTESIAN_POINT('Ctrl Pts',(0.0800079576859287,0.0391735495545708,
-1.1537080507936));
#42524=CARTESIAN_POINT('Ctrl Pts',(0.0669856073847669,0.0657703645921076,
-1.15159175401205));
#42525=CARTESIAN_POINT('Ctrl Pts',(0.0125622154273748,0.104499379851189,
-1.14735916044895));
#42526=CARTESIAN_POINT('Ctrl Pts',(-0.0811541182039119,0.0671791560281841,
-1.14101027010431));
#42527=CARTESIAN_POINT('Ctrl Pts',(-0.100367548684175,-0.0316841982689489,
-1.13466137975966));
#42528=CARTESIAN_POINT('Ctrl Pts',(-0.0278936765835931,-0.101517854627537,
-1.12831248941502));
#42529=CARTESIAN_POINT('Ctrl Pts',(0.0701665010789239,-0.078503723520769,
-1.12196359907037));
#42530=CARTESIAN_POINT('Ctrl Pts',(0.104000645581044,0.0163397166628863,
-1.11561470872573));
#42531=CARTESIAN_POINT('Ctrl Pts',(0.0427114819908452,0.0962287529105411,
-1.10926581838108));
#42532=CARTESIAN_POINT('Ctrl Pts',(-0.0576611840811396,0.0880888031830703,
-1.10291692803644));
#42533=CARTESIAN_POINT('Ctrl Pts',(-0.105278732315225,-0.000638694591246696,
-1.09656803769179));
#42534=CARTESIAN_POINT('Ctrl Pts',(-0.0565875443108695,-0.0887809554458167,
-1.09021914734715));
#42535=CARTESIAN_POINT('Ctrl Pts',(0.0438727593435398,-0.0957047580870532,
-1.0838702570025));
#42536=CARTESIAN_POINT('Ctrl Pts',(0.104196432509398,-0.0150752811268102,
-1.07752136665786));
#42537=CARTESIAN_POINT('Ctrl Pts',(0.0691991082535025,0.0793452876551954,
-1.07117247631321));
#42538=CARTESIAN_POINT('Ctrl Pts',(-0.0291034416533303,0.101178949658241,
-1.06482358596857));
#42539=CARTESIAN_POINT('Ctrl Pts',(-0.100781348896612,0.0304516337180169,
-1.05847469562392));
#42540=CARTESIAN_POINT('Ctrl Pts',(-0.080262111234698,-0.068133549720299,
-1.05212580527927));
#42541=CARTESIAN_POINT('Ctrl Pts',(0.0136828699897497,-0.104388531955573,
-1.04577691493463));
#42542=CARTESIAN_POINT('Ctrl Pts',(0.0951104156404598,-0.0451463659057333,
-1.03942802458998));
#42543=CARTESIAN_POINT('Ctrl Pts',(0.0895286716321017,0.0553967797979785,
-1.03307913424534));
#42544=CARTESIAN_POINT('Ctrl Pts',(0.00204393839436774,0.105261618989727,
-1.02673024390069));
#42545=CARTESIAN_POINT('Ctrl Pts',(-0.087310636464981,0.0588305936669936,
-1.02038135355605));
#42546=CARTESIAN_POINT('Ctrl Pts',(-0.0967913399847819,-0.041420074911301,
-1.0140324632114));
#42547=CARTESIAN_POINT('Ctrl Pts',(-0.0177249943318654,-0.103778661820372,
-1.00768357286676));
#42548=CARTESIAN_POINT('Ctrl Pts',(0.0775566025854628,-0.0711980298477954,
-1.00133468252211));
#42549=CARTESIAN_POINT('Ctrl Pts',(0.101887552130213,0.0265162741709498,
-0.994985792177467));
#42550=CARTESIAN_POINT('Ctrl Pts',(0.0330093154964704,0.0999728521160336,
-0.988636901832822));
#42551=CARTESIAN_POINT('Ctrl Pts',(-0.0660666377453062,0.0819718576420304,
-0.982288011488176));
#42552=CARTESIAN_POINT('Ctrl Pts',(-0.104703239960795,-0.0110189660260845,
-0.97593912114353));
#42553=CARTESIAN_POINT('Ctrl Pts',(-0.0475547970551419,-0.0939293742484679,
-0.969590230798886));
#42554=CARTESIAN_POINT('Ctrl Pts',(0.0530979192795061,-0.0909109291434562,
-0.96324134045424));
#42555=CARTESIAN_POINT('Ctrl Pts',(0.105175380495662,-0.0047249769794186,
-0.956892450109596));
#42556=CARTESIAN_POINT('Ctrl Pts',(0.061035871072958,0.0857834979006917,
-0.950543559764949));
#42557=CARTESIAN_POINT('Ctrl Pts',(-0.0389407229128716,0.0978151632863322,
-0.944194669420305));
#42558=CARTESIAN_POINT('Ctrl Pts',(-0.10329340590964,0.0203631619681055,
-0.937845779075658));
#42559=CARTESIAN_POINT('Ctrl Pts',(-0.0731507939374694,-0.0757175502512242,
-0.931496888731016));
#42560=CARTESIAN_POINT('Ctrl Pts',(0.0239119257552284,-0.102530024268049,
-0.925147998386367));
#42561=CARTESIAN_POINT('Ctrl Pts',(0.0990994399824792,-0.0355455632237716,
-0.918799108041724));
#42562=CARTESIAN_POINT('Ctrl Pts',(0.0836284002593778,0.0639568349732043,
-0.912450217697077));
#42563=CARTESIAN_POINT('Ctrl Pts',(-0.00834791374207134,0.104949980494938,
-0.906101327352435));
#42564=CARTESIAN_POINT('Ctrl Pts',(-0.0926873552395928,0.0499323567281097,
-0.899752437007785));
#42565=CARTESIAN_POINT('Ctrl Pts',(-0.0922341723087004,-0.0507645893144231,
-0.893403546663144));
#42566=CARTESIAN_POINT('Ctrl Pts',(-0.00740294760695452,-0.105020866671638,
-0.887054656318496));
#42567=CARTESIAN_POINT('Ctrl Pts',(0.0842006718241181,-0.0632015263589454,
-0.880705765973852));
#42568=CARTESIAN_POINT('Ctrl Pts',(0.0987754891694415,0.0364360921212848,
-0.874356875629206));
#42569=CARTESIAN_POINT('Ctrl Pts',(0.022988110568765,0.102741096169992,
-0.868007985284561));
#42570=CARTESIAN_POINT('Ctrl Pts',(-0.0738293451199607,0.0750560714991865,
-0.861659094939917));
#42571=CARTESIAN_POINT('Ctrl Pts',(-0.10310593812715,-0.0212920546836966,
-0.85531020459527));
#42572=CARTESIAN_POINT('Ctrl Pts',(-0.0380587362072462,-0.0981616965421876,
-0.848961314250626));
#42573=CARTESIAN_POINT('Ctrl Pts',(0.0618055140263025,-0.0852306547298433,
-0.842612423905979));
#42574=CARTESIAN_POINT('Ctrl Pts',(0.105128591789345,0.00567144233176898,
-0.836263533561335));
#42575=CARTESIAN_POINT('Ctrl Pts',(0.0522775023508458,0.0913851673833921,
-0.829914643216689));
#42576=CARTESIAN_POINT('Ctrl Pts',(-0.048398305048717,0.0934975408133528,
-0.823565752872045));
#42577=CARTESIAN_POINT('Ctrl Pts',(-0.104798177587918,0.0100761125432544,
-0.817216862527398));
#42578=CARTESIAN_POINT('Ctrl Pts',(-0.0653261537932172,-0.0825631861080844,
-0.810867972182754));
#42579=CARTESIAN_POINT('Ctrl Pts',(0.033907808505632,-0.0996716940363645,
-0.804519081838107));
#42580=CARTESIAN_POINT('Ctrl Pts',(0.102122091104091,-0.0255981362263135,
-0.798170191493465));
#42581=CARTESIAN_POINT('Ctrl Pts',(0.07691262572259,0.0718932129911442,
-0.791821301148816));
#42582=CARTESIAN_POINT('Ctrl Pts',(-0.0186583616792568,0.103614919819393,
-0.785472410804175));
#42583=CARTESIAN_POINT('Ctrl Pts',(-0.0971602305349011,0.0405472030125148,
-0.779123520459527));
#42584=CARTESIAN_POINT('Ctrl Pts',(-0.0867775809378697,-0.0596140714622373,
-0.772774630114882));
#42585=CARTESIAN_POINT('Ctrl Pts',(0.00299128925257632,-0.105238957892696,
-0.766425739770237));
#42586=CARTESIAN_POINT('Ctrl Pts',(0.090023656006337,-0.0545887115527192,
-0.760076849425591));
#42587=CARTESIAN_POINT('Ctrl Pts',(0.0947002145305326,0.0460006025787094,
-0.753727959080947));
#42588=CARTESIAN_POINT('Ctrl Pts',(0.0127427364785399,0.104507457804559,
-0.7473790687363));
#42589=CARTESIAN_POINT('Ctrl Pts',(-0.0808721037413772,0.0674083741546789,
-0.741030178391657));
#42590=CARTESIAN_POINT('Ctrl Pts',(-0.100503196107536,-0.0313575133246159,
-0.73468128804701));
#42591=CARTESIAN_POINT('Ctrl Pts',(-0.0281915446185915,-0.101436792544674,
-0.728332397702365));
#42592=CARTESIAN_POINT('Ctrl Pts',(0.0699104107227152,-0.0787192514084998,
-0.721983507357721));
#42593=CARTESIAN_POINT('Ctrl Pts',(0.104056638934646,0.0160125564279404,
-0.715634617013074));
#42594=CARTESIAN_POINT('Ctrl Pts',(0.043009348228488,0.0960956920714652,
-0.70928572666843));
#42595=CARTESIAN_POINT('Ctrl Pts',(-0.0573839298760781,0.0882681746821054,
-0.702936836323783));
#42596=CARTESIAN_POINT('Ctrl Pts',(-0.105281007159824,-0.000309194350488767,
-0.696587945979139));
#42597=CARTESIAN_POINT('Ctrl Pts',(-0.0568644839910446,-0.0886037049460429,
-0.690239055634493));
#42598=CARTESIAN_POINT('Ctrl Pts',(0.0435730383949847,-0.0958414127335492,
-0.683890165289848));
#42599=CARTESIAN_POINT('Ctrl Pts',(0.104148896044978,-0.015401088349387,
-0.677541274945203));
#42600=CARTESIAN_POINT('Ctrl Pts',(0.0694468357508554,0.0791285225056486,
-0.671192384600558));
#42601=CARTESIAN_POINT('Ctrl Pts',(-0.0287868621257805,0.101269455605748,
-0.664843494255913));
#42602=CARTESIAN_POINT('Ctrl Pts',(-0.100685645359594,0.0307666522107167,
-0.658494603911267));
#42603=CARTESIAN_POINT('Ctrl Pts',(-0.0804747757692551,-0.06788222546898,
-0.652145713566622));
#42604=CARTESIAN_POINT('Ctrl Pts',(0.01335635647853,-0.104430808726887,
-0.645796823221977));
#42605=CARTESIAN_POINT('Ctrl Pts',(0.094968772206802,-0.0454435735309818,
-0.639447932877331));
#42606=CARTESIAN_POINT('Ctrl Pts',(0.0897014683299295,0.0551165369847199,
-0.633099042532686));
#42607=CARTESIAN_POINT('Ctrl Pts',(0.00237310126795229,0.10525471229406,
-0.626750152188041));
#42608=CARTESIAN_POINT('Ctrl Pts',(-0.0871262359767842,0.05910334232724,
-0.620401261843395));
#42609=CARTESIAN_POINT('Ctrl Pts',(-0.0969203946031063,-0.0411171883731305,
-0.61405237149875));
#42610=CARTESIAN_POINT('Ctrl Pts',(-0.0180494424622608,-0.103722725072834,
-0.607703481154104));
#42611=CARTESIAN_POINT('Ctrl Pts',(0.0773335742626736,-0.0714402152956775,
-0.601354590809461));
#42612=CARTESIAN_POINT('Ctrl Pts',(0.101969975106609,0.0261975236709649,
-0.595005700464813));
#42613=CARTESIAN_POINT('Ctrl Pts',(0.033321787347942,0.0998691371629481,
-0.58865681012017));
#42614=CARTESIAN_POINT('Ctrl Pts',(-0.0658099738450268,0.0821780591900918,
-0.582307919775524));
#42615=CARTESIAN_POINT('Ctrl Pts',(-0.104737186300359,-0.0106914861276222,
-0.575959029430879));
#42616=CARTESIAN_POINT('Ctrl Pts',(-0.047848298720281,-0.0937802024912932,
-0.569610139086233));
#42617=CARTESIAN_POINT('Ctrl Pts',(0.0528133646870868,-0.0910765314456041,
-0.563261248741589));
#42618=CARTESIAN_POINT('Ctrl Pts',(0.105160090364957,-0.00505385636590638,
-0.556912358396943));
#42619=CARTESIAN_POINT('Ctrl Pts',(0.0613038331858501,0.0855922082111139,
-0.550563468052297));
#42620=CARTESIAN_POINT('Ctrl Pts',(-0.0386346467507483,0.0979364597082119,
-0.544214577707653));
#42621=CARTESIAN_POINT('Ctrl Pts',(-0.10322922154093,0.0206860796137611,
-0.537865687363007));
#42622=CARTESIAN_POINT('Ctrl Pts',(-0.0733872187685025,-0.0754884242195927,
-0.531516797018362));
#42623=CARTESIAN_POINT('Ctrl Pts',(0.0235911788530122,-0.10260429986145,
-0.525167906673717));
#42624=CARTESIAN_POINT('Ctrl Pts',(0.098987797998531,-0.0358552913408218,
-0.518819016329071));
#42625=CARTESIAN_POINT('Ctrl Pts',(0.083827995968931,0.0636950010720324,
-0.512470125984427));
#42626=CARTESIAN_POINT('Ctrl Pts',(-0.00801967530028448,0.104975572767245,
-0.50612123563978));
#42627=CARTESIAN_POINT('Ctrl Pts',(-0.0925307544958878,0.050221962746939,
-0.499772345295136));
#42628=CARTESIAN_POINT('Ctrl Pts',(-0.0923924713942769,-0.050475908108632,
-0.49342345495049));
#42629=CARTESIAN_POINT('Ctrl Pts',(-0.0077313307065766,-0.104997202797211,
-0.487074564605845));
#42630=CARTESIAN_POINT('Ctrl Pts',(0.0840026174772474,-0.0634645280980206,
-0.480725674261199));
#42631=CARTESIAN_POINT('Ctrl Pts',(0.0988889484608699,0.0361270250925362,
-0.474376783916555));
#42632=CARTESIAN_POINT('Ctrl Pts',(0.0233092882066613,0.102668705811615,
-0.468027893571909));
#42633=CARTESIAN_POINT('Ctrl Pts',(-0.0735942701725054,0.0752865822541408,
-0.461679003227264));
#42634=CARTESIAN_POINT('Ctrl Pts',(-0.10317201809253,-0.0209695196046023,
-0.455330112882619));
#42635=CARTESIAN_POINT('Ctrl Pts',(-0.0383655195419671,-0.0980421999957576,
-0.448981222537972));
#42636=CARTESIAN_POINT('Ctrl Pts',(0.0615386801040004,-0.085423515034157,
-0.442632332193329));
#42637=CARTESIAN_POINT('Ctrl Pts',(0.105145813376782,0.00534265842705816,
-0.436283441848682));
#42638=CARTESIAN_POINT('Ctrl Pts',(0.0525630247251494,0.0912212393112291,
-0.429934551504037));
#42639=CARTESIAN_POINT('Ctrl Pts',(-0.0481056846307652,0.0936484339214419,
-0.423585661159393));
#42640=CARTESIAN_POINT('Ctrl Pts',(-0.104766155330783,0.0104037861829001,
-0.417236770814747));
#42641=CARTESIAN_POINT('Ctrl Pts',(-0.0655840244288016,-0.0823584956726115,
-0.410887880470102));
#42642=CARTESIAN_POINT('Ctrl Pts',(0.0335959512441284,-0.0997772425442569,
-0.404538990125456));
#42643=CARTESIAN_POINT('Ctrl Pts',(0.102041541748826,-0.0259173653610067,
-0.398190099780811));
#42644=CARTESIAN_POINT('Ctrl Pts',(0.0771370727633386,0.0716523417289106,
-0.391841209436165));
#42645=CARTESIAN_POINT('Ctrl Pts',(-0.0183342477999184,0.103672761260345,
-0.385492319091521));
#42646=CARTESIAN_POINT('Ctrl Pts',(-0.0970329569982577,0.0408508424136822,
-0.379143428746875));
#42647=CARTESIAN_POINT('Ctrl Pts',(-0.0869635806399119,-0.0593424107364946,
-0.37279453840223));
#42648=CARTESIAN_POINT('Ctrl Pts',(0.00266217331803697,-0.105247797615712,
-0.366445648057585));
#42649=CARTESIAN_POINT('Ctrl Pts',(0.0898525070211284,-0.054869964933024,
-0.36009675771294));
#42650=CARTESIAN_POINT('Ctrl Pts',(0.0948436037074879,0.0457042329058294,
-0.353747867368294));
#42651=CARTESIAN_POINT('Ctrl Pts',(0.0130694879458553,0.104467097952257,
-0.347398977023649));
#42652=CARTESIAN_POINT('Ctrl Pts',(-0.080660910093978,0.0676609462876806,
-0.341050086679004));
#42653=CARTESIAN_POINT('Ctrl Pts',(-0.100600765314109,-0.0310430682753637,
-0.334701196334358));
#42654=CARTESIAN_POINT('Ctrl Pts',(-0.0285086180195555,-0.101348136481873,
-0.328352305989713));
#42655=CARTESIAN_POINT('Ctrl Pts',(0.0696638995094961,-0.078937489033184,
-0.322003415645068));
#42656=CARTESIAN_POINT('Ctrl Pts',(0.104106204302866,0.015687074149861,
-0.315654525300422));
#42657=CARTESIAN_POINT('Ctrl Pts',(0.0433096465857946,0.0959607241653938,
-0.309305634955778));
#42658=CARTESIAN_POINT('Ctrl Pts',(-0.0571076186979503,0.0884471930384607,
-0.302956744611132));
#42659=CARTESIAN_POINT('Ctrl Pts',(-0.105281459280032,2.00399652468685E-5,
-0.296607854266487));
#42660=CARTESIAN_POINT('Ctrl Pts',(-0.0571412857991351,-0.0884254461507251,
-0.290258963921841));
#42661=CARTESIAN_POINT('Ctrl Pts',(0.043273111858272,-0.0959772048969685,
-0.283910073577196));
#42662=CARTESIAN_POINT('Ctrl Pts',(0.104100224797478,-0.0157267055306558,
-0.277561183232551));
#42663=CARTESIAN_POINT('Ctrl Pts',(0.0696939454217535,0.0789109627446204,
-0.271212292887905));
#42664=CARTESIAN_POINT('Ctrl Pts',(-0.0284700334136715,0.101358982173054,
-0.264863402543261));
#42665=CARTESIAN_POINT('Ctrl Pts',(-0.100588940141157,0.0310813640468423,
-0.258514512198615));
#42666=CARTESIAN_POINT('Ctrl Pts',(-0.0806866623069133,-0.0676302343297956,
-0.25216562185397));
#42667=CARTESIAN_POINT('Ctrl Pts',(0.0130297170915128,-0.104472065846558,
-0.245816731509324));
#42668=CARTESIAN_POINT('Ctrl Pts',(0.0948261975469705,-0.0457403359029975,
-0.239467841164679));
#42669=CARTESIAN_POINT('Ctrl Pts',(0.0898733891291647,0.0548357547241582,
-0.233118950820034));
#42670=CARTESIAN_POINT('Ctrl Pts',(0.00270224023944843,0.10524677651794,
-0.226770060475389));
#42671=CARTESIAN_POINT('Ctrl Pts',(-0.086940983089775,0.0593755128747225,
-0.220421170130743));
#42672=CARTESIAN_POINT('Ctrl Pts',(-0.0970485016021008,-0.0408138996727319,
-0.214072279786098));
#42673=CARTESIAN_POINT('Ctrl Pts',(-0.0183737139804013,-0.103665774025371,
-0.207723389441453));
#42674=CARTESIAN_POINT('Ctrl Pts',(0.0771097896195066,-0.0716817020912496,
-0.201374499096807));
#42675=CARTESIAN_POINT('Ctrl Pts',(0.102051400916568,0.0258785169688173,
-0.195025608752163));
#42676=CARTESIAN_POINT('Ctrl Pts',(0.0336339333232127,0.0997644455649112,
-0.188676718407517));
#42677=CARTESIAN_POINT('Ctrl Pts',(-0.0655526663661519,0.082383457094612,
-0.182327828062872));
#42678=CARTESIAN_POINT('Ctrl Pts',(-0.104770108381624,-0.010363901676382,
-0.175978937718226));
#42679=CARTESIAN_POINT('Ctrl Pts',(-0.0481413324750565,-0.0936301136242282,
-0.169630047373582));
#42680=CARTESIAN_POINT('Ctrl Pts',(0.0525282936431593,-0.0912412430972631,
-0.163281157028936));
#42681=CARTESIAN_POINT('Ctrl Pts',(0.105143771793484,-0.00538268630395523,
-0.156932266684291));
#42682=CARTESIAN_POINT('Ctrl Pts',(0.0615711958866884,0.0854000814424367,
-0.150583376339645));
#42683=CARTESIAN_POINT('Ctrl Pts',(-0.0383281929513239,0.0980567984730965,
-0.144234485995));
#42684=CARTESIAN_POINT('Ctrl Pts',(-0.103164027318611,0.0210087947901778,
-0.137885595650355));
#42685=CARTESIAN_POINT('Ctrl Pts',(-0.0736229265800177,-0.0752585596347131,
-0.13153670530571));
#42686=CARTESIAN_POINT('Ctrl Pts',(0.0232702024884716,-0.102677572684301,
-0.125187814961064));
#42687=CARTESIAN_POINT('Ctrl Pts',(0.0988751856278969,-0.0361646676307727,
-0.118838924616419));
#42688=CARTESIAN_POINT('Ctrl Pts',(0.084026776369664,0.0634325420263019,
-0.112490034271774));
#42689=CARTESIAN_POINT('Ctrl Pts',(-0.00769136690761526,0.10500014272577,
-0.106141143927129));
#42690=CARTESIAN_POINT('Ctrl Pts',(-0.0923732327931005,0.050511069528061,
-0.0997922535824832));
#42691=CARTESIAN_POINT('Ctrl Pts',(-0.0925498974318917,-0.0501867179177923,
-0.093443363237838));
#42692=CARTESIAN_POINT('Ctrl Pts',(-0.00805958038587264,-0.104972541267559,
-0.0870944728931927));
#42693=CARTESIAN_POINT('Ctrl Pts',(0.0838036320025109,-0.0637268539308632,
-0.0807455825485475));
#42694=CARTESIAN_POINT('Ctrl Pts',(0.0990016486232777,0.0358174999517078,
-0.0743966922039025));
#42695=CARTESIAN_POINT('Ctrl Pts',(0.0236298435523293,0.102595510207315,
-0.0680478018592568));
#42696=CARTESIAN_POINT('Ctrl Pts',(-0.0733577276587055,0.0755159797753619,
-0.0616989115146119));
#42697=CARTESIAN_POINT('Ctrl Pts',(-0.103238507428393,-0.0206460645117284,
-0.0553500211699664));
#42698=CARTESIAN_POINT('Ctrl Pts',(-0.0386692378469765,-0.0979231005682837,
-0.0490011308253213));
#42699=CARTESIAN_POINT('Ctrl Pts',(0.061266142931286,-0.0856129683647319,
-0.0426522404806759));
#42700=CARTESIAN_POINT('Ctrl Pts',(0.105171683260548,0.00500894404312121,
-0.0363033501360307));
#42701=CARTESIAN_POINT('Ctrl Pts',(0.0528296669834879,0.0910656811754109,
-0.0299544597913853));
#42702=CARTESIAN_POINT('Ctrl Pts',(-0.0477776392088496,0.0937807573036459,
-0.0236055694467402));
#42703=CARTESIAN_POINT('Ctrl Pts',(-0.104800439435505,0.0107655840639825,
-0.0172566791020948));
#42704=CARTESIAN_POINT('Ctrl Pts',(-0.0657048316307863,-0.0822241129237459,
-0.0109077887574495));
#42705=CARTESIAN_POINT('Ctrl Pts',(6.79802070497962E-5,-0.0938765563598085,
-0.00667519519435267));
#42706=CARTESIAN_POINT('Ctrl Pts',(0.028162876328643,-0.0845144524603652,
-0.00455889841280429));
#42707=CARTESIAN_POINT('Ctrl Pts',(0.08682622236805,0.0425119128515047,
-1.149325));
#42708=CARTESIAN_POINT('Ctrl Pts',(0.0726941095669478,0.0713753039881243,
-1.14720870321845));
#42709=CARTESIAN_POINT('Ctrl Pts',(0.0136327653108478,0.113404799406328,
-1.14297610965536));
#42710=CARTESIAN_POINT('Ctrl Pts',(-0.0880700584923845,0.0729041523931668,
-1.13662721931071));
#42711=CARTESIAN_POINT('Ctrl Pts',(-0.108920854282986,-0.0343843203103918,
-1.13027832896607));
#42712=CARTESIAN_POINT('Ctrl Pts',(-0.030270771005262,-0.110169189105151,
-1.12392943862142));
#42713=CARTESIAN_POINT('Ctrl Pts',(0.0761460784861183,-0.0851937976206204,
-1.11758054827678));
#42714=CARTESIAN_POINT('Ctrl Pts',(0.112863563085659,0.01773218456559,-1.11123165793213));
#42715=CARTESIAN_POINT('Ctrl Pts',(0.0463513472942736,0.10442935103042,
-1.10488276758748));
#42716=CARTESIAN_POINT('Ctrl Pts',(-0.0625750604794491,0.0955957161577918,
-1.09853387724284));
#42717=CARTESIAN_POINT('Ctrl Pts',(-0.11425056815612,-0.000693124036769614,
-1.09218498689819));
#42718=CARTESIAN_POINT('Ctrl Pts',(-0.0614099253087358,-0.0963468535198246,
-1.08583609655355));
#42719=CARTESIAN_POINT('Ctrl Pts',(0.0476115885074291,-0.103860701456305,
-1.0794872062089));
#42720=CARTESIAN_POINT('Ctrl Pts',(0.11307603494308,-0.0163599940460347,
-1.07313831586426));
#42721=CARTESIAN_POINT('Ctrl Pts',(0.075096244607004,0.0861070797088801,
-1.06678942551961));
#42722=CARTESIAN_POINT('Ctrl Pts',(-0.0315836320505423,0.109801402711436,
-1.06044053517497));
#42723=CARTESIAN_POINT('Ctrl Pts',(-0.109369918479851,0.0330467168159683,
-1.05409164483032));
#42724=CARTESIAN_POINT('Ctrl Pts',(-0.0871020348394502,-0.0739398793550231,
-1.04774275448568));
#42725=CARTESIAN_POINT('Ctrl Pts',(0.0148489218663328,-0.113284505071712,
-1.04139386414103));
#42726=CARTESIAN_POINT('Ctrl Pts',(0.10321570924649,-0.0489937316063985,
-1.03504497379639));
#42727=CARTESIAN_POINT('Ctrl Pts',(0.0971582899536019,0.0601176840445611,
-1.02869608345174));
#42728=CARTESIAN_POINT('Ctrl Pts',(0.00221812248017289,0.114231996435905,
-1.02234719310709));
#42729=CARTESIAN_POINT('Ctrl Pts',(-0.0947512342030169,0.0638441269533003,
-1.01599830276245));
#42730=CARTESIAN_POINT('Ctrl Pts',(-0.105039881680398,-0.0449498867208618,
-1.0096494124178));
#42731=CARTESIAN_POINT('Ctrl Pts',(-0.0192355153642617,-0.112622661906281,
-1.00330052207316));
#42732=CARTESIAN_POINT('Ctrl Pts',(0.0841659631986869,-0.0772655139629808,
-0.996951631728514));
#42733=CARTESIAN_POINT('Ctrl Pts',(0.110570392166754,0.0287759865909447,
-0.990602741383869));
#42734=CARTESIAN_POINT('Ctrl Pts',(0.0358223638049151,0.108492521739767,
-0.984253851039224));
#42735=CARTESIAN_POINT('Ctrl Pts',(-0.0716968254895517,0.0889574855477255,
-0.977904960694578));
#42736=CARTESIAN_POINT('Ctrl Pts',(-0.113626032440148,-0.0119580004554367,
-0.971556070349933));
#42737=CARTESIAN_POINT('Ctrl Pts',(-0.0516074088528242,-0.101934019705939,
-0.965207180005287));
#42738=CARTESIAN_POINT('Ctrl Pts',(0.0576229150197905,-0.0986583432173273,
-0.958858289660643));
#42739=CARTESIAN_POINT('Ctrl Pts',(0.114138408711896,-0.00512763872200404,
-0.952509399315997));
#42740=CARTESIAN_POINT('Ctrl Pts',(0.0662373377284729,0.0930939531474212,
-0.946160508971352));
#42741=CARTESIAN_POINT('Ctrl Pts',(-0.0422592447626037,0.106150955031313,
-0.939811618626706));
#42742=CARTESIAN_POINT('Ctrl Pts',(-0.112096052568544,0.0220985072022432,
-0.933462728282062));
#42743=CARTESIAN_POINT('Ctrl Pts',(-0.0793846922795672,-0.0821701871341873,
-0.927113837937415));
#42744=CARTESIAN_POINT('Ctrl Pts',(0.0259496960417602,-0.111267615671996,
-0.920764947592771));
#42745=CARTESIAN_POINT('Ctrl Pts',(0.107544677571258,-0.0385747501364792,
-0.914416057248124));
#42746=CARTESIAN_POINT('Ctrl Pts',(0.0907551984479919,0.0694072256804634,
-0.908067166903481));
#42747=CARTESIAN_POINT('Ctrl Pts',(-0.00905932154553617,0.113893800161064,
-0.901718276558834));
#42748=CARTESIAN_POINT('Ctrl Pts',(-0.10058615604626,0.0541875837607848,
-0.895369386214191));
#42749=CARTESIAN_POINT('Ctrl Pts',(-0.100094352942304,-0.0550907390679732,
-0.889020495869543));
#42750=CARTESIAN_POINT('Ctrl Pts',(-0.00803382555549734,-0.113970727245806,
-0.8826716055249));
#42751=CARTESIAN_POINT('Ctrl Pts',(0.0913762388991208,-0.0685875497932755,
-0.876322715180253));
#42752=CARTESIAN_POINT('Ctrl Pts',(0.10719311972448,0.0395411697566919,
-0.86997382483561));
#42753=CARTESIAN_POINT('Ctrl Pts',(0.0249471534806576,0.111496675085882,
-0.863624934490962));
#42754=CARTESIAN_POINT('Ctrl Pts',(-0.0801210694795765,0.08145233727428,
-0.857276044146319));
#42755=CARTESIAN_POINT('Ctrl Pts',(-0.111892608813196,-0.0231065599986507,
-0.850927153801672));
#42756=CARTESIAN_POINT('Ctrl Pts',(-0.0413020952984331,-0.106527019792883,
-0.844578263457028));
#42757=CARTESIAN_POINT('Ctrl Pts',(0.0670725695247095,-0.0924939967746403,
-0.838229373112382));
#42758=CARTESIAN_POINT('Ctrl Pts',(0.114087632679905,0.00615476169231666,
-0.831880482767737));
#42759=CARTESIAN_POINT('Ctrl Pts',(0.0567325822986109,0.0991729959602187,
-0.825531592423091));
#42760=CARTESIAN_POINT('Ctrl Pts',(-0.0525228004555824,0.101465385498195,
-0.819182702078447));
#42761=CARTESIAN_POINT('Ctrl Pts',(-0.113729060635869,0.0109347971575568,
-0.8128338117338));
#42762=CARTESIAN_POINT('Ctrl Pts',(-0.0708932376197477,-0.0895992069260895,
-0.806484921389157));
#42763=CARTESIAN_POINT('Ctrl Pts',(0.0367974262370298,-0.108165699019257,
-0.80013603104451));
#42764=CARTESIAN_POINT('Ctrl Pts',(0.110824918512494,-0.027779605085262,
-0.793787140699865));
#42765=CARTESIAN_POINT('Ctrl Pts',(0.0834671067359925,0.0780199404967516,
-0.78743825035522));
#42766=CARTESIAN_POINT('Ctrl Pts',(-0.0202484241198383,0.112444965839549,
-0.781089360010574));
#42767=CARTESIAN_POINT('Ctrl Pts',(-0.105440209021084,0.0440026288258347,
-0.77474046966593));
#42768=CARTESIAN_POINT('Ctrl Pts',(-0.0941727517736408,-0.0646943725943335,
-0.768391579321284));
#42769=CARTESIAN_POINT('Ctrl Pts',(0.00324620641900389,-0.114207404164001,
-0.762042688976639));
#42770=CARTESIAN_POINT('Ctrl Pts',(0.0976954568128644,-0.0592407523595027,
-0.755693798631993));
#42771=CARTESIAN_POINT('Ctrl Pts',(0.102770550867044,0.0499207661848099,
-0.749344908287349));
#42772=CARTESIAN_POINT('Ctrl Pts',(0.0138286703355967,0.113413565761524,
-0.742996017942703));
#42773=CARTESIAN_POINT('Ctrl Pts',(-0.0877640108048387,0.0731529044498054,
-0.736647127598058));
#42774=CARTESIAN_POINT('Ctrl Pts',(-0.109068061556924,-0.0340297953301104,
-0.730298237253412));
#42775=CARTESIAN_POINT('Ctrl Pts',(-0.0305940233040475,-0.110081218925235,
-0.723949346908768));
#42776=CARTESIAN_POINT('Ctrl Pts',(0.0758681641528745,-0.0854276927586528,
-0.717600456564121));
#42777=CARTESIAN_POINT('Ctrl Pts',(0.112924328183426,0.0173771437905098,
-0.711251566219477));
#42778=CARTESIAN_POINT('Ctrl Pts',(0.046674597642533,0.104284950769043,
-0.704902675874831));
#42779=CARTESIAN_POINT('Ctrl Pts',(-0.0622741787177168,0.0957903736657717,
-0.698553785530186));
#42780=CARTESIAN_POINT('Ctrl Pts',(-0.114253036862592,-0.000335543840976016,
-0.692204895185541));
#42781=CARTESIAN_POINT('Ctrl Pts',(-0.061710465741824,-0.0961544977623059,
-0.685856004840896));
#42782=CARTESIAN_POINT('Ctrl Pts',(0.0472863253901056,-0.104009001788765,
-0.67950711449625));
#42783=CARTESIAN_POINT('Ctrl Pts',(0.113024447429166,-0.0167135665052596,
-0.673158224151605));
#42784=CARTESIAN_POINT('Ctrl Pts',(0.0753650833999685,0.0858718418697883,
-0.666809333806959));
#42785=CARTESIAN_POINT('Ctrl Pts',(-0.0312400736689609,0.10989962156055,
-0.660460443462316));
#42786=CARTESIAN_POINT('Ctrl Pts',(-0.109266059103523,0.0333885811315727,
-0.654111553117668));
#42787=CARTESIAN_POINT('Ctrl Pts',(-0.0873328226098335,-0.0736671372933253,
-0.647762662773025));
#42788=CARTESIAN_POINT('Ctrl Pts',(0.0144945829286659,-0.113330384662359,
-0.641413772428378));
#42789=CARTESIAN_POINT('Ctrl Pts',(0.103061994983266,-0.0493162672154266,
-0.635064882083734));
#42790=CARTESIAN_POINT('Ctrl Pts',(0.0973458123569227,0.0598135589859446,
-0.628715991739088));
#42791=CARTESIAN_POINT('Ctrl Pts',(0.00257533655841932,0.114224501152796,
-0.622367101394443));
#42792=CARTESIAN_POINT('Ctrl Pts',(-0.0945511191362657,0.0641401192084473,
-0.616018211049797));
#42793=CARTESIAN_POINT('Ctrl Pts',(-0.105179934311565,-0.0446211882429091,
-0.609669320705153));
#42794=CARTESIAN_POINT('Ctrl Pts',(-0.0195876129096983,-0.112561958238536,
-0.603320430360507));
#42795=CARTESIAN_POINT('Ctrl Pts',(0.0839239284397834,-0.0775283384139518,
-0.596971540015862));
#42796=CARTESIAN_POINT('Ctrl Pts',(0.11065983921532,0.028430072227023,-0.590622649671217));
#42797=CARTESIAN_POINT('Ctrl Pts',(0.0361614644549543,0.108379968215843,
-0.58427375932657));
#42798=CARTESIAN_POINT('Ctrl Pts',(-0.0714182887349078,0.0891812595569921,
-0.577924868981927));
#42799=CARTESIAN_POINT('Ctrl Pts',(-0.113662871681053,-0.0116026127751691,
-0.57157597863728));
#42800=CARTESIAN_POINT('Ctrl Pts',(-0.051925922680446,-0.101772135556735,
-0.565227088292636));
#42801=CARTESIAN_POINT('Ctrl Pts',(0.057314110732919,-0.09883805811978,
-0.55887819794799));
#42802=CARTESIAN_POINT('Ctrl Pts',(0.114121815558828,-0.00548454515443092,
-0.552529307603345));
#42803=CARTESIAN_POINT('Ctrl Pts',(0.0665281355275057,0.0928863617827071,
-0.546180417258698));
#42804=CARTESIAN_POINT('Ctrl Pts',(-0.041927084841482,0.106282588313841,
-0.539831526914056));
#42805=CARTESIAN_POINT('Ctrl Pts',(-0.11202639841874,0.0224489438352882,
-0.533482636569408));
#42806=CARTESIAN_POINT('Ctrl Pts',(-0.0796412651948913,-0.0819215350207207,
-0.527133746224765));
#42807=CARTESIAN_POINT('Ctrl Pts',(0.0256016151425451,-0.11134822101896,
-0.520784855880118));
#42808=CARTESIAN_POINT('Ctrl Pts',(0.107423521476236,-0.0389108732315119,
-0.514435965535474));
#42809=CARTESIAN_POINT('Ctrl Pts',(0.0909718036703051,0.0691230783383215,
-0.508087075190828));
#42810=CARTESIAN_POINT('Ctrl Pts',(-0.0087031106790096,0.113921573402508,
-0.501738184846182));
#42811=CARTESIAN_POINT('Ctrl Pts',(-0.100416209813545,0.0545018699557744,
-0.495389294501538));
#42812=CARTESIAN_POINT('Ctrl Pts',(-0.100266142249298,-0.0547774564984331,
-0.489040404156892));
#42813=CARTESIAN_POINT('Ctrl Pts',(-0.00839019340757563,-0.113945046739986,
-0.482691513812247));
#42814=CARTESIAN_POINT('Ctrl Pts',(0.0911613063941586,-0.06887296449627,
-0.476342623467602));
#42815=CARTESIAN_POINT('Ctrl Pts',(0.107316247997619,0.0392057640877946,
-0.469993733122956));
#42816=CARTESIAN_POINT('Ctrl Pts',(0.0252957018227751,0.111418115633354,
-0.463644842778311));
#42817=CARTESIAN_POINT('Ctrl Pts',(-0.0798659614846814,0.0817024921169577,
-0.457295952433666));
#42818=CARTESIAN_POINT('Ctrl Pts',(-0.111964320102099,-0.022756538534425,
-0.450947062089021));
#42819=CARTESIAN_POINT('Ctrl Pts',(-0.0416350226572824,-0.106397339770888,
-0.444598171744375));
#42820=CARTESIAN_POINT('Ctrl Pts',(0.0667829960604789,-0.0927032926016133,
-0.43824928139973));
#42821=CARTESIAN_POINT('Ctrl Pts',(0.114106321888124,0.00579795887860732,
-0.431900391055085));
#42822=CARTESIAN_POINT('Ctrl Pts',(0.0570424368415761,0.0989950979653487,
-0.425551500710439));
#42823=CARTESIAN_POINT('Ctrl Pts',(-0.0522052429748849,0.101629137691547,
-0.419202610365795));
#42824=CARTESIAN_POINT('Ctrl Pts',(-0.113694309447372,0.0112903950895989,
-0.412853720021149));
#42825=CARTESIAN_POINT('Ctrl Pts',(-0.071173083947476,-0.0893770728061716,
-0.406504829676504));
#42826=CARTESIAN_POINT('Ctrl Pts',(0.036458992552212,-0.10828024235322,
-0.400155939331858));
#42827=CARTESIAN_POINT('Ctrl Pts',(0.110737504754736,-0.0281260388730614,
-0.393807048987213));
#42828=CARTESIAN_POINT('Ctrl Pts',(0.0837106811157609,0.0777585422261086,
-0.387458158642568));
#42829=CARTESIAN_POINT('Ctrl Pts',(-0.0198966893102775,0.112507736518359,
-0.381109268297923));
#42830=CARTESIAN_POINT('Ctrl Pts',(-0.105302089255079,0.0443321443256423,
-0.374760377953277));
#42831=CARTESIAN_POINT('Ctrl Pts',(-0.0943746023389721,-0.0643995609872857,
-0.368411487608632));
#42832=CARTESIAN_POINT('Ctrl Pts',(0.00288904327994013,-0.114216997206724,
-0.362062597263987));
#42833=CARTESIAN_POINT('Ctrl Pts',(0.0975097225399547,-0.0595459741055193,
-0.355713706919342));
#42834=CARTESIAN_POINT('Ctrl Pts',(0.102926159645516,0.0495991399383105,
-0.349364816574696));
#42835=CARTESIAN_POINT('Ctrl Pts',(0.0141832675079377,0.113369766449404,
-0.343015926230051));
#42836=CARTESIAN_POINT('Ctrl Pts',(-0.0875348192703691,0.0734270007374531,
-0.336667035885406));
#42837=CARTESIAN_POINT('Ctrl Pts',(-0.109173945594853,-0.0336885533267078,
-0.33031814554076));
#42838=CARTESIAN_POINT('Ctrl Pts',(-0.0309381176468522,-0.10998500760769,
-0.323969255196116));
#42839=CARTESIAN_POINT('Ctrl Pts',(0.0756006452955727,-0.0856645285569653,
-0.31762036485147));
#42840=CARTESIAN_POINT('Ctrl Pts',(0.11297811750398,0.0170239239674976,
-0.311271474506825));
#42841=CARTESIAN_POINT('Ctrl Pts',(0.0470004873752844,0.104138480920743,
-0.304922584162179));
#42842=CARTESIAN_POINT('Ctrl Pts',(-0.0619743203475146,0.0959846479363122,
-0.298573693817534));
#42843=CARTESIAN_POINT('Ctrl Pts',(-0.114253527512409,2.17477677095862E-5,
-0.292224803472889));
#42844=CARTESIAN_POINT('Ctrl Pts',(-0.0620108565533915,-0.0959610477824666,
-0.285875913128243));
#42845=CARTESIAN_POINT('Ctrl Pts',(0.0469608391644364,-0.104156366137486,
-0.279527022783599));
#42846=CARTESIAN_POINT('Ctrl Pts',(0.11297162842615,-0.0170669327278882,
-0.273178132438953));
#42847=CARTESIAN_POINT('Ctrl Pts',(0.0756332517154119,0.0856357417025584,
-0.266829242094308));
#42848=CARTESIAN_POINT('Ctrl Pts',(-0.0308962448673541,0.109996777566847,
-0.260480351749662));
#42849=CARTESIAN_POINT('Ctrl Pts',(-0.109161112682653,0.0337301126573813,
-0.254131461405017));
#42850=CARTESIAN_POINT('Ctrl Pts',(-0.0875627660825531,-0.0733936715116903,
-0.247782571060372));
#42851=CARTESIAN_POINT('Ctrl Pts',(0.0141401073880872,-0.113375157706821,
-0.241433680715727));
#42852=CARTESIAN_POINT('Ctrl Pts',(0.102907270134931,-0.049638319626816,
-0.235084790371081));
#42853=CARTESIAN_POINT('Ctrl Pts',(0.0975323842177206,0.0595088485084162,
-0.228735900026436));
#42854=CARTESIAN_POINT('Ctrl Pts',(0.00293252469764535,0.114215889091171,
-0.222387009681791));
#42855=CARTESIAN_POINT('Ctrl Pts',(-0.0943500790294188,0.0644354840841576,
-0.216038119337145));
#42856=CARTESIAN_POINT('Ctrl Pts',(-0.105318958567443,-0.0442920533305308,
-0.2096892289925));
#42857=CARTESIAN_POINT('Ctrl Pts',(-0.0199395187920133,-0.112500153832397,
-0.203340338647855));
#42858=CARTESIAN_POINT('Ctrl Pts',(0.0836810729070069,-0.0777904046735807,
-0.196991448303209));
#42859=CARTESIAN_POINT('Ctrl Pts',(0.110748204119093,0.0280838798274333,
-0.190642557958565));
#42860=CARTESIAN_POINT('Ctrl Pts',(0.036500211457678,0.10826635481745,-0.184293667613919));
#42861=CARTESIAN_POINT('Ctrl Pts',(-0.0711390535560091,0.0894041614363504,
-0.177944777269274));
#42862=CARTESIAN_POINT('Ctrl Pts',(-0.11369859937654,-0.0112471116321533,
-0.171595886924628));
#42863=CARTESIAN_POINT('Ctrl Pts',(-0.0522439287224621,-0.101609256141691,
-0.165246996579984));
#42864=CARTESIAN_POINT('Ctrl Pts',(0.0570047459826288,-0.0990168064706588,
-0.158898106235338));
#42865=CARTESIAN_POINT('Ctrl Pts',(0.114104106321442,-0.00584139792443139,
-0.152549215890693));
#42866=CARTESIAN_POINT('Ctrl Pts',(0.0668182828326907,0.0926778620031539,
-0.146200325546047));
#42867=CARTESIAN_POINT('Ctrl Pts',(-0.0415945151008719,0.106413182328006,
-0.139851435201403));
#42868=CARTESIAN_POINT('Ctrl Pts',(-0.111955648355773,0.0227991607446998,
-0.133502544856757));
#42869=CARTESIAN_POINT('Ctrl Pts',(-0.079897059986415,-0.0816720814146227,
-0.127153654512112));
#42870=CARTESIAN_POINT('Ctrl Pts',(0.0252532852262649,-0.111427738139436,
-0.120804764167466));
#42871=CARTESIAN_POINT('Ctrl Pts',(0.107301312298338,-0.0392466145167992,
-0.114455873822821));
#42872=CARTESIAN_POINT('Ctrl Pts',(0.0911875241033174,0.0688382525769072,
-0.108106983478176));
#42873=CARTESIAN_POINT('Ctrl Pts',(-0.00834682390039813,0.113948237208761,
-0.101758093133531));
#42874=CARTESIAN_POINT('Ctrl Pts',(-0.10024526413777,0.0548156143681033,
-0.0954092027888852));
#42875=CARTESIAN_POINT('Ctrl Pts',(-0.100436984107331,-0.0544636215682244,
-0.0890603124442403));
#42876=CARTESIAN_POINT('Ctrl Pts',(-0.00874641646927006,-0.113918283558929,
-0.0827114220995946));
#42877=CARTESIAN_POINT('Ctrl Pts',(0.0909453634107706,-0.0691576456924166,
-0.0763625317549498));
#42878=CARTESIAN_POINT('Ctrl Pts',(0.10743855244889,0.0388698612665832,
-0.0700136414103045));
#42879=CARTESIAN_POINT('Ctrl Pts',(0.0256435748410253,0.111338682311979,
-0.0636647510656591));
#42880=CARTESIAN_POINT('Ctrl Pts',(-0.0796092608576849,0.0819514388563111,
-0.0573158607210139));
#42881=CARTESIAN_POINT('Ctrl Pts',(-0.112036475647968,-0.0224055186530005,
-0.0509669703763686));
#42882=CARTESIAN_POINT('Ctrl Pts',(-0.0419646237851041,-0.106268090710258,
-0.0446180800317233));
#42883=CARTESIAN_POINT('Ctrl Pts',(0.066487233315796,-0.0929088911131196,
-0.0382691896870782));
#42884=CARTESIAN_POINT('Ctrl Pts',(0.114134396399028,0.00543580541106296,
-0.0319202993424328));
#42885=CARTESIAN_POINT('Ctrl Pts',(0.0573318023082725,0.0988262831913889,
-0.0255714089977875));
#42886=CARTESIAN_POINT('Ctrl Pts',(-0.0518492415773505,0.101772737650102,
-0.0192225186531422));
#42887=CARTESIAN_POINT('Ctrl Pts',(-0.113731515237727,0.0116830253251869,
-0.0128736283084969));
#42888=CARTESIAN_POINT('Ctrl Pts',(-0.0713041863188721,-0.0892312379820752,
-0.00652473796385158));
#42889=CARTESIAN_POINT('Ctrl Pts',(7.37734688490074E-5,-0.101876700685701,
-0.0022921444007548));
#42890=CARTESIAN_POINT('Ctrl Pts',(0.0305629119072589,-0.091716759868353,
-0.000175847619206415));
#42891=CARTESIAN_POINT('Ctrl Pts',(-0.0967093838725941,-8.47898118814713E-5,
-0.0522235916889671));
#42892=CARTESIAN_POINT('Ctrl Pts',(-0.0967676968424891,-0.00643802185033027,
-0.0518047179181009));
#42893=CARTESIAN_POINT('Ctrl Pts',(-0.096195117326514,-0.0127808110712041,
-0.0513858441472348));
#42894=CARTESIAN_POINT('Ctrl Pts',(-0.0949532978724438,-0.0189897877443241,
-0.0509669703763687));
#42895=CARTESIAN_POINT('Ctrl Pts',(-0.0886791916936804,-0.0503597093387527,
-0.0488506735948202));
#42896=CARTESIAN_POINT('Ctrl Pts',(-0.0653219077393917,-0.0783139000245061,
-0.0467343768132717));
#42897=CARTESIAN_POINT('Ctrl Pts',(-0.0355679562454307,-0.0900644621011926,
-0.0446180800317233));
#42898=CARTESIAN_POINT('Ctrl Pts',(-0.00581400475147052,-0.101815024177879,
-0.0425017832501749));
#42899=CARTESIAN_POINT('Ctrl Pts',(0.0303366142821625,-0.0973619576454991,
-0.0403854864686265));
#42900=CARTESIAN_POINT('Ctrl Pts',(0.056353117646184,-0.0787446416252796,
-0.0382691896870782));
#42901=CARTESIAN_POINT('Ctrl Pts',(0.0823696210102062,-0.0601273256050595,
-0.0361528929055297));
#42902=CARTESIAN_POINT('Ctrl Pts',(0.0982520087046172,-0.0273457600969982,
-0.0340365961239812));
#42903=CARTESIAN_POINT('Ctrl Pts',(0.0967261035366966,0.00461010228708682,
-0.0319202993424328));
#42904=CARTESIAN_POINT('Ctrl Pts',(0.095200198368776,0.0365659646711728,
-0.0298040025608842));
#42905=CARTESIAN_POINT('Ctrl Pts',(0.0762660003385246,0.0676961239312805,
-0.0276877057793359));
#42906=CARTESIAN_POINT('Ctrl Pts',(0.0486020606757939,0.0837522793044539,
-0.0255714089977874));
#42907=CARTESIAN_POINT('Ctrl Pts',(0.0209381210130655,0.0998084346776261,
-0.0234551122162391));
#42908=CARTESIAN_POINT('Ctrl Pts',(-0.0154555602821406,0.100790586163864,
-0.0213388154346908));
#42909=CARTESIAN_POINT('Ctrl Pts',(-0.0439661132064728,0.0862667098528324,
-0.0192225186531425));
#42910=CARTESIAN_POINT('Ctrl Pts',(-0.0704497203496431,0.0727754024257818,
-0.0172566791020951));
#42911=CARTESIAN_POINT('Ctrl Pts',(-0.0901312497269368,0.0459044819879136,
-0.0152908395510477));
#42912=CARTESIAN_POINT('Ctrl Pts',(-0.0953948120465076,0.0166363274765985,
-0.0133250000000003));
#42913=CARTESIAN_POINT('',(-0.0601936375465013,0.0430788095790887,-1.149325));
#42914=CARTESIAN_POINT('Ctrl Pts',(-0.0601945574557614,0.0430798164930455,
-1.149325));
#42915=CARTESIAN_POINT('Ctrl Pts',(-0.0593969414063664,0.0446614288629473,
-1.149325));
#42916=CARTESIAN_POINT('Ctrl Pts',(-0.0585400474987182,0.0462093080774674,
-1.149325));
#42917=CARTESIAN_POINT('Ctrl Pts',(-0.057624700283891,0.0477197559654082,
-1.149325));
#42918=CARTESIAN_POINT('Ctrl Pts',(-0.0555316807570405,0.0511735239700963,
-1.149325));
#42919=CARTESIAN_POINT('Ctrl Pts',(-0.0531337632154356,0.0544318108953775,
-1.149325));
#42920=CARTESIAN_POINT('Ctrl Pts',(-0.0504744945711353,0.057482955786154,
-1.149325));
#42921=CARTESIAN_POINT('Ctrl Pts',(-0.0486009492640357,0.0596325912521487,
-1.149325));
#42922=CARTESIAN_POINT('Ctrl Pts',(-0.0465971933153744,0.061678830173069,
-1.149325));
#42923=CARTESIAN_POINT('Ctrl Pts',(-0.0444878921416535,0.0636076850959539,
-1.149325));
#42924=CARTESIAN_POINT('Ctrl Pts',(-0.0415466589643101,0.0662973020004301,
-1.149325));
#42925=CARTESIAN_POINT('Ctrl Pts',(-0.0383961696174096,0.0687641338366335,
-1.149325));
#42926=CARTESIAN_POINT('Ctrl Pts',(-0.0350729886334158,0.0709963287796745,
-1.149325));
#42927=CARTESIAN_POINT('Ctrl Pts',(-0.0327258042152802,0.0725729426366335,
-1.149325));
#42928=CARTESIAN_POINT('Ctrl Pts',(-0.0302911492173328,0.0740325115864712,
-1.149325));
#42929=CARTESIAN_POINT('Ctrl Pts',(-0.0277962837734336,0.0753625431214874,
-1.149325));
#42930=CARTESIAN_POINT('Ctrl Pts',(-0.0218327884651418,0.0785417273289343,
-1.149325));
#42931=CARTESIAN_POINT('Ctrl Pts',(-0.0155102394754001,0.0809963000056631,
-1.149325));
#42932=CARTESIAN_POINT('Ctrl Pts',(-0.0089852668252898,0.0826657982356903,
-1.149325));
#42933=CARTESIAN_POINT('Ctrl Pts',(-0.00663553819203132,0.0832670065479126,
-1.149325));
#42934=CARTESIAN_POINT('Ctrl Pts',(-0.00425676076600993,0.0837664401122449,
-1.149325));
#42935=CARTESIAN_POINT('Ctrl Pts',(-0.00186339920018093,0.0841586454601682,
-1.149325));
#42936=CARTESIAN_POINT('Ctrl Pts',(0.00212334881951441,0.0848119625002976,
-1.149325));
#42937=CARTESIAN_POINT('Ctrl Pts',(0.00613700862087291,0.0851664111597531,
-1.149325));
#42938=CARTESIAN_POINT('Ctrl Pts',(0.0101454841298669,0.0852107399416391,
-1.149325));
#42939=CARTESIAN_POINT('Ctrl Pts',(0.0153704726303765,0.0852685218527613,
-1.149325));
#42940=CARTESIAN_POINT('Ctrl Pts',(0.0205868041004565,0.0848003053162965,
-1.149325));
#42941=CARTESIAN_POINT('Ctrl Pts',(0.0257427285955276,0.0838507664789196,
-1.149325));
#42942=CARTESIAN_POINT('Ctrl Pts',(0.0288674016778731,0.0832753122711186,
-1.149325));
#42943=CARTESIAN_POINT('Ctrl Pts',(0.0319730906513826,0.0825211692425999,
-1.149325));
#42944=CARTESIAN_POINT('Ctrl Pts',(0.0350236518943335,0.0816043220267138,
-1.149325));
#42945=CARTESIAN_POINT('Ctrl Pts',(0.040291699894543,0.0800210084140771,
-1.149325));
#42946=CARTESIAN_POINT('Ctrl Pts',(0.0454099142546439,0.0779519494185946,
-1.149325));
#42947=CARTESIAN_POINT('Ctrl Pts',(0.050321493373422,0.0754465004076252,
-1.149325));
#42948=CARTESIAN_POINT('Ctrl Pts',(0.0539221601041848,0.073609761818822,
-1.149325));
#42949=CARTESIAN_POINT('Ctrl Pts',(0.057411918207577,0.0715380616425189,
-1.149325));
#42950=CARTESIAN_POINT('Ctrl Pts',(0.0607676654134175,0.0692448068755771,
-1.149325));
#42951=CARTESIAN_POINT('Ctrl Pts',(0.0631311994125498,0.0676296120239192,
-1.149325));
#42952=CARTESIAN_POINT('Ctrl Pts',(0.0654216850985366,0.0659085707891866,
-1.149325));
#42953=CARTESIAN_POINT('Ctrl Pts',(0.0676254903620251,0.0640927368991582,
-1.149325));
#42954=CARTESIAN_POINT('Ctrl Pts',(0.0734188261013449,0.0593192954585486,
-1.149325));
#42955=CARTESIAN_POINT('Ctrl Pts',(0.0786285494123232,0.0538847809587341,
-1.149325));
#42956=CARTESIAN_POINT('Ctrl Pts',(0.0831143226909517,0.0478769911187842,
-1.149325));
#42957=CARTESIAN_POINT('Ctrl Pts',(0.0844138435846824,0.0461365446144203,
-1.149325));
#42958=CARTESIAN_POINT('Ctrl Pts',(0.0856524500666806,0.0443476946186774,
-1.149325));
#42959=CARTESIAN_POINT('Ctrl Pts',(0.0868262223680489,0.042511912851507,
-1.149325));
#42960=CARTESIAN_POINT('Ctrl Pts',(-0.0601945574557609,0.0430798164930462,
-1.149325));
#42961=CARTESIAN_POINT('Ctrl Pts',(-0.0689950045553977,0.0306449443926568,
-1.14800758135659));
#42962=CARTESIAN_POINT('Ctrl Pts',(-0.0737382340313444,0.0152576839591632,
-1.14669016271317));
#42963=CARTESIAN_POINT('Ctrl Pts',(-0.0738510899558415,-6.10647340483529E-5,
-1.14537274406976));
#42964=CARTESIAN_POINT('Origin',(-2.39206768658147E-17,-5.43753587379397E-18,
-1.149325));
#42965=CARTESIAN_POINT('Ctrl Pts',(0.086954608065376,-0.0426125957048272,
-1.149325));
#42966=CARTESIAN_POINT('Ctrl Pts',(0.0857330349750578,-0.0445411053039618,
-1.149325));
#42967=CARTESIAN_POINT('Ctrl Pts',(0.0844400486091011,-0.0464202818838494,
-1.149325));
#42968=CARTESIAN_POINT('Ctrl Pts',(0.0830754117572655,-0.0482455415151559,
-1.149325));
#42969=CARTESIAN_POINT('Ctrl Pts',(0.0800390864492769,-0.0523067553133409,
-1.149325));
#42970=CARTESIAN_POINT('Ctrl Pts',(0.0766483379746834,-0.0561016838993785,
-1.149325));
#42971=CARTESIAN_POINT('Ctrl Pts',(0.0729515424226022,-0.059605136564689,
-1.149325));
#42972=CARTESIAN_POINT('Ctrl Pts',(0.070603271984809,-0.0618305921540642,
-1.149325));
#42973=CARTESIAN_POINT('Ctrl Pts',(0.0681306233770263,-0.063938250313155,
-1.149325));
#42974=CARTESIAN_POINT('Ctrl Pts',(0.0655584298678572,-0.0659112849073347,
-1.149325));
#42975=CARTESIAN_POINT('Ctrl Pts',(0.061295013787923,-0.0691815938421431,
-1.149325));
#42976=CARTESIAN_POINT('Ctrl Pts',(0.0567507752997466,-0.0720904225810572,
-1.149325));
#42977=CARTESIAN_POINT('Ctrl Pts',(0.0519830713174729,-0.0746026273715568,
-1.149325));
#42978=CARTESIAN_POINT('Ctrl Pts',(0.0495592178451569,-0.0758798073993565,
-1.149325));
#42979=CARTESIAN_POINT('Ctrl Pts',(0.047077602993811,-0.0770537891045191,
-1.149325));
#42980=CARTESIAN_POINT('Ctrl Pts',(0.0445587027673779,-0.0781143696302628,
-1.149325));
#42981=CARTESIAN_POINT('Ctrl Pts',(0.038135306482972,-0.0808189344784,-1.149325));
#42982=CARTESIAN_POINT('Ctrl Pts',(0.031448698113717,-0.0828009884055702,
-1.149325));
#42983=CARTESIAN_POINT('Ctrl Pts',(0.0246280221596509,-0.0839739399799056,
-1.149325));
#42984=CARTESIAN_POINT('Ctrl Pts',(0.0221514627490004,-0.0843998338765254,
-1.149325));
#42985=CARTESIAN_POINT('Ctrl Pts',(0.0196572765175813,-0.0847185915787331,
-1.149325));
#42986=CARTESIAN_POINT('Ctrl Pts',(0.0171520746182129,-0.0849244113167061,
-1.149325));
#42987=CARTESIAN_POINT('Ctrl Pts',(0.0146062307049426,-0.0851335700784337,
-1.149325));
#42988=CARTESIAN_POINT('Ctrl Pts',(0.0120579190174,-0.0852252699062859,
-1.149325));
#42989=CARTESIAN_POINT('Ctrl Pts',(0.00951710917596823,-0.0851952692846318,
-1.149325));
#42990=CARTESIAN_POINT('Ctrl Pts',(0.00767225013911105,-0.0851734861046915,
-1.149325));
#42991=CARTESIAN_POINT('Ctrl Pts',(0.00583076398118415,-0.0850875694335481,
-1.149325));
#42992=CARTESIAN_POINT('Ctrl Pts',(0.00399523787071753,-0.0849356509029418,
-1.149325));
#42993=CARTESIAN_POINT('Ctrl Pts',(-0.000130301487827045,-0.0845941979136682,
-1.149325));
#42994=CARTESIAN_POINT('Ctrl Pts',(-0.0042260125748701,-0.0839196884632143,
-1.149325));
#42995=CARTESIAN_POINT('Ctrl Pts',(-0.00825975656469361,-0.0829293963495848,
-1.149325));
#42996=CARTESIAN_POINT('Ctrl Pts',(-0.0108453319126542,-0.0822946324967623,
-1.149325));
#42997=CARTESIAN_POINT('Ctrl Pts',(-0.0134073686845953,-0.0815292810894073,
-1.149325));
#42998=CARTESIAN_POINT('Ctrl Pts',(-0.0159300211431115,-0.0806390832814289,
-1.149325));
#42999=CARTESIAN_POINT('Ctrl Pts',(-0.0221589550044849,-0.0784410067090031,
-1.149325));
#43000=CARTESIAN_POINT('Ctrl Pts',(-0.0281034482611466,-0.075502483957626,
-1.149325));
#43001=CARTESIAN_POINT('Ctrl Pts',(-0.0336303034371419,-0.0718981146415137,
-1.149325));
#43002=CARTESIAN_POINT('Ctrl Pts',(-0.0361277442859076,-0.070269394713553,
-1.149325));
#43003=CARTESIAN_POINT('Ctrl Pts',(-0.0385394333564065,-0.0685042094556212,
-1.149325));
#43004=CARTESIAN_POINT('Ctrl Pts',(-0.0408500806194884,-0.0666075686697806,
-1.149325));
#43005=CARTESIAN_POINT('Ctrl Pts',(-0.0424803759150722,-0.0652693788906776,
-1.149325));
#43006=CARTESIAN_POINT('Ctrl Pts',(-0.0440585000802111,-0.063866941402308,
-1.149325));
#43007=CARTESIAN_POINT('Ctrl Pts',(-0.0455732185102893,-0.06240842283285,
-1.149325));
#43008=CARTESIAN_POINT('Ctrl Pts',(-0.0499785755932977,-0.0581665155693797,
-1.149325));
#43009=CARTESIAN_POINT('Ctrl Pts',(-0.053867914455048,-0.053437905398849,
-1.149325));
#43010=CARTESIAN_POINT('Ctrl Pts',(-0.0571076045136135,-0.0482724182734906,
-1.149325));
#43011=CARTESIAN_POINT('Ctrl Pts',(-0.058182525399877,-0.0465585228395456,
-1.149325));
#43012=CARTESIAN_POINT('Ctrl Pts',(-0.0591855280879638,-0.0447964220518841,
-1.149325));
#43013=CARTESIAN_POINT('Ctrl Pts',(-0.0601104350279423,-0.042987737795231,
-1.149325));
#43014=CARTESIAN_POINT('Origin',(0.,0.,-1.149325));
#43015=CARTESIAN_POINT('Origin',(0.,0.,-1.25327725593024));
#43016=CARTESIAN_POINT('Ctrl Pts',(-0.0786356739692314,-0.056235988516294,
-1.16247415238079));
#43017=CARTESIAN_POINT('Ctrl Pts',(-0.0599413062053112,-0.0823766192285753,
-1.16035785559925));
#43018=CARTESIAN_POINT('Ctrl Pts',(0.00523751855363567,-0.11410112217152,
-1.15612526203615));
#43019=CARTESIAN_POINT('Ctrl Pts',(0.0988778236354322,-0.0573979516486903,
-1.1497763716915));
#43020=CARTESIAN_POINT('Ctrl Pts',(0.10176744392733,0.0518596603249867,
-1.14342748134686));
#43021=CARTESIAN_POINT('Ctrl Pts',(0.0117062229254556,0.113650929875517,
-1.13707859100221));
#43022=CARTESIAN_POINT('Ctrl Pts',(-0.0891415772947104,0.071484176152418,
-1.13072970065757));
#43023=CARTESIAN_POINT('Ctrl Pts',(-0.108399781825892,-0.0360846577190267,
-1.12438081031292));
#43024=CARTESIAN_POINT('Ctrl Pts',(-0.0285127216364505,-0.110638879749571,
-1.11803191996828));
#43025=CARTESIAN_POINT('Ctrl Pts',(0.077469779648326,-0.0839798348596053,
-1.11168302962363));
#43026=CARTESIAN_POINT('Ctrl Pts',(0.112575094334631,0.0195069576219953,
-1.10533413927899));
#43027=CARTESIAN_POINT('Ctrl Pts',(0.0446971480117591,0.105147802803276,
-1.09898524893434));
#43028=CARTESIAN_POINT('Ctrl Pts',(-0.0640724843747248,0.0945971764401096,
-1.0926363585897));
#43029=CARTESIAN_POINT('Ctrl Pts',(-0.114226190614228,-0.00249336732137551,
-1.08628746824505));
#43030=CARTESIAN_POINT('Ctrl Pts',(-0.0598834883344679,-0.0973028434580084,
-1.0799385779004));
#43031=CARTESIAN_POINT('Ctrl Pts',(0.0492423141801099,-0.103097375035228,
-1.07358968755576));
#43032=CARTESIAN_POINT('Ctrl Pts',(0.113319933754507,-0.0145759245129412,
-1.06724079721111));
#43033=CARTESIAN_POINT('Ctrl Pts',(0.0737298168519105,0.0872799217159805,
-1.06089190686647));
#43034=CARTESIAN_POINT('Ctrl Pts',(-0.0333101475173397,0.109289999720582,
-1.05454301652182));
#43035=CARTESIAN_POINT('Ctrl Pts',(-0.109877168057254,0.0313189512811141,
-1.04819412617718));
#43036=CARTESIAN_POINT('Ctrl Pts',(-0.0859259193914243,-0.0753034263167131,
-1.04184523583253));
#43037=CARTESIAN_POINT('Ctrl Pts',(0.0166324346020325,-0.11303641711073,
-1.03549634548789));
#43038=CARTESIAN_POINT('Ctrl Pts',(0.103975034167995,-0.047360971234609,
-1.02914745514324));
#43039=CARTESIAN_POINT('Ctrl Pts',(0.0961987702738092,0.0616414313136374,
-1.0227985647986));
#43040=CARTESIAN_POINT('Ctrl Pts',(0.000417554159368378,0.114252768332749,
-1.01644967445395));
#43041=CARTESIAN_POINT('Ctrl Pts',(-0.0957456501507325,0.0623429216779739,
-1.01010078410931));
#43042=CARTESIAN_POINT('Ctrl Pts',(-0.10431842841873,-0.0465997308728082,
-1.00375189376466));
#43043=CARTESIAN_POINT('Ctrl Pts',(-0.017458196332613,-0.11291182754622,
-0.997403003420017));
#43044=CARTESIAN_POINT('Ctrl Pts',(0.0853732140821567,-0.0759294655224641,
-0.991054113075372));
#43045=CARTESIAN_POINT('Ctrl Pts',(0.110103152550627,0.030514999891575,
-0.984705222730726));
#43046=CARTESIAN_POINT('Ctrl Pts',(0.0341080758322783,0.109043608624817,
-0.978356332386081));
#43047=CARTESIAN_POINT('Ctrl Pts',(-0.073089889950516,0.0878164984827856,
-0.972007442041436));
#43048=CARTESIAN_POINT('Ctrl Pts',(-0.113423464450988,-0.0137472590385073,
-0.96565855169679));
#43049=CARTESIAN_POINT('Ctrl Pts',(-0.0499945225011397,-0.102734692966118,
-0.959309661352146));
#43050=CARTESIAN_POINT('Ctrl Pts',(0.0591706124692214,-0.0977379559790979,
-0.952960771007499));
#43051=CARTESIAN_POINT('Ctrl Pts',(0.114205046360993,-0.00332818339188197,
-0.946611880662856));
#43052=CARTESIAN_POINT('Ctrl Pts',(0.0647619538532123,0.09412629150292,
-0.940262990318209));
#43053=CARTESIAN_POINT('Ctrl Pts',(-0.0439269334678215,0.105471768426881,
-0.933914099973564));
#43054=CARTESIAN_POINT('Ctrl Pts',(-0.112430404318708,0.020329131897814,
-0.927565209628919));
#43055=CARTESIAN_POINT('Ctrl Pts',(-0.0780798340429289,-0.0834110840045326,
-0.921216319284272));
#43056=CARTESIAN_POINT('Ctrl Pts',(0.0277000485302825,-0.110844831771279,
-0.91486742893963));
#43057=CARTESIAN_POINT('Ctrl Pts',(0.108139259707659,-0.0368750583574256,
-0.908518538594982));
#43058=CARTESIAN_POINT('Ctrl Pts',(0.0896500721767574,0.0708289063708139,
-0.902169648250338));
#43059=CARTESIAN_POINT('Ctrl Pts',(-0.0108531601007334,0.113736882033979,
-0.895820757905693));
#43060=CARTESIAN_POINT('Ctrl Pts',(-0.101427660180571,0.0525956192974108,
-0.889471867561047));
#43061=CARTESIAN_POINT('Ctrl Pts',(-0.0992136944107583,-0.0566613824430021,
-0.883122977216402));
#43062=CARTESIAN_POINT('Ctrl Pts',(-0.00623665198847288,-0.114083187152876,
-0.876774086871757));
#43063=CARTESIAN_POINT('Ctrl Pts',(0.0924458298476606,-0.0671389452014324,
-0.870425196527112));
#43064=CARTESIAN_POINT('Ctrl Pts',(0.106556640499711,0.0412256204853105,
-0.864076306182466));
#43065=CARTESIAN_POINT('Ctrl Pts',(0.0231868706034319,0.111875995864185,
-0.857727415837821));
#43066=CARTESIAN_POINT('Ctrl Pts',(-0.0813948068466306,0.0801795163204622,
-0.851378525493176));
#43067=CARTESIAN_POINT('Ctrl Pts',(-0.111514555055875,-0.0248671154272822,
-0.845029635148529));
#43068=CARTESIAN_POINT('Ctrl Pts',(-0.039618103097239,-0.10716471119711,
-0.838680744803886));
#43069=CARTESIAN_POINT('Ctrl Pts',(0.0685219435546145,-0.0914254487026546,
-0.832331854459239));
#43070=CARTESIAN_POINT('Ctrl Pts',(0.113976466275917,0.00795201573427383,
-0.825982964114595));
#43071=CARTESIAN_POINT('Ctrl Pts',(0.0551625731639185,0.100054784697779,
-0.819634073769949));
#43072=CARTESIAN_POINT('Ctrl Pts',(-0.0541153701596963,0.100625027361301,
-0.813285183425305));
#43073=CARTESIAN_POINT('Ctrl Pts',(-0.113887269795971,0.00914107200515301,
-0.806936293080658));
#43074=CARTESIAN_POINT('Ctrl Pts',(-0.0694723526865942,-0.0907053561327721,
-0.800587402736014));
#43075=CARTESIAN_POINT('Ctrl Pts',(0.0384975455125421,-0.107572340350544,
-0.794238512391367));
#43076=CARTESIAN_POINT('Ctrl Pts',(0.111248962079288,-0.0260295573390085,
-0.787889622046723));
#43077=CARTESIAN_POINT('Ctrl Pts',(0.0822271493284522,0.0793256915021855,
-0.781540731702078));
#43078=CARTESIAN_POINT('Ctrl Pts',(-0.0220180396078722,0.112111887642701,
-0.775191841357432));
#43079=CARTESIAN_POINT('Ctrl Pts',(-0.106120595729893,0.0423354293815024,
-0.768842951012787));
#43080=CARTESIAN_POINT('Ctrl Pts',(-0.093141475558706,-0.0661704990893252,
-0.762494060668143));
#43081=CARTESIAN_POINT('Ctrl Pts',(0.00504570924375355,-0.114142061647804,
-0.756145170323495));
#43082=CARTESIAN_POINT('Ctrl Pts',(0.0986169577324141,-0.0576937177393419,
-0.749796279978852));
#43083=CARTESIAN_POINT('Ctrl Pts',(0.101971038651006,0.0515342283867572,
-0.743447389634206));
#43084=CARTESIAN_POINT('Ctrl Pts',(0.0120395580109721,0.113617421471727,
-0.73709849928956));
#43085=CARTESIAN_POINT('Ctrl Pts',(-0.0889060002027456,0.0717606615558481,
-0.730749608944917));
#43086=CARTESIAN_POINT('Ctrl Pts',(-0.108518208628496,-0.0357444795044725,
-0.724400718600269));
#43087=CARTESIAN_POINT('Ctrl Pts',(-0.0288553467483356,-0.110549710008741,
-0.718051828255626));
#43088=CARTESIAN_POINT('Ctrl Pts',(0.0772050811564295,-0.0842214038271311,
-0.711702937910979));
#43089=CARTESIAN_POINT('Ctrl Pts',(0.112636441767823,0.019154670575798,
-0.705354047566334));
#43090=CARTESIAN_POINT('Ctrl Pts',(0.0450252732328951,0.105007591103151,
-0.699005157221689));
#43091=CARTESIAN_POINT('Ctrl Pts',(-0.0637760994367215,0.0947970387703165,
-0.692656266877044));
#43092=CARTESIAN_POINT('Ctrl Pts',(-0.114233560651881,-0.00213612728472956,
-0.686307376532398));
#43093=CARTESIAN_POINT('Ctrl Pts',(-0.0601874099079299,-0.0971151126630577,
-0.679958486187754));
#43094=CARTESIAN_POINT('Ctrl Pts',(0.0489196326960759,-0.103250854504282,
-0.673609595843107));
#43095=CARTESIAN_POINT('Ctrl Pts',(0.113273817354663,-0.0149302284271154,
-0.667260705498463));
#43096=CARTESIAN_POINT('Ctrl Pts',(0.0740023863324715,0.0870489301260112,
-0.660911815153817));
#43097=CARTESIAN_POINT('Ctrl Pts',(-0.0329682096391889,0.109393631314487,
-0.654562924809173));
#43098=CARTESIAN_POINT('Ctrl Pts',(-0.109778693578452,0.0316624044442602,
-0.648214034464526));
#43099=CARTESIAN_POINT('Ctrl Pts',(-0.0861609852278712,-0.0750343524230471,
-0.641865144119882));
#43100=CARTESIAN_POINT('Ctrl Pts',(0.0162788671133667,-0.113087876912112,
-0.635516253775236));
#43101=CARTESIAN_POINT('Ctrl Pts',(0.103826419834063,-0.0476858885145751,
-0.629167363430591));
#43102=CARTESIAN_POINT('Ctrl Pts',(0.096391063613419,0.0613402989433316,
-0.622818473085946));
#43103=CARTESIAN_POINT('Ctrl Pts',(0.000774841360944117,0.11425090389073,
-0.616469582741301));
#43104=CARTESIAN_POINT('Ctrl Pts',(-0.0955502244262325,0.062642030866505,
-0.610120692396655));
#43105=CARTESIAN_POINT('Ctrl Pts',(-0.104463644116912,-0.0462732803764618,
-0.603771802052011));
#43106=CARTESIAN_POINT('Ctrl Pts',(-0.0178112067483281,-0.11285668049855,
-0.597422911707364));
#43107=CARTESIAN_POINT('Ctrl Pts',(0.0851353514366683,-0.0761960717802332,
-0.59107402136272));
#43108=CARTESIAN_POINT('Ctrl Pts',(0.110198040119839,0.0301705381577773,
-0.584725131018074));
#43109=CARTESIAN_POINT('Ctrl Pts',(0.0344489081994947,0.108936413300817,
-0.578376240673429));
#43110=CARTESIAN_POINT('Ctrl Pts',(-0.0728149144505367,0.08804463443359,
-0.572027350328784));
#43111=CARTESIAN_POINT('Ctrl Pts',(-0.113465900022296,-0.013392496074814,
-0.565678459984138));
#43112=CARTESIAN_POINT('Ctrl Pts',(-0.0503155480636912,-0.102577848690806,
-0.559329569639494));
#43113=CARTESIAN_POINT('Ctrl Pts',(0.0588646788314206,-0.097922515312145,
-0.552980679294847));
#43114=CARTESIAN_POINT('Ctrl Pts',(0.114194080105829,-0.00368530701123027,
-0.546631788950203));
#43115=CARTESIAN_POINT('Ctrl Pts',(0.0650559871753232,0.0939233088835127,
-0.540282898605557));
#43116=CARTESIAN_POINT('Ctrl Pts',(-0.0435968893318331,0.105608620195377,
-0.533934008260913));
#43117=CARTESIAN_POINT('Ctrl Pts',(-0.112366281691608,0.0206806227610694,
-0.527585117916266));
#43118=CARTESIAN_POINT('Ctrl Pts',(-0.0783402938480742,-0.0831665063519015,
-0.521236227571622));
#43119=CARTESIAN_POINT('Ctrl Pts',(0.0273532811943798,-0.110930912855185,
-0.514887337226976));
#43120=CARTESIAN_POINT('Ctrl Pts',(0.108023415949815,-0.0372130491295291,
-0.508538446882331));
#43121=CARTESIAN_POINT('Ctrl Pts',(0.0898711286561028,0.0705482080074449,
-0.502189556537686));
#43122=CARTESIAN_POINT('Ctrl Pts',(-0.0104974311744136,0.113770265701201,
-0.495840666193041));
#43123=CARTESIAN_POINT('Ctrl Pts',(-0.101262688194809,0.0529125448125908,
-0.489491775848395));
#43124=CARTESIAN_POINT('Ctrl Pts',(-0.0993903997105554,-0.0563508461725251,
-0.48314288550375));
#43125=CARTESIAN_POINT('Ctrl Pts',(-0.00659338031061752,-0.114063126184859,
-0.476793995159105));
#43126=CARTESIAN_POINT('Ctrl Pts',(0.0922354221620667,-0.0674277117924733,
-0.47044510481446));
#43127=CARTESIAN_POINT('Ctrl Pts',(0.106685039467939,0.0408921969660201,
-0.464096214469814));
#43128=CARTESIAN_POINT('Ctrl Pts',(0.0235366137575775,0.111802939280728,
-0.45774732412517));
#43129=CARTESIAN_POINT('Ctrl Pts',(-0.081143672965582,0.080433660594543,
-0.451398433780523));
#43130=CARTESIAN_POINT('Ctrl Pts',(-0.111591773769459,-0.0245182675972318,
-0.445049543435879));
#43131=CARTESIAN_POINT('Ctrl Pts',(-0.0399530328668883,-0.107040294206064,
-0.438700653091233));
#43132=CARTESIAN_POINT('Ctrl Pts',(0.0682357045470802,-0.0916392822099074,
-0.432351762746588));
#43133=CARTESIAN_POINT('Ctrl Pts',(0.114000776367053,0.00759555177013864,
-0.426002872401942));
#43134=CARTESIAN_POINT('Ctrl Pts',(0.0554751928969789,0.0998817920945878,
-0.419653982057298));
#43135=CARTESIAN_POINT('Ctrl Pts',(-0.0538004328442067,0.10079376391801,
-0.413305091712651));
#43136=CARTESIAN_POINT('Ctrl Pts',(-0.113858127137762,0.00949717345661038,
-0.406956201368007));
#43137=CARTESIAN_POINT('Ctrl Pts',(-0.0697556650911323,-0.0904876599690656,
-0.400607311023361));
#43138=CARTESIAN_POINT('Ctrl Pts',(0.0381609590549173,-0.107692203167139,
-0.394258420678717));
#43139=CARTESIAN_POINT('Ctrl Pts',(0.111167018964811,-0.0263773257450609,
-0.387909530334071));
#43140=CARTESIAN_POINT('Ctrl Pts',(0.0824748130913862,0.0790681644185857,
-0.381560639989426));
#43141=CARTESIAN_POINT('Ctrl Pts',(-0.0216673377414524,0.112180193858725,
-0.37521174964478));
#43142=CARTESIAN_POINT('Ctrl Pts',(-0.105987686272075,0.042667080725961,
-0.368862859300135));
#43143=CARTESIAN_POINT('Ctrl Pts',(-0.0933479472818827,-0.0658789052523071,
-0.36251396895549));
#43144=CARTESIAN_POINT('Ctrl Pts',(0.00468874164365965,-0.114157282381732,
-0.356165078610845));
#43145=CARTESIAN_POINT('Ctrl Pts',(0.09843605681153,-0.0580018287503136,
-0.349816188266199));
#43146=CARTESIAN_POINT('Ctrl Pts',(0.102131696927743,0.0512150944707055,
-0.343467297921554));
#43147=CARTESIAN_POINT('Ctrl Pts',(0.0123948014252152,0.113579216041549,
-0.337118407576909));
#43148=CARTESIAN_POINT('Ctrl Pts',(-0.0886811568803896,0.0720383358590353,
-0.330769517232263));
#43149=CARTESIAN_POINT('Ctrl Pts',(-0.108629457483411,-0.0354049486067051,
-0.324420626887619));
#43150=CARTESIAN_POINT('Ctrl Pts',(-0.0292009146492382,-0.11045893355737,
-0.318071736542973));
#43151=CARTESIAN_POINT('Ctrl Pts',(0.0769413280463485,-0.0844624263057108,
-0.311722846198328));
#43152=CARTESIAN_POINT('Ctrl Pts',(0.112695791144682,0.0188023423343459,
-0.305373955853682));
#43153=CARTESIAN_POINT('Ctrl Pts',(0.0453534308576449,0.104866275457958,
-0.299025065509037));
#43154=CARTESIAN_POINT('Ctrl Pts',(-0.0634793400610372,0.094996014676399,
-0.292676175164392));
#43155=CARTESIAN_POINT('Ctrl Pts',(-0.114239682147924,-0.0017788877774734,
-0.286327284819747));
#43156=CARTESIAN_POINT('Ctrl Pts',(-0.0604908121837178,-0.0969264208579767,
-0.279978394475101));
#43157=CARTESIAN_POINT('Ctrl Pts',(0.0485965093481745,-0.103403330208249,
-0.273629504130457));
#43158=CARTESIAN_POINT('Ctrl Pts',(0.113226573953927,-0.0152843831946183,
-0.267280613785811));
#43159=CARTESIAN_POINT('Ctrl Pts',(0.074274242279478,0.0868170856041166,
-0.260931723441166));
#43160=CARTESIAN_POINT('Ctrl Pts',(-0.0326259547108729,0.109496193989502,
-0.25458283309652));
#43161=CARTESIAN_POINT('Ctrl Pts',(-0.109679142718567,0.0320055475114412,
-0.248233942751875));
#43162=CARTESIAN_POINT('Ctrl Pts',(-0.0863952099601143,-0.074764544504249,
-0.24188505240723));
#43163=CARTESIAN_POINT('Ctrl Pts',(0.0159251412139454,-0.113138230922594,
-0.235536162062585));
#43164=CARTESIAN_POINT('Ctrl Pts',(0.103676789737939,-0.0480103393931116,
-0.229187271717939));
#43165=CARTESIAN_POINT('Ctrl Pts',(0.0965824145351879,0.0610385666731131,
-0.222838381373294));
#43166=CARTESIAN_POINT('Ctrl Pts',(0.0011321208704043,0.114247922174953,
-0.216489491028648));
#43167=CARTESIAN_POINT('Ctrl Pts',(-0.0953538642286377,0.0629405274509425,
-0.210140600684003));
#43168=CARTESIAN_POINT('Ctrl Pts',(-0.104607838265844,-0.045946377355595,
-0.203791710339358));
#43169=CARTESIAN_POINT('Ctrl Pts',(-0.0181640429686614,-0.112800429794994,
-0.197442819994713));
#43170=CARTESIAN_POINT('Ctrl Pts',(0.0848966562237705,-0.0764619328946917,
-0.191093929650067));
#43171=CARTESIAN_POINT('Ctrl Pts',(0.11029185002685,0.029825781379531,-0.184745039305422));
#43172=CARTESIAN_POINT('Ctrl Pts',(0.0347894036947918,0.108828152651674,
-0.178396148960777));
#43173=CARTESIAN_POINT('Ctrl Pts',(-0.0725392269022447,0.0882719093800321,
-0.172047258616132));
#43174=CARTESIAN_POINT('Ctrl Pts',(-0.113507225919962,-0.0130376021601832,
-0.165698368271487));
#43175=CARTESIAN_POINT('Ctrl Pts',(-0.0506360816870214,-0.102420001242717,
-0.159349477926841));
#43176=CARTESIAN_POINT('Ctrl Pts',(0.0585581697499888,-0.0981061170983672,
-0.153000587582196));
#43177=CARTESIAN_POINT('Ctrl Pts',(0.114181996713574,-0.00404239446648764,
-0.146651697237551));
#43178=CARTESIAN_POINT('Ctrl Pts',(0.0653493850557507,0.0937194075251059,
-0.140302806892906));
#43179=CARTESIAN_POINT('Ctrl Pts',(-0.0432664202898733,0.105744439634424,
-0.13395391654826));
#43180=CARTESIAN_POINT('Ctrl Pts',(-0.112301057470237,0.0210319105336957,
-0.127605026203615));
#43181=CARTESIAN_POINT('Ctrl Pts',(-0.0785999927227247,-0.0829211137801427,
-0.121256135858969));
#43182=CARTESIAN_POINT('Ctrl Pts',(0.02700625619051,-0.111015912167295,
-0.114907245514325));
#43183=CARTESIAN_POINT('Ctrl Pts',(0.107906497161016,-0.0375506701933854,
-0.108558355169679));
#43184=CARTESIAN_POINT('Ctrl Pts',(0.0900913416102402,0.0702668087494677,
-0.102209464825034));
#43185=CARTESIAN_POINT('Ctrl Pts',(-0.0101416666357262,0.113802557607322,
-0.0958605744803883));
#43186=CARTESIAN_POINT('Ctrl Pts',(-0.101096598775461,0.0532289133730042,
-0.0895116841357433));
#43187=CARTESIAN_POINT('Ctrl Pts',(-0.0995663742066905,-0.0560396839009997,
-0.0831627937910978));
#43188=CARTESIAN_POINT('Ctrl Pts',(-0.00694958676658794,-0.114042091871885,
-0.0768139034464529));
#43189=CARTESIAN_POINT('Ctrl Pts',(0.0920232450043284,-0.0677155494623698,
-0.0704650131018075));
#43190=CARTESIAN_POINT('Ctrl Pts',(0.106814040378024,0.0405578623688256,
-0.0641161227571624));
#43191=CARTESIAN_POINT('Ctrl Pts',(0.0238830063610432,0.111729758858221,
-0.057767232412517));
#43192=CARTESIAN_POINT('Ctrl Pts',(-0.0808858272408635,0.0806851793959811,
-0.0514183420678718));
#43193=CARTESIAN_POINT('Ctrl Pts',(-0.111679127879553,-0.024165691358642,
-0.0450694517232264));
#43194=CARTESIAN_POINT('Ctrl Pts',(-0.0402662619737551,-0.106921455580305,
-0.0387205613785813));
#43195=CARTESIAN_POINT('Ctrl Pts',(0.0679082340930717,-0.0918395816349683,
-0.0323716710339359));
#43196=CARTESIAN_POINT('Ctrl Pts',(0.114102150823536,0.00721443260332955,
-0.0260227806892906));
#43197=CARTESIAN_POINT('Ctrl Pts',(0.0556285462168408,0.0997595234912466,
-0.0196738903446454));
#43198=CARTESIAN_POINT('Ctrl Pts',(-0.0168574189684883,0.100472359437058,
-0.0154412967815485));
#43199=CARTESIAN_POINT('Ctrl Pts',(-0.0452560140322605,0.0854280329804675,
-0.013325));
#43200=CARTESIAN_POINT('Ctrl Pts',(-0.0724605943221351,-0.0518199049426062,
-1.1580911015872));
#43201=CARTESIAN_POINT('Ctrl Pts',(-0.055234252507093,-0.075907771705324,
-1.15597480480565));
#43202=CARTESIAN_POINT('Ctrl Pts',(0.0048262281991512,-0.105141021982032,
-1.15174221124255));
#43203=CARTESIAN_POINT('Ctrl Pts',(0.0911131742662497,-0.0528906217674777,
-1.14539332089791));
#43204=CARTESIAN_POINT('Ctrl Pts',(0.0937758792848175,0.0477872397960602,
-1.13904443055326));
#43205=CARTESIAN_POINT('Ctrl Pts',(0.010786960009752,0.104726182257502,
-1.13269554020861));
#43206=CARTESIAN_POINT('Ctrl Pts',(-0.0821414930851173,0.0658706872743175,
-1.12634664986397));
#43207=CARTESIAN_POINT('Ctrl Pts',(-0.0998873948555119,-0.0332510120693374,
-1.11999775951932));
#43208=CARTESIAN_POINT('Ctrl Pts',(-0.0262736828112808,-0.101950661539774,
-1.11364886917468));
#43209=CARTESIAN_POINT('Ctrl Pts',(0.0713862550159982,-0.0773850904791992,
-1.10729997883003));
#43210=CARTESIAN_POINT('Ctrl Pts',(0.103734829621343,0.0179751208498506,
-1.10095108848539));
#43211=CARTESIAN_POINT('Ctrl Pts',(0.0411871831950449,0.0968907863086817,
-1.09460219814074));
#43212=CARTESIAN_POINT('Ctrl Pts',(-0.0590410187023357,0.0871686765058855,
-1.0882533077961));
#43213=CARTESIAN_POINT('Ctrl Pts',(-0.10525626908595,-0.00229756888763826,
-1.08190441745145));
#43214=CARTESIAN_POINT('Ctrl Pts',(-0.055180974941425,-0.0896618736803812,
-1.07555552710681));
#43215=CARTESIAN_POINT('Ctrl Pts',(0.0453754278584056,-0.0950013739441941,
-1.06920663676216));
#43216=CARTESIAN_POINT('Ctrl Pts',(0.104421178504928,-0.013431310494212,
-1.06285774641752));
#43217=CARTESIAN_POINT('Ctrl Pts',(0.0679399829451714,0.0804260290616174,
-1.05650885607287));
#43218=CARTESIAN_POINT('Ctrl Pts',(-0.0306943778088397,0.100707705974746,
-1.05015996572823));
#43219=CARTESIAN_POINT('Ctrl Pts',(-0.101248765324717,0.0288595456594365,
-1.04381107538358));
#43220=CARTESIAN_POINT('Ctrl Pts',(-0.0791783534431802,-0.0693900204573446,
-1.03746218503894));
#43221=CARTESIAN_POINT('Ctrl Pts',(0.0153263275489798,-0.104159925774821,
-1.03111329469429));
#43222=CARTESIAN_POINT('Ctrl Pts',(0.0958101125123582,-0.0436418224720267,
-1.02476440434965));
#43223=CARTESIAN_POINT('Ctrl Pts',(0.0886445008384644,0.0568008706786289,
-1.018415514005));
#43224=CARTESIAN_POINT('Ctrl Pts',(0.000384764586127094,0.105280759717015,
-1.01206662366036));
#43225=CARTESIAN_POINT('Ctrl Pts',(-0.0882269632024242,0.0574472746088744,
-1.00571773331571));
#43226=CARTESIAN_POINT('Ctrl Pts',(-0.0961265407978823,-0.042940360574977,
-0.999368842971065));
#43227=CARTESIAN_POINT('Ctrl Pts',(-0.0160872440992713,-0.104045119943892,
-0.993019952626418));
#43228=CARTESIAN_POINT('Ctrl Pts',(0.0786690508178819,-0.069966898235941,
-0.986671062281774));
#43229=CARTESIAN_POINT('Ctrl Pts',(0.101457003772623,0.028118726733982,
-0.980322171937128));
#43230=CARTESIAN_POINT('Ctrl Pts',(0.0314296466379681,0.100480663408266,
-0.973973281592484));
#43231=CARTESIAN_POINT('Ctrl Pts',(-0.0673503080399109,0.0809204696820091,
-0.967624391247837));
#43232=CARTESIAN_POINT('Ctrl Pts',(-0.104516579172577,-0.0126677182244316,
-0.961275500903192));
#43233=CARTESIAN_POINT('Ctrl Pts',(-0.0460685669801909,-0.0946671724685623,
-0.954926610558547));
#43234=CARTESIAN_POINT('Ctrl Pts',(0.0545240795876188,-0.0900628178102374,
-0.948577720213902));
#43235=CARTESIAN_POINT('Ctrl Pts',(0.105236785242567,-0.00306682876124731,
-0.942228829869257));
#43236=CARTESIAN_POINT('Ctrl Pts',(0.0596763457194078,0.0867347690859587,
-0.935879939524611));
#43237=CARTESIAN_POINT('Ctrl Pts',(-0.0404774518378589,0.097189311652734,
-0.929531049179967));
#43238=CARTESIAN_POINT('Ctrl Pts',(-0.103601501781483,0.0187327316599986,
-0.923182158835321));
#43239=CARTESIAN_POINT('Ctrl Pts',(-0.0719484032341107,-0.0768610023281135,
-0.916833268490676));
#43240=CARTESIAN_POINT('Ctrl Pts',(0.0255248270656589,-0.102140440620203,
-0.91048437814603));
#43241=CARTESIAN_POINT('Ctrl Pts',(0.0996473309434417,-0.0339793443531499,
-0.904135487801385));
#43242=CARTESIAN_POINT('Ctrl Pts',(0.0826100570269412,0.0652668743301431,
-0.89778659745674));
#43243=CARTESIAN_POINT('Ctrl Pts',(-0.0100008862578078,0.104805384789522,
-0.891437707112095));
#43244=CARTESIAN_POINT('Ctrl Pts',(-0.0934627779786483,0.0484654055934257,
-0.885088816767449));
#43245=CARTESIAN_POINT('Ctrl Pts',(-0.0914226698776842,-0.0522118936570709,
-0.878739926422805));
#43246=CARTESIAN_POINT('Ctrl Pts',(-0.00574690197024275,-0.105124495359387,
-0.872391036078158));
#43247=CARTESIAN_POINT('Ctrl Pts',(0.0851862702414863,-0.0618666773729265,
-0.866042145733514));
#43248=CARTESIAN_POINT('Ctrl Pts',(0.0981889912026475,0.0379882667863077,
-0.859693255388868));
#43249=CARTESIAN_POINT('Ctrl Pts',(0.0213660586803464,0.103090629755033,
-0.853344365044224));
#43250=CARTESIAN_POINT('Ctrl Pts',(-0.0750030588044541,0.0738832022640935,
-0.846995474699577));
#43251=CARTESIAN_POINT('Ctrl Pts',(-0.102757572066831,-0.0229143577206821,
-0.840646584354933));
#43252=CARTESIAN_POINT('Ctrl Pts',(-0.0365069840625374,-0.0987493114987594,
-0.834297694010287));
#43253=CARTESIAN_POINT('Ctrl Pts',(0.0631410720281716,-0.0842460172943181,
-0.827948803665642));
#43254=CARTESIAN_POINT('Ctrl Pts',(0.105026155028839,0.00732756212390092,
-0.821599913320996));
#43255=CARTESIAN_POINT('Ctrl Pts',(0.0508307824430911,0.0921977112679295,
-0.815251022976352));
#43256=CARTESIAN_POINT('Ctrl Pts',(-0.0498658138959695,0.0927231740791579,
-0.808902132631705));
#43257=CARTESIAN_POINT('Ctrl Pts',(-0.104943962944481,0.00842324452504938,
-0.802553242287061));
#43258=CARTESIAN_POINT('Ctrl Pts',(-0.0640168477044826,-0.0835824719471878,
-0.796204351942415));
#43259=CARTESIAN_POINT('Ctrl Pts',(0.0354744213023932,-0.0991249304669698,
-0.789855461597771));
#43260=CARTESIAN_POINT('Ctrl Pts',(0.102512835499318,-0.0239855157274384,
-0.783506571253125));
#43261=CARTESIAN_POINT('Ctrl Pts',(0.0757700393346405,0.0730964263562066,
-0.777157680908479));
#43262=CARTESIAN_POINT('Ctrl Pts',(-0.0202890133098994,0.103307997491637,
-0.770808790563835));
#43263=CARTESIAN_POINT('Ctrl Pts',(-0.0977871880314241,0.0390109249278746,
-0.764459900219188));
#43264=CARTESIAN_POINT('Ctrl Pts',(-0.0858272884856976,-0.0609742811192895,
-0.758111009874544));
#43265=CARTESIAN_POINT('Ctrl Pts',(0.00464948123573095,-0.105178746574866,
-0.751762119529899));
#43266=CARTESIAN_POINT('Ctrl Pts',(0.0908727935660286,-0.0531631620234097,
-0.745413229185254));
#43267=CARTESIAN_POINT('Ctrl Pts',(0.0939634861804381,0.0474873632837188,
-0.739064338840607));
#43268=CARTESIAN_POINT('Ctrl Pts',(0.0110941190532975,0.104695305192032,
-0.732715448495963));
#43269=CARTESIAN_POINT('Ctrl Pts',(-0.0819244153234499,0.0661254609113028,
-0.726366558151318));
#43270=CARTESIAN_POINT('Ctrl Pts',(-0.0999965218721342,-0.0329375472720281,
-0.720017667806672));
#43271=CARTESIAN_POINT('Ctrl Pts',(-0.0265894023566692,-0.101868494094771,
-0.713668777462027));
#43272=CARTESIAN_POINT('Ctrl Pts',(0.0711423426913388,-0.0776076895881424,
-0.707319887117382));
#43273=CARTESIAN_POINT('Ctrl Pts',(0.103791359580901,0.0176504980997559,
-0.700970996772737));
#43274=CARTESIAN_POINT('Ctrl Pts',(0.0414895414929455,0.0967615851127215,
-0.69462210642809));
#43275=CARTESIAN_POINT('Ctrl Pts',(-0.0587679081957195,0.087352844104361,
-0.688273216083447));
#43276=CARTESIAN_POINT('Ctrl Pts',(-0.1052630603714,-0.00196838209410804,
-0.681924325738799));
#43277=CARTESIAN_POINT('Ctrl Pts',(-0.0554610302487527,-0.0894888849554417,
-0.675575435394156));
#43278=CARTESIAN_POINT('Ctrl Pts',(0.0450780858133816,-0.0951428010215314,
-0.66922654504951));
#43279=CARTESIAN_POINT('Ctrl Pts',(0.104378683520503,-0.0137577917322536,
-0.662877654704865));
#43280=CARTESIAN_POINT('Ctrl Pts',(0.0681911481677555,0.0802131767129601,
-0.65652876436022));
#43281=CARTESIAN_POINT('Ctrl Pts',(-0.0303792915302921,0.100803199616574,
-0.650179874015574));
#43282=CARTESIAN_POINT('Ctrl Pts',(-0.101158023821536,0.0291760282311139,
-0.643830983670929));
#43283=CARTESIAN_POINT('Ctrl Pts',(-0.0793949600970565,-0.0691420763212106,
-0.637482093326283));
#43284=CARTESIAN_POINT('Ctrl Pts',(0.0150005249066355,-0.104207344555683,
-0.631133202981639));
#43285=CARTESIAN_POINT('Ctrl Pts',(0.0956731685222073,-0.0439412247410412,
-0.624784312636993));
#43286=CARTESIAN_POINT('Ctrl Pts',(0.0888216938218651,0.056523385544712,
-0.618435422292349));
#43287=CARTESIAN_POINT('Ctrl Pts',(0.000713994840833118,0.105279041685364,
-0.612086531947701));
#43288=CARTESIAN_POINT('Ctrl Pts',(-0.0880468838131556,0.0577228954368544,
-0.605737641603059));
#43289=CARTESIAN_POINT('Ctrl Pts',(-0.0962603530393757,-0.0426395454895582,
-0.599388751258411));
#43290=CARTESIAN_POINT('Ctrl Pts',(-0.0164125334143298,-0.103994303467761,
-0.593039860913768));
#43291=CARTESIAN_POINT('Ctrl Pts',(0.0784498669819821,-0.0702125685139818,
-0.586690970569121));
#43292=CARTESIAN_POINT('Ctrl Pts',(0.101544440038021,0.0278013147923997,
-0.580342080224476));
#43293=CARTESIAN_POINT('Ctrl Pts',(0.0317437142188269,0.100381885887917,
-0.573993189879831));
#43294=CARTESIAN_POINT('Ctrl Pts',(-0.0670969257371112,0.0811306906383144,
-0.567644299535187));
#43295=CARTESIAN_POINT('Ctrl Pts',(-0.104555682375514,-0.0123408139849797,
-0.56129540919054));
#43296=CARTESIAN_POINT('Ctrl Pts',(-0.0463643831394596,-0.0945226448155085,
-0.554946518845896));
#43297=CARTESIAN_POINT('Ctrl Pts',(0.0542421702187635,-0.0902328841209236,
-0.54859762850125));
#43298=CARTESIAN_POINT('Ctrl Pts',(0.105226680142342,-0.00339590827946428,
-0.542248738156605));
#43299=CARTESIAN_POINT('Ctrl Pts',(0.0599472892771499,0.0865477262274584,
-0.53589984781196));
#43300=CARTESIAN_POINT('Ctrl Pts',(-0.040173325313101,0.0973154167648122,
-0.529550957467314));
#43301=CARTESIAN_POINT('Ctrl Pts',(-0.103542414557649,0.0190566207495772,
-0.523202067122669));
#43302=CARTESIAN_POINT('Ctrl Pts',(-0.0721884097263963,-0.0766356307992258,
-0.516853176778024));
#43303=CARTESIAN_POINT('Ctrl Pts',(0.0252052905756322,-0.102219761953447,
-0.510504286433378));
#43304=CARTESIAN_POINT('Ctrl Pts',(0.0995405841309819,-0.0342907934828616,
-0.504155396088733));
#43305=CARTESIAN_POINT('Ctrl Pts',(0.0828137544464914,0.0650082185673283,
-0.497806505744088));
#43306=CARTESIAN_POINT('Ctrl Pts',(-0.00967309191056538,0.104836146913701,
-0.491457615399442));
#43307=CARTESIAN_POINT('Ctrl Pts',(-0.0933107608656584,0.0487574436726666,
-0.485108725054797));
#43308=CARTESIAN_POINT('Ctrl Pts',(-0.0915854989143904,-0.0519257430897579,
-0.478759834710152));
#43309=CARTESIAN_POINT('Ctrl Pts',(-0.00607561723304139,-0.105106009733311,
-0.472410944365507));
#43310=CARTESIAN_POINT('Ctrl Pts',(0.0849923853902668,-0.0621327677839452,
-0.466062054020862));
#43311=CARTESIAN_POINT('Ctrl Pts',(0.098307307293533,0.0376810262534904,
-0.459713163676216));
#43312=CARTESIAN_POINT('Ctrl Pts',(0.0216883373044148,0.103023310138003,
-0.453364273331571));
#43313=CARTESIAN_POINT('Ctrl Pts',(-0.0747716458927733,0.0741173891695262,
-0.447015382986926));
#43314=CARTESIAN_POINT('Ctrl Pts',(-0.102828726971427,-0.0225929041129553,
-0.44066649264228));
#43315=CARTESIAN_POINT('Ctrl Pts',(-0.0368156125633175,-0.0986346646894945,
-0.434317602297635));
#43316=CARTESIAN_POINT('Ctrl Pts',(0.062877310715307,-0.0844430589452562,
-0.42796871195299));
#43317=CARTESIAN_POINT('Ctrl Pts',(0.105048556104111,0.00699909045968183,
-0.421619821608345));
#43318=CARTESIAN_POINT('Ctrl Pts',(0.0511188528634354,0.0920383033782552,
-0.4152709312637));
#43319=CARTESIAN_POINT('Ctrl Pts',(-0.049575607887644,0.0928786601399474,
-0.408922040919054));
#43320=CARTESIAN_POINT('Ctrl Pts',(-0.104917108792576,0.00875138214388225,
-0.402573150574409));
#43321=CARTESIAN_POINT('Ctrl Pts',(-0.0642779122337915,-0.083381870965374,
-0.396224260229764));
#43322=CARTESIAN_POINT('Ctrl Pts',(0.0351642662095556,-0.0992353807306885,
-0.389875369885118));
#43323=CARTESIAN_POINT('Ctrl Pts',(0.102437327190227,-0.0243059746758653,
-0.383526479540474));
#43324=CARTESIAN_POINT('Ctrl Pts',(0.0759982546286465,0.0728591222855505,
-0.377177589195827));
#43325=CARTESIAN_POINT('Ctrl Pts',(-0.0199658512590393,0.103370939776724,
-0.370828698851183));
#43326=CARTESIAN_POINT('Ctrl Pts',(-0.0976647156493817,0.0393165324506968,
-0.364479808506537));
#43327=CARTESIAN_POINT('Ctrl Pts',(-0.0860175464566275,-0.0607055854794545,
-0.358130918161892));
#43328=CARTESIAN_POINT('Ctrl Pts',(0.00432054548493318,-0.105192772059367,
-0.351782027817247));
#43329=CARTESIAN_POINT('Ctrl Pts',(0.0907060983807646,-0.0534470777813002,
-0.345433137472601));
#43330=CARTESIAN_POINT('Ctrl Pts',(0.0941115283301076,0.0471932902242764,
-0.339084247127957));
#43331=CARTESIAN_POINT('Ctrl Pts',(0.0114214660146163,0.104660099946915,
-0.332735356783311));
#43332=CARTESIAN_POINT('Ctrl Pts',(-0.0817172284330107,0.0663813300864664,
-0.326386466438666));
#43333=CARTESIAN_POINT('Ctrl Pts',(-0.100099034608884,-0.0326246789591988,
-0.32003757609402));
#43334=CARTESIAN_POINT('Ctrl Pts',(-0.0269078336005834,-0.101784846110532,
-0.313688685749375));
#43335=CARTESIAN_POINT('Ctrl Pts',(0.0708993015098229,-0.0778297851226668,
-0.30733979540473));
#43336=CARTESIAN_POINT('Ctrl Pts',(0.103846048386919,0.0173258373893755,
-0.300990905060084));
#43337=CARTESIAN_POINT('Ctrl Pts',(0.0417919296498781,0.0966313666619745,
-0.294642014715439));
#43338=CARTESIAN_POINT('Ctrl Pts',(-0.0584944526551572,0.0875361948875711,
-0.288293124370794));
#43339=CARTESIAN_POINT('Ctrl Pts',(-0.105268701160358,-0.00163919578839571,
-0.281944234026149));
#43340=CARTESIAN_POINT('Ctrl Pts',(-0.0557406070376653,-0.0893150106862998,
-0.275595343681503));
#43341=CARTESIAN_POINT('Ctrl Pts',(0.0447803366030493,-0.0952833031571579,
-0.269246453336859));
#43342=CARTESIAN_POINT('Ctrl Pts',(0.104335150035986,-0.0140841355357712,
-0.262897562992213));
#43343=CARTESIAN_POINT('Ctrl Pts',(0.0684416558889433,0.0799995384111712,
-0.256548672647568));
#43344=CARTESIAN_POINT('Ctrl Pts',(-0.0300639130988035,0.100897708279267,
-0.250199782302922));
#43345=CARTESIAN_POINT('Ctrl Pts',(-0.101066290463019,0.0294922250579535,
-0.243850891958277));
#43346=CARTESIAN_POINT('Ctrl Pts',(-0.0796107916967184,-0.0688934558012595,
-0.237502001613632));
#43347=CARTESIAN_POINT('Ctrl Pts',(0.0146745762931698,-0.104253744380875,
-0.231153111268987));
#43348=CARTESIAN_POINT('Ctrl Pts',(0.0955352885353473,-0.0442401972340638,
-0.224804220924341));
#43349=CARTESIAN_POINT('Ctrl Pts',(0.0889980183933423,0.0562453476196506,
-0.218455330579696));
#43350=CARTESIAN_POINT('Ctrl Pts',(0.00104321800746791,0.105276294116908,
-0.212106440235051));
#43351=CARTESIAN_POINT('Ctrl Pts',(-0.0878659433328274,0.0579979517671395,
-0.205757549890405));
#43352=CARTESIAN_POINT('Ctrl Pts',(-0.0963932239515455,-0.0423383134153348,
-0.19940865954576));
#43353=CARTESIAN_POINT('Ctrl Pts',(-0.0167376622131716,-0.103942470003317,
-0.193059769201115));
#43354=CARTESIAN_POINT('Ctrl Pts',(0.078229915958288,-0.0704575521631122,
-0.18671087885647));
#43355=CARTESIAN_POINT('Ctrl Pts',(0.101630883267566,0.0274836309755344,
-0.180361988511825));
#43356=CARTESIAN_POINT('Ctrl Pts',(0.0320574713815479,0.100282126699974,
-0.174013098167179));
#43357=CARTESIAN_POINT('Ctrl Pts',(-0.0668428873015247,0.0813401182029611,
-0.167664207822534));
#43358=CARTESIAN_POINT('Ctrl Pts',(-0.104593763044944,-0.012013789077868,
-0.161315317477889));
#43359=CARTESIAN_POINT('Ctrl Pts',(-0.046659745990369,-0.0943771927665409,
-0.154966427133243));
#43360=CARTESIAN_POINT('Ctrl Pts',(0.0539597305945496,-0.0904020680787478,
-0.148617536788598));
#43361=CARTESIAN_POINT('Ctrl Pts',(0.105215545631247,-0.00372495447347343,
-0.142268646443953));
#43362=CARTESIAN_POINT('Ctrl Pts',(0.0602176472929908,0.0863598367764309,
-0.135919756099308));
#43363=CARTESIAN_POINT('Ctrl Pts',(-0.0398688072492659,0.0974405706139124,
-0.129570865754662));
#43364=CARTESIAN_POINT('Ctrl Pts',(-0.103482312245223,0.0193803226967692,
-0.123221975410017));
#43365=CARTESIAN_POINT('Ctrl Pts',(-0.0724277150423184,-0.0764095083449458,
-0.116873085065372));
#43366=CARTESIAN_POINT('Ctrl Pts',(0.0248855166517145,-0.102298086463958,
-0.110524194720727));
#43367=CARTESIAN_POINT('Ctrl Pts',(0.0994328467072885,-0.0346019019366694,
-0.104175304376081));
#43368=CARTESIAN_POINT('Ctrl Pts',(0.0830166745809391,0.0647489169495561,
-0.0978264140314359));
#43369=CARTESIAN_POINT('Ctrl Pts',(-0.00934526474751318,0.104865903010281,
-0.0914775236867907));
#43370=CARTESIAN_POINT('Ctrl Pts',(-0.0931577140685862,0.0490489685335253,
-0.0851286333421453));
#43371=CARTESIAN_POINT('Ctrl Pts',(-0.0917476545357751,-0.0516390156798273,
-0.0787797429975));
#43372=CARTESIAN_POINT('Ctrl Pts',(-0.00640385161062303,-0.105086627196832,
-0.0724308526528549));
#43373=CARTESIAN_POINT('Ctrl Pts',(0.0847968700195037,-0.0623980022198728,
-0.0660819623082098));
#43374=CARTESIAN_POINT('Ctrl Pts',(0.0984261780571572,0.0373729461876333,
-0.0597330719635643));
#43375=CARTESIAN_POINT('Ctrl Pts',(0.0220075284888858,0.102955876406722,
-0.0533841816189193));
#43376=CARTESIAN_POINT('Ctrl Pts',(-0.0745340482031569,0.0743491567746786,
-0.0470352912742738));
#43377=CARTESIAN_POINT('Ctrl Pts',(-0.102909221363023,-0.0222680148800854,
-0.0406864009296286));
#43378=CARTESIAN_POINT('Ctrl Pts',(-0.037104244504737,-0.0985251581892469,
-0.0343375105849833));
#43379=CARTESIAN_POINT('Ctrl Pts',(0.0625755557671689,-0.0846276293145263,
-0.027988620240338));
#43380=CARTESIAN_POINT('Ctrl Pts',(0.105141969856357,0.00664789970947171,
-0.0216397298956927));
#43381=CARTESIAN_POINT('Ctrl Pts',(0.051260163697788,0.0919256362487216,
-0.0152908395510475));
#43382=CARTESIAN_POINT('Ctrl Pts',(-0.0155336444076485,0.0925824948178739,
-0.0110582459879506));
#43383=CARTESIAN_POINT('Ctrl Pts',(-0.0417021627450095,0.0787195649134732,
-0.00894194920640216));
#43384=CARTESIAN_POINT('Ctrl Pts',(-0.0662855146750388,-0.0474038213689184,
-1.1537080507936));
#43385=CARTESIAN_POINT('Ctrl Pts',(-0.0505271988088748,-0.0694389241820727,
-1.15159175401205));
#43386=CARTESIAN_POINT('Ctrl Pts',(0.00441493784466667,-0.0961809217925434,
-1.14735916044895));
#43387=CARTESIAN_POINT('Ctrl Pts',(0.0833485248970674,-0.0483832918862652,
-1.14101027010431));
#43388=CARTESIAN_POINT('Ctrl Pts',(0.0857843146423046,0.043714819267134,
-1.13466137975966));
#43389=CARTESIAN_POINT('Ctrl Pts',(0.00986769709404836,0.0958014346394865,
-1.12831248941502));
#43390=CARTESIAN_POINT('Ctrl Pts',(-0.0751414088755243,0.0602571983962171,
-1.12196359907037));
#43391=CARTESIAN_POINT('Ctrl Pts',(-0.0913750078851314,-0.0304173664196481,
-1.11561470872573));
#43392=CARTESIAN_POINT('Ctrl Pts',(-0.024034643986111,-0.0932624433299762,
-1.10926581838108));
#43393=CARTESIAN_POINT('Ctrl Pts',(0.0653027303836705,-0.070790346098793,
-1.10291692803644));
#43394=CARTESIAN_POINT('Ctrl Pts',(0.0948945649080561,0.016443284077706,
-1.09656803769179));
#43395=CARTESIAN_POINT('Ctrl Pts',(0.0376772183783308,0.0886337698140873,
-1.09021914734715));
#43396=CARTESIAN_POINT('Ctrl Pts',(-0.0540095530299468,0.0797401765716616,
-1.0838702570025));
#43397=CARTESIAN_POINT('Ctrl Pts',(-0.0962863475576708,-0.00210177045390104,
-1.07752136665785));
#43398=CARTESIAN_POINT('Ctrl Pts',(-0.0504784615483822,-0.0820209039027542,
-1.07117247631321));
#43399=CARTESIAN_POINT('Ctrl Pts',(0.0415085415367013,-0.0869053728531599,
-1.06482358596856));
#43400=CARTESIAN_POINT('Ctrl Pts',(0.0955224232553502,-0.0122866964754829,
-1.05847469562392));
#43401=CARTESIAN_POINT('Ctrl Pts',(0.0621501490384322,0.0735721364072543,
-1.05212580527927));
#43402=CARTESIAN_POINT('Ctrl Pts',(-0.0280786081003397,0.0921254122289098,
-1.04577691493463));
#43403=CARTESIAN_POINT('Ctrl Pts',(-0.0926203625921804,0.0264001400377588,
-1.03942802458998));
#43404=CARTESIAN_POINT('Ctrl Pts',(-0.0724307874949361,-0.0634766145979759,
-1.03307913424534));
#43405=CARTESIAN_POINT('Ctrl Pts',(0.0140202204959272,-0.0952834344389127,
-1.02673024390069));
#43406=CARTESIAN_POINT('Ctrl Pts',(0.0876451908567207,-0.0399226737094445,
-1.02038135355605));
#43407=CARTESIAN_POINT('Ctrl Pts',(0.0810902314031199,0.0519603100436204,
-1.0140324632114));
#43408=CARTESIAN_POINT('Ctrl Pts',(0.000351975012885768,0.0963087511012804,
-1.00768357286676));
#43409=CARTESIAN_POINT('Ctrl Pts',(-0.0807082762541159,0.0525516275397749,
-1.00133468252211));
#43410=CARTESIAN_POINT('Ctrl Pts',(-0.0879346531770343,-0.0392809902771458,
-0.994985792177466));
#43411=CARTESIAN_POINT('Ctrl Pts',(-0.0147162918659295,-0.0951784123415638,
-0.988636901832821));
#43412=CARTESIAN_POINT('Ctrl Pts',(0.071964887553607,-0.0640043309494178,
-0.982288011488176));
#43413=CARTESIAN_POINT('Ctrl Pts',(0.0928108549946201,0.0257224535763889,
-0.975939121143531));
#43414=CARTESIAN_POINT('Ctrl Pts',(0.0287512174436577,0.0919177181917147,
-0.969590230798886));
#43415=CARTESIAN_POINT('Ctrl Pts',(-0.0616107261293058,0.0740244408812324,
-0.963241340454239));
#43416=CARTESIAN_POINT('Ctrl Pts',(-0.0956096938941654,-0.0115881774103558,
-0.956892450109595));
#43417=CARTESIAN_POINT('Ctrl Pts',(-0.0421426114592421,-0.0865996519710071,
-0.950543559764949));
#43418=CARTESIAN_POINT('Ctrl Pts',(0.0498775467060162,-0.0823876796413767,
-0.944194669420304));
#43419=CARTESIAN_POINT('Ctrl Pts',(0.0962685241241404,-0.00280547413061279,
-0.937845779075659));
#43420=CARTESIAN_POINT('Ctrl Pts',(0.0545907375856034,0.0793432466689976,
-0.931496888731014));
#43421=CARTESIAN_POINT('Ctrl Pts',(-0.0370279702078962,0.0889068548785865,
-0.925147998386368));
#43422=CARTESIAN_POINT('Ctrl Pts',(-0.0947725992442585,0.0171363314221833,
-0.918799108041723));
#43423=CARTESIAN_POINT('Ctrl Pts',(-0.0658169724252926,-0.0703109206516945,
-0.912450217697078));
#43424=CARTESIAN_POINT('Ctrl Pts',(0.0233496056010352,-0.0934360494691271,
-0.906101327352432));
#43425=CARTESIAN_POINT('Ctrl Pts',(0.0911554021792248,-0.0310836303488742,
-0.899752437007787));
#43426=CARTESIAN_POINT('Ctrl Pts',(0.0755700418771249,0.0597048422894724,
-0.893403546663142));
#43427=CARTESIAN_POINT('Ctrl Pts',(-0.00914861241488205,0.0958738875450639,
-0.887054656318497));
#43428=CARTESIAN_POINT('Ctrl Pts',(-0.0854978957767257,0.0443351918894408,
-0.880705765973851));
#43429=CARTESIAN_POINT('Ctrl Pts',(-0.0836316453446097,-0.0477624048711401,
-0.874356875629207));
#43430=CARTESIAN_POINT('Ctrl Pts',(-0.00525715195201284,-0.0961658035658973,
-0.86800798528456));
#43431=CARTESIAN_POINT('Ctrl Pts',(0.0779267106353122,-0.056594409544421,
-0.861659094939916));
#43432=CARTESIAN_POINT('Ctrl Pts',(0.0898213419055841,0.0347509130873053,
-0.85531020459527));
#43433=CARTESIAN_POINT('Ctrl Pts',(0.019545246757261,0.0943052636458809,
-0.848961314250626));
#43434=CARTESIAN_POINT('Ctrl Pts',(-0.0686113107622776,0.0675868882077251,
-0.84261242390598));
#43435=CARTESIAN_POINT('Ctrl Pts',(-0.0940005890777867,-0.0209616000140822,
-0.836263533561334));
#43436=CARTESIAN_POINT('Ctrl Pts',(-0.0333958650278359,-0.0903339118004081,
-0.82991464321669));
#43437=CARTESIAN_POINT('Ctrl Pts',(0.0577602005017288,-0.0770665858859817,
-0.823565752872044));
#43438=CARTESIAN_POINT('Ctrl Pts',(0.09607584378176,0.00670310851352802,
-0.817216862527399));
#43439=CARTESIAN_POINT('Ctrl Pts',(0.0464989917222637,0.0843406378380802,
-0.810867972182753));
#43440=CARTESIAN_POINT('Ctrl Pts',(-0.0456162576322428,0.084821320797015,
-0.804519081838108));
#43441=CARTESIAN_POINT('Ctrl Pts',(-0.0960006560929914,0.00770541704494582,
-0.798170191493463));
#43442=CARTESIAN_POINT('Ctrl Pts',(-0.058561342722371,-0.0764595877616036,
-0.791821301148817));
#43443=CARTESIAN_POINT('Ctrl Pts',(0.0324512970922443,-0.0906775205833958,
-0.785472410804173));
#43444=CARTESIAN_POINT('Ctrl Pts',(0.0937767089193475,-0.0219414741158684,
-0.779123520459527));
#43445=CARTESIAN_POINT('Ctrl Pts',(0.0693129293408286,0.0668671612102279,
-0.772774630114882));
#43446=CARTESIAN_POINT('Ctrl Pts',(-0.0185599870119265,0.0945041073405723,
-0.766425739770236));
#43447=CARTESIAN_POINT('Ctrl Pts',(-0.0894537803329552,0.0356864204742467,
-0.760076849425591));
#43448=CARTESIAN_POINT('Ctrl Pts',(-0.0785131014126889,-0.0557780631492537,
-0.753727959080947));
#43449=CARTESIAN_POINT('Ctrl Pts',(0.0042532532277082,-0.0962154315019286,
-0.747379068736299));
#43450=CARTESIAN_POINT('Ctrl Pts',(0.0831286293996434,-0.0486326063074775,
-0.741030178391657));
#43451=CARTESIAN_POINT('Ctrl Pts',(0.08595593370987,0.0434404981806807,
-0.734681288047009));
#43452=CARTESIAN_POINT('Ctrl Pts',(0.0101486800956229,0.0957731889123362,
-0.728332397702366));
#43453=CARTESIAN_POINT('Ctrl Pts',(-0.0749428304441543,0.0604902602667578,
-0.721983507357719));
#43454=CARTESIAN_POINT('Ctrl Pts',(-0.0914748351157721,-0.0301306150395839,
-0.715634617013074));
#43455=CARTESIAN_POINT('Ctrl Pts',(-0.0243234579650029,-0.0931872781808012,
-0.70928572666843));
#43456=CARTESIAN_POINT('Ctrl Pts',(0.0650796042262482,-0.0709939753491537,
-0.702936836323783));
#43457=CARTESIAN_POINT('Ctrl Pts',(0.0949462773939787,0.0161463256237138,
-0.696587945979139));
#43458=CARTESIAN_POINT('Ctrl Pts',(0.0379538097529958,0.0885155791222918,
-0.690239055634493));
#43459=CARTESIAN_POINT('Ctrl Pts',(-0.0537597169547176,0.0799086494384053,
-0.683890165289848));
#43460=CARTESIAN_POINT('Ctrl Pts',(-0.0962925600909185,-0.00180063690348633,
-0.677541274945203));
#43461=CARTESIAN_POINT('Ctrl Pts',(-0.0507346505895757,-0.0818626572478259,
-0.671192384600557));
#43462=CARTESIAN_POINT('Ctrl Pts',(0.0412365389306873,-0.0870347475387801,
-0.664843494255913));
#43463=CARTESIAN_POINT('Ctrl Pts',(0.0954835496863418,-0.0125853550373922,
-0.658494603911266));
#43464=CARTESIAN_POINT('Ctrl Pts',(0.0623799100030393,0.0733774232999093,
-0.652145713566622));
#43465=CARTESIAN_POINT('Ctrl Pts',(-0.0277903734213952,0.0922127679186605,
-0.645796823221977));
#43466=CARTESIAN_POINT('Ctrl Pts',(-0.0925373540646213,0.0266896520179679,
-0.639447932877331));
#43467=CARTESIAN_POINT('Ctrl Pts',(-0.0726289349662417,-0.0632498002193741,
-0.633099042532686));
#43468=CARTESIAN_POINT('Ctrl Pts',(0.0137221826999042,-0.0953268121992537,
-0.626750152188041));
#43469=CARTESIAN_POINT('Ctrl Pts',(0.0875199172103516,-0.0401965609675073,
-0.620401261843396));
#43470=CARTESIAN_POINT('Ctrl Pts',(0.0812523240303111,0.0517064721460925,
-0.61405237149875));
#43471=CARTESIAN_POINT('Ctrl Pts',(0.000653148320722093,0.0963071794799973,
-0.607703481154105));
#43472=CARTESIAN_POINT('Ctrl Pts',(-0.0805435432000787,0.0528037600072041,
-0.60135459080946));
#43473=CARTESIAN_POINT('Ctrl Pts',(-0.0880570619618391,-0.0390058106026548,
-0.595005700464814));
#43474=CARTESIAN_POINT('Ctrl Pts',(-0.0150138600803315,-0.0951319264369724,
-0.588656810120169));
#43475=CARTESIAN_POINT('Ctrl Pts',(0.0717643825272961,-0.0642290652477304,
-0.582307919775524));
#43476=CARTESIAN_POINT('Ctrl Pts',(0.0928908399562031,0.025432091427022,
-0.575959029430878));
#43477=CARTESIAN_POINT('Ctrl Pts',(0.029038520238159,0.0918273584750176,
-0.569610139086234));
#43478=CARTESIAN_POINT('Ctrl Pts',(-0.0613789370236857,0.0742167468430388,
-0.563261248741587));
#43479=CARTESIAN_POINT('Ctrl Pts',(-0.095645464728733,-0.0112891318951454,
-0.556912358396944));
#43480=CARTESIAN_POINT('Ctrl Pts',(-0.0424132182152278,-0.0864674409402106,
-0.550563468052297));
#43481=CARTESIAN_POINT('Ctrl Pts',(0.0496196616061063,-0.0825432529297025,
-0.544214577707653));
#43482=CARTESIAN_POINT('Ctrl Pts',(0.0962592801788553,-0.00310650954769815,
-0.537865687363006));
#43483=CARTESIAN_POINT('Ctrl Pts',(0.0548385913789765,0.0791721435714039,
-0.531516797018362));
#43484=CARTESIAN_POINT('Ctrl Pts',(-0.0367497612943688,0.0890222133342473,
-0.525167906673716));
#43485=CARTESIAN_POINT('Ctrl Pts',(-0.0947185474236903,0.0174326187380849,
-0.518819016329072));
#43486=CARTESIAN_POINT('Ctrl Pts',(-0.0660365256047182,-0.0701047552465502,
-0.512470125984425));
#43487=CARTESIAN_POINT('Ctrl Pts',(0.0230572999568844,-0.0935086110517078,
-0.506121235639781));
#43488=CARTESIAN_POINT('Ctrl Pts',(0.0910577523121486,-0.0313685378361942,
-0.499772345295134));
#43489=CARTESIAN_POINT('Ctrl Pts',(0.0757563802368799,0.0594682291272118,
-0.493423454950491));
#43490=CARTESIAN_POINT('Ctrl Pts',(-0.00884875264671714,0.0959020281262003,
-0.487074564605844));
#43491=CARTESIAN_POINT('Ctrl Pts',(-0.0853588335365077,0.0446023425327426,
-0.4807256742612));
#43492=CARTESIAN_POINT('Ctrl Pts',(-0.0837805981182255,-0.0475006400069908,
-0.474376783916553));
#43493=CARTESIAN_POINT('Ctrl Pts',(-0.0055578541554653,-0.0961488932817632,
-0.468027893571909));
#43494=CARTESIAN_POINT('Ctrl Pts',(0.0777493486184669,-0.0568378237754173,
-0.461679003227264));
#43495=CARTESIAN_POINT('Ctrl Pts',(0.0899295751191266,0.0344698555409609,
-0.455330112882618));
#43496=CARTESIAN_POINT('Ctrl Pts',(0.019840060851252,0.0942436809952789,
-0.448981222537974));
#43497=CARTESIAN_POINT('Ctrl Pts',(-0.0683996188199645,0.0678011177445095,
-0.442632332193327));
#43498=CARTESIAN_POINT('Ctrl Pts',(-0.0940656801733943,-0.0206675406286791,
-0.436283441848683));
#43499=CARTESIAN_POINT('Ctrl Pts',(-0.0336781922597468,-0.0902290351729243,
-0.429934551504037));
#43500=CARTESIAN_POINT('Ctrl Pts',(0.0575189168835339,-0.0772468356806051,
-0.423585661159392));
#43501=CARTESIAN_POINT('Ctrl Pts',(0.0960963358411698,0.00640262914922511,
-0.417236770814747));
#43502=CARTESIAN_POINT('Ctrl Pts',(0.0467625128298921,0.0841948146619225,
-0.410887880470101));
#43503=CARTESIAN_POINT('Ctrl Pts',(-0.0453507829310814,0.084963556361885,
-0.404538990125456));
#43504=CARTESIAN_POINT('Ctrl Pts',(-0.0959760904473898,0.00800559083115412,
-0.398190099780811));
#43505=CARTESIAN_POINT('Ctrl Pts',(-0.0588001593764506,-0.0762760819616825,
-0.391841209436166));
#43506=CARTESIAN_POINT('Ctrl Pts',(0.0321675733641939,-0.0907785582942382,
-0.38549231909152));
#43507=CARTESIAN_POINT('Ctrl Pts',(0.0937076354156433,-0.0222346236066698,
-0.379143428746875));
#43508=CARTESIAN_POINT('Ctrl Pts',(0.0695216961659067,0.0666500801525155,
-0.37279453840223));
#43509=CARTESIAN_POINT('Ctrl Pts',(-0.0182643647766261,0.0945616856947227,
-0.366445648057585));
#43510=CARTESIAN_POINT('Ctrl Pts',(-0.0893417450266884,0.0359659841754329,
-0.360096757712939));
#43511=CARTESIAN_POINT('Ctrl Pts',(-0.078687145631372,-0.0555322657066021,
-0.353747867368294));
#43512=CARTESIAN_POINT('Ctrl Pts',(0.00395234932620661,-0.0962282617370018,
-0.347398977023649));
#43513=CARTESIAN_POINT('Ctrl Pts',(0.0829761399499992,-0.0488923268122867,
-0.341050086679003));
#43514=CARTESIAN_POINT('Ctrl Pts',(0.0860913597324722,0.0431714859778473,
-0.334701196334359));
#43515=CARTESIAN_POINT('Ctrl Pts',(0.0104481306040173,0.0957409838522809,
-0.328352305989713));
#43516=CARTESIAN_POINT('Ctrl Pts',(-0.0747532999856318,0.0607243243138976,
-0.322003415645068));
#43517=CARTESIAN_POINT('Ctrl Pts',(-0.0915686117343578,-0.0298444093116925,
-0.315654525300423));
#43518=CARTESIAN_POINT('Ctrl Pts',(-0.0246147525519286,-0.0931107586636937,
-0.309305634955777));
#43519=CARTESIAN_POINT('Ctrl Pts',(0.0648572749732974,-0.0711971439396228,
-0.302956744611133));
#43520=CARTESIAN_POINT('Ctrl Pts',(0.0949963056291566,0.0158493324444051,
-0.296607854266486));
#43521=CARTESIAN_POINT('Ctrl Pts',(0.0382304284421113,0.088396457865991,
-0.290258963921842));
#43522=CARTESIAN_POINT('Ctrl Pts',(-0.053509565249277,0.0800763750987432,
-0.283910073577196));
#43523=CARTESIAN_POINT('Ctrl Pts',(-0.0962977201727911,-0.00149950379931796,
-0.277561183232552));
#43524=CARTESIAN_POINT('Ctrl Pts',(-0.0509904018916127,-0.0817036005146229,
-0.271212292887905));
#43525=CARTESIAN_POINT('Ctrl Pts',(0.040964163857924,-0.0871632761060666,
-0.264863402543261));
#43526=CARTESIAN_POINT('Ctrl Pts',(0.0954437261180456,-0.0128838878769242,
-0.258514512198614));
#43527=CARTESIAN_POINT('Ctrl Pts',(0.0626090694984084,0.073181991218226,
-0.25216562185397));
#43528=CARTESIAN_POINT('Ctrl Pts',(-0.0275018714867341,0.0922992225690327,
-0.245816731509324));
#43529=CARTESIAN_POINT('Ctrl Pts',(-0.09245343820747,0.0269789026044658,
-0.239467841164679));
#43530=CARTESIAN_POINT('Ctrl Pts',(-0.0728263734333226,-0.0630223670982701,
-0.233118950820034));
#43531=CARTESIAN_POINT('Ctrl Pts',(0.0134240113723944,-0.0953692578391558,
-0.226770060475389));
#43532=CARTESIAN_POINT('Ctrl Pts',(0.0873937873327554,-0.040470055075016,
-0.220421170130743));
#43533=CARTESIAN_POINT('Ctrl Pts',(0.0814136222514969,0.0514521285661883,
-0.214072279786098));
#43534=CARTESIAN_POINT('Ctrl Pts',(0.00095431514453144,0.0963046660588629,
-0.207723389441453));
#43535=CARTESIAN_POINT('Ctrl Pts',(-0.080378022437017,0.0530553760833366,
-0.201374499096808));
#43536=CARTESIAN_POINT('Ctrl Pts',(-0.0881786096372469,-0.0387302494750746,
-0.195025608752162));
#43537=CARTESIAN_POINT('Ctrl Pts',(-0.0153112814576817,-0.0950845102116404,
-0.188676718407517));
#43538=CARTESIAN_POINT('Ctrl Pts',(0.0715631756928054,-0.0644531714315326,
-0.182327828062872));
#43539=CARTESIAN_POINT('Ctrl Pts',(0.0929699165082818,0.0251414805715377,
-0.175978937718227));
#43540=CARTESIAN_POINT('Ctrl Pts',(0.0293255390683039,0.0917361007482732,
-0.169630047373581));
#43541=CARTESIAN_POINT('Ctrl Pts',(-0.0611465477008044,0.07440832702589,
-0.163281157028936));
#43542=CARTESIAN_POINT('Ctrl Pts',(-0.0956803001699257,-0.0109899759955527,
-0.156932266684291));
#43543=CARTESIAN_POINT('Ctrl Pts',(-0.0426834102937165,-0.0863343842903646,
-0.150583376339646));
#43544=CARTESIAN_POINT('Ctrl Pts',(0.0493612914391104,-0.0826980190591283,
-0.144234485995));
#43545=CARTESIAN_POINT('Ctrl Pts',(0.0962490945489212,-0.00340751448045925,
-0.137885595650355));
#43546=CARTESIAN_POINT('Ctrl Pts',(0.0550859095302308,0.079000266027756,
-0.13153670530571));
#43547=CARTESIAN_POINT('Ctrl Pts',(-0.0364711942086585,0.0891367015934007,
-0.125187814961065));
#43548=CARTESIAN_POINT('Ctrl Pts',(-0.0946635670202091,0.0177287348598427,
-0.118838924616419));
#43549=CARTESIAN_POINT('Ctrl Pts',(-0.0662554373619121,-0.069897902909749,
-0.112490034271774));
#43550=CARTESIAN_POINT('Ctrl Pts',(0.0227647771129189,-0.0935802607606224,
-0.106141143927129));
#43551=CARTESIAN_POINT('Ctrl Pts',(0.0909591962535613,-0.0316531336799535,
-0.0997922535824833));
#43552=CARTESIAN_POINT('Ctrl Pts',(0.0759420075516381,0.0592310251496444,
-0.0934433632378381));
#43553=CARTESIAN_POINT('Ctrl Pts',(-0.00854886285930021,0.0959292484132404,
-0.0870944728931927));
#43554=CARTESIAN_POINT('Ctrl Pts',(-0.0852188293617118,0.0448690236940463,
-0.0807455825485475));
#43555=CARTESIAN_POINT('Ctrl Pts',(-0.0839289348648598,-0.0472383474586548,
-0.0743966922039022));
#43556=CARTESIAN_POINT('Ctrl Pts',(-0.00585811645465809,-0.096131162521779,
-0.068047801859257));
#43557=CARTESIAN_POINT('Ctrl Pts',(0.0775704950346791,-0.0570804549773756,
-0.0616989115146119));
#43558=CARTESIAN_POINT('Ctrl Pts',(0.0900383157362904,0.0341880300064409,
-0.0553500211699665));
#43559=CARTESIAN_POINT('Ctrl Pts',(0.0201320506167284,0.0941819939552226,
-0.0490011308253214));
#43560=CARTESIAN_POINT('Ctrl Pts',(-0.0681822691654502,0.0680131341533761,
-0.042652240480676));
#43561=CARTESIAN_POINT('Ctrl Pts',(-0.0941393148464921,-0.0203703384015287,
-0.0363033501360307));
#43562=CARTESIAN_POINT('Ctrl Pts',(-0.0339422270357189,-0.0901288607981892,
-0.0299544597913855));
#43563=CARTESIAN_POINT('Ctrl Pts',(0.0572428774412662,-0.0774156769940841,
-0.0236055694467402));
#43564=CARTESIAN_POINT('Ctrl Pts',(0.0961817888891786,0.00608136681561371,
-0.0172566791020948));
#43565=CARTESIAN_POINT('Ctrl Pts',(0.0468917811787354,0.0840917490061967,
-0.0109077887574496));
#43566=CARTESIAN_POINT('Ctrl Pts',(-0.0142098698468084,0.0846926301986895,
-0.00667519519435273));
#43567=CARTESIAN_POINT('Ctrl Pts',(-0.0381483114577586,0.0720110968464789,
-0.00455889841280429));
#43568=CARTESIAN_POINT('Ctrl Pts',(-0.0601104350279426,-0.0429877377952305,
-1.149325));
#43569=CARTESIAN_POINT('Ctrl Pts',(-0.0458201451106566,-0.0629700766588213,
-1.14720870321845));
#43570=CARTESIAN_POINT('Ctrl Pts',(0.00400364749018219,-0.0872208216030551,
-1.14297610965536));
#43571=CARTESIAN_POINT('Ctrl Pts',(0.075583875527885,-0.0438759620050528,
-1.13662721931071));
#43572=CARTESIAN_POINT('Ctrl Pts',(0.0777927499997916,0.0396423987382078,
-1.13027832896607));
#43573=CARTESIAN_POINT('Ctrl Pts',(0.00894843417834478,0.0868766870214709,
-1.12392943862142));
#43574=CARTESIAN_POINT('Ctrl Pts',(-0.0681413246659313,0.0546437095181167,
-1.11758054827678));
#43575=CARTESIAN_POINT('Ctrl Pts',(-0.0828626209147509,-0.0275837207699589,
-1.11123165793213));
#43576=CARTESIAN_POINT('Ctrl Pts',(-0.0217956051609413,-0.0845742251201784,
-1.10488276758748));
#43577=CARTESIAN_POINT('Ctrl Pts',(0.0592192057513427,-0.0641956017183869,
-1.09853387724284));
#43578=CARTESIAN_POINT('Ctrl Pts',(0.0860543001947688,0.0149114473055614,
-1.09218498689819));
#43579=CARTESIAN_POINT('Ctrl Pts',(0.0341672535616166,0.0803767533194929,
-1.08583609655355));
#43580=CARTESIAN_POINT('Ctrl Pts',(-0.0489780873575578,0.0723116766374376,
-1.0794872062089));
#43581=CARTESIAN_POINT('Ctrl Pts',(-0.0873164260293921,-0.00190597202016384,
-1.07313831586426));
#43582=CARTESIAN_POINT('Ctrl Pts',(-0.0457759481553394,-0.074379934125127,
-1.06678942551961));
#43583=CARTESIAN_POINT('Ctrl Pts',(0.037641655214997,-0.0788093717621258,
-1.06044053517497));
#43584=CARTESIAN_POINT('Ctrl Pts',(0.0866236680057719,-0.0111420824567537,
-1.05409164483032));
#43585=CARTESIAN_POINT('Ctrl Pts',(0.0563603151316931,0.0667182437528911,
-1.04774275448568));
#43586=CARTESIAN_POINT('Ctrl Pts',(-0.0254628383918398,0.0835431184830735,
-1.04139386414103));
#43587=CARTESIAN_POINT('Ctrl Pts',(-0.0839919598596433,0.0239407344160811,
-1.03504497379639));
#43588=CARTESIAN_POINT('Ctrl Pts',(-0.0656832215466922,-0.0575632087386073,
-1.02869608345174));
#43589=CARTESIAN_POINT('Ctrl Pts',(0.0127141134428745,-0.0864069431030045,
-1.0223471931071));
#43590=CARTESIAN_POINT('Ctrl Pts',(0.0794802692010834,-0.0362035249468621,
-1.01599830276245));
#43591=CARTESIAN_POINT('Ctrl Pts',(0.0735359619677752,0.0471197494086118,
-1.0096494124178));
#43592=CARTESIAN_POINT('Ctrl Pts',(0.000319185439644519,0.0873367424855461,
-1.00330052207316));
#43593=CARTESIAN_POINT('Ctrl Pts',(-0.0731895893058077,0.0476559804706753,
-0.996951631728512));
#43594=CARTESIAN_POINT('Ctrl Pts',(-0.0797427655561862,-0.0356216199793146,
-0.990602741383869));
#43595=CARTESIAN_POINT('Ctrl Pts',(-0.0133453396325877,-0.0863117047392357,
-0.984253851039223));
#43596=CARTESIAN_POINT('Ctrl Pts',(0.0652607242893321,-0.0580417636628946,
-0.977904960694579));
#43597=CARTESIAN_POINT('Ctrl Pts',(0.0841647062166166,0.0233261804187959,
-0.971556070349931));
#43598=CARTESIAN_POINT('Ctrl Pts',(0.0260727882493475,0.0833547729751633,
-0.965207180005289));
#43599=CARTESIAN_POINT('Ctrl Pts',(-0.0558711442187008,0.0671284120804557,
-0.958858289660641));
#43600=CARTESIAN_POINT('Ctrl Pts',(-0.0867028086157542,-0.0105086365962801,
-0.952509399315998));
#43601=CARTESIAN_POINT('Ctrl Pts',(-0.0382166559382933,-0.0785321314734518,
-0.946160508971351));
#43602=CARTESIAN_POINT('Ctrl Pts',(0.0452310138244137,-0.0747125414725162,
-0.939811618626707));
#43603=CARTESIAN_POINT('Ctrl Pts',(0.087300263005714,-0.00254411949997818,
-0.933462728282061));
#43604=CARTESIAN_POINT('Ctrl Pts',(0.0495051294517987,0.0719517242520363,
-0.927113837937416));
#43605=CARTESIAN_POINT('Ctrl Pts',(-0.0335784885779334,0.0806243981044391,
-0.920764947592771));
#43606=CARTESIAN_POINT('Ctrl Pts',(-0.0859436967070338,0.0155399311843679,
-0.914416057248125));
#43607=CARTESIAN_POINT('Ctrl Pts',(-0.0596855416164745,-0.0637608389752754,
-0.908067166903481));
#43608=CARTESIAN_POINT('Ctrl Pts',(0.0211743841364114,-0.0847316583180511,
-0.901718276558834));
#43609=CARTESIAN_POINT('Ctrl Pts',(0.0826634734150078,-0.0281879163445984,
-0.89536938621419));
#43610=CARTESIAN_POINT('Ctrl Pts',(0.0685300267273087,0.0541428102488016,
-0.889020495869544));
#43611=CARTESIAN_POINT('Ctrl Pts',(-0.00829633857195642,0.0869423903006062,
-0.882671605524899));
#43612=CARTESIAN_POINT('Ctrl Pts',(-0.0775330135748029,0.0402049781854557,
-0.876322715180253));
#43613=CARTESIAN_POINT('Ctrl Pts',(-0.0758406208115356,-0.043312916085209,
-0.86997382483561));
#43614=CARTESIAN_POINT('Ctrl Pts',(-0.00476740193378281,-0.087207111772408,
-0.863624934490961));
#43615=CARTESIAN_POINT('Ctrl Pts',(0.0706671510291381,-0.0513221417159152,
-0.857276044146319));
#43616=CARTESIAN_POINT('Ctrl Pts',(0.0814536926085207,0.0315135593883026,
-0.850927153801671));
#43617=CARTESIAN_POINT('Ctrl Pts',(0.0177244348341756,0.0855198975367287,
-0.844578263457028));
#43618=CARTESIAN_POINT('Ctrl Pts',(-0.0622195627201011,0.0612905741513564,
-0.838229373112381));
#43619=CARTESIAN_POINT('Ctrl Pts',(-0.0852436060887428,-0.0190088423074822,
-0.831880482767737));
#43620=CARTESIAN_POINT('Ctrl Pts',(-0.0302847459931343,-0.081918512102057,
-0.825531592423091));
#43621=CARTESIAN_POINT('Ctrl Pts',(0.0523793289752858,-0.0698871544776452,
-0.819182702078447));
#43622=CARTESIAN_POINT('Ctrl Pts',(0.0871255325346814,0.00607865490315511,
-0.812833811733801));
#43623=CARTESIAN_POINT('Ctrl Pts',(0.0421672010014363,0.0764835644082308,
-0.806484921389155));
#43624=CARTESIAN_POINT('Ctrl Pts',(-0.041366701368516,0.0769194675148722,
-0.800136031044511));
#43625=CARTESIAN_POINT('Ctrl Pts',(-0.0870573492415018,0.0069875895648422,
-0.793787140699864));
#43626=CARTESIAN_POINT('Ctrl Pts',(-0.0531058377402594,-0.0693367035760193,
-0.787438250355221));
#43627=CARTESIAN_POINT('Ctrl Pts',(0.0294281728820954,-0.0822301106998219,
-0.781089360010573));
#43628=CARTESIAN_POINT('Ctrl Pts',(0.0850405823393773,-0.0198974325042983,
-0.77474046966593));
#43629=CARTESIAN_POINT('Ctrl Pts',(0.0628558193470167,0.0606378960642491,
-0.768391579321283));
#43630=CARTESIAN_POINT('Ctrl Pts',(-0.0168309607139535,0.0857002171895078,
-0.762042688976639));
#43631=CARTESIAN_POINT('Ctrl Pts',(-0.0811203726344865,0.0323619160206188,
-0.755693798631993));
#43632=CARTESIAN_POINT('Ctrl Pts',(-0.0711989143396801,-0.0505818451792178,
-0.749344908287349));
#43633=CARTESIAN_POINT('Ctrl Pts',(0.00385702521968538,-0.0872521164289911,
-0.742996017942701));
#43634=CARTESIAN_POINT('Ctrl Pts',(0.0753844652332581,-0.0441020505915453,
-0.736647127598059));
#43635=CARTESIAN_POINT('Ctrl Pts',(0.0779483812393019,0.0393936330776424,
-0.730298237253411));
#43636=CARTESIAN_POINT('Ctrl Pts',(0.00920324113794826,0.086851072632641,
-0.723949346908768));
#43637=CARTESIAN_POINT('Ctrl Pts',(-0.0679612455648586,0.0548550596222128,
-0.717600456564122));
#43638=CARTESIAN_POINT('Ctrl Pts',(-0.0829531483594101,-0.0273236828071396,
-0.711251566219477));
#43639=CARTESIAN_POINT('Ctrl Pts',(-0.0220575135733365,-0.0845060622668312,
-0.704902675874831));
#43640=CARTESIAN_POINT('Ctrl Pts',(0.0590168657611575,-0.064380261110165,
-0.698553785530186));
#43641=CARTESIAN_POINT('Ctrl Pts',(0.0861011952070565,0.0146421531476717,
-0.692204895185541));
#43642=CARTESIAN_POINT('Ctrl Pts',(0.0344180780130461,0.080269573131862,
-0.685856004840895));
#43643=CARTESIAN_POINT('Ctrl Pts',(-0.0487515257137156,0.0724644547724496,
-0.679507114496251));
#43644=CARTESIAN_POINT('Ctrl Pts',(-0.0873220598104371,-0.00163289171286479,
-0.673158224151604));
#43645=CARTESIAN_POINT('Ctrl Pts',(-0.0460082709303986,-0.0742364295402099,
-0.66680933380696));
#43646=CARTESIAN_POINT('Ctrl Pts',(0.037394992047993,-0.0789266940560291,
-0.660460443462315));
#43647=CARTESIAN_POINT('Ctrl Pts',(0.0865884158521809,-0.0114129183425305,
-0.654111553117668));
#43648=CARTESIAN_POINT('Ctrl Pts',(0.0565686718383231,0.0665416698868583,
-0.647762662773025));
#43649=CARTESIAN_POINT('Ctrl Pts',(-0.0252014553124982,0.0836223362207471,
-0.641413772428377));
#43650=CARTESIAN_POINT('Ctrl Pts',(-0.0839166843077061,0.0242032758048216,
-0.635064882083734));
#43651=CARTESIAN_POINT('Ctrl Pts',(-0.0658629098354269,-0.0573575241175375,
-0.628715991739088));
#43652=CARTESIAN_POINT('Ctrl Pts',(0.0124438404931729,-0.0864462798428249,
-0.622367101394442));
#43653=CARTESIAN_POINT('Ctrl Pts',(0.0793666658984961,-0.0364518971939734,
-0.616018211049798));
#43654=CARTESIAN_POINT('Ctrl Pts',(0.073682954238757,0.0468895587474729,
-0.609669320705152));
#43655=CARTESIAN_POINT('Ctrl Pts',(0.000592301800611145,0.087335317274631,
-0.603320430360507));
#43656=CARTESIAN_POINT('Ctrl Pts',(-0.0730402025870019,0.0478846245775535,
-0.596971540015862));
#43657=CARTESIAN_POINT('Ctrl Pts',(-0.0798537708843025,-0.0353720757157512,
-0.590622649671216));
#43658=CARTESIAN_POINT('Ctrl Pts',(-0.0136151867463331,-0.0862695494061835,
-0.584273759326571));
#43659=CARTESIAN_POINT('Ctrl Pts',(0.06507889807261,-0.058245561981479,
-0.577924868981926));
#43660=CARTESIAN_POINT('Ctrl Pts',(0.0842372398743852,0.0230628680616442,
-0.57157597863728));
#43661=CARTESIAN_POINT('Ctrl Pts',(0.0263333262574912,0.083272831062118,
-0.565227088292636));
#43662=CARTESIAN_POINT('Ctrl Pts',(-0.0556609483102603,0.0673028030477632,
-0.55887819794799));
#43663=CARTESIAN_POINT('Ctrl Pts',(-0.0867352470819517,-0.010237449805311,
-0.552529307603345));
#43664=CARTESIAN_POINT('Ctrl Pts',(-0.0384620532909962,-0.0784122370649128,
-0.5461804172587));
#43665=CARTESIAN_POINT('Ctrl Pts',(0.0449971529934493,-0.0748536217384812,
-0.539831526914054));
#43666=CARTESIAN_POINT('Ctrl Pts',(0.0872918802153685,-0.00281711081593204,
-0.533482636569409));
#43667=CARTESIAN_POINT('Ctrl Pts',(0.0497298934808031,0.0717965609153495,
-0.527133746224764));
#43668=CARTESIAN_POINT('Ctrl Pts',(-0.0333261972756367,0.0807290099036824,
-0.520784855880119));
#43669=CARTESIAN_POINT('Ctrl Pts',(-0.0858946802897314,0.0158086167265926,
-0.514435965535473));
#43670=CARTESIAN_POINT('Ctrl Pts',(-0.0598846414830402,-0.0635738796938743,
-0.508087075190828));
#43671=CARTESIAN_POINT('Ctrl Pts',(0.0209093093381367,-0.0847974601499693,
-0.501738184846182));
#43672=CARTESIAN_POINT('Ctrl Pts',(0.0825749204933152,-0.0284462821895266,
-0.495389294501537));
#43673=CARTESIAN_POINT('Ctrl Pts',(0.0686990060272686,0.0539282396870952,
-0.489040404156892));
#43674=CARTESIAN_POINT('Ctrl Pts',(-0.00802441338286892,0.0869679093386998,
-0.482691513812247));
#43675=CARTESIAN_POINT('Ctrl Pts',(-0.0774069062073571,0.0404472413928185,
-0.476342623467602));
#43676=CARTESIAN_POINT('Ctrl Pts',(-0.0759756973220605,-0.0430755369242237,
-0.469993733122956));
#43677=CARTESIAN_POINT('Ctrl Pts',(-0.0050400910778892,-0.0871917768302152,
-0.463644842778311));
#43678=CARTESIAN_POINT('Ctrl Pts',(0.070506311846667,-0.0515428797668893,
-0.457295952433666));
#43679=CARTESIAN_POINT('Ctrl Pts',(0.0815518429447203,0.0312586848284312,
-0.45094706208902));
#43680=CARTESIAN_POINT('Ctrl Pts',(0.0179917843980893,0.0854640518525547,
-0.444598171744375));
#43681=CARTESIAN_POINT('Ctrl Pts',(-0.0620275917471557,0.0614848463194927,
-0.43824928139973));
#43682=CARTESIAN_POINT('Ctrl Pts',(-0.0853026333753618,-0.0187421771444026,
-0.431900391055085));
#43683=CARTESIAN_POINT('Ctrl Pts',(-0.0305407719561762,-0.0818234056563543,
-0.425551500710439));
#43684=CARTESIAN_POINT('Ctrl Pts',(0.0521605230517608,-0.0700506124159539,
-0.419202610365794));
#43685=CARTESIAN_POINT('Ctrl Pts',(0.0871441155782282,0.00580616783876835,
-0.412853720021149));
#43686=CARTESIAN_POINT('Ctrl Pts',(0.0424061727963488,0.0763513259455898,
-0.406504829676504));
#43687=CARTESIAN_POINT('Ctrl Pts',(-0.0411259579745188,0.0770484525838227,
-0.400155939331858));
#43688=CARTESIAN_POINT('Ctrl Pts',(-0.0870350721022039,0.00725979951842593,
-0.393807048987213));
#43689=CARTESIAN_POINT('Ctrl Pts',(-0.0533224065191096,-0.0691702929579908,
-0.387458158642567));
#43690=CARTESIAN_POINT('Ctrl Pts',(0.0291708805188321,-0.082321735857788,
-0.381109268297923));
#43691=CARTESIAN_POINT('Ctrl Pts',(0.0849779436410596,-0.0201632725374741,
-0.374760377953277));
#43692=CARTESIAN_POINT('Ctrl Pts',(0.0630451377031669,0.0604410380194803,
-0.368411487608632));
#43693=CARTESIAN_POINT('Ctrl Pts',(-0.0165628782942129,0.0857524316127216,
-0.362062597263987));
#43694=CARTESIAN_POINT('Ctrl Pts',(-0.0810187744039951,0.0326154359001687,
-0.355713706919342));
#43695=CARTESIAN_POINT('Ctrl Pts',(-0.0713567448061166,-0.0503589459337495,
-0.349364816574696));
#43696=CARTESIAN_POINT('Ctrl Pts',(0.00358415316748011,-0.0872637514146367,
-0.343015926230051));
#43697=CARTESIAN_POINT('Ctrl Pts',(0.0752461815192336,-0.0443375758432733,
-0.336667035885405));
#43698=CARTESIAN_POINT('Ctrl Pts',(0.0780711911348368,0.0391496817314182,
-0.330318145540761));
#43699=CARTESIAN_POINT('Ctrl Pts',(0.00947479519341831,0.0868218677576465,
-0.323969255196115));
#43700=CARTESIAN_POINT('Ctrl Pts',(-0.0677893715382528,0.0550673185413288,
-0.31762036485147));
#43701=CARTESIAN_POINT('Ctrl Pts',(-0.0830381888598311,-0.0270641396641863,
-0.311271474506825));
#43702=CARTESIAN_POINT('Ctrl Pts',(-0.0223216715032739,-0.0844366712168558,
-0.304922584162179));
#43703=CARTESIAN_POINT('Ctrl Pts',(0.0588152484367718,-0.0645645027565787,
-0.298573693817534));
#43704=CARTESIAN_POINT('Ctrl Pts',(0.0861465628713941,0.0143728274994348,
-0.292224803472889));
#43705=CARTESIAN_POINT('Ctrl Pts',(0.0346689272343444,0.0801615490700074,
-0.285875913128243));
#43706=CARTESIAN_POINT('Ctrl Pts',(-0.0485246778433969,0.0726165553099154,
-0.279527022783598));
#43707=CARTESIAN_POINT('Ctrl Pts',(-0.0873267391852247,-0.00135981181024029,
-0.273178132438953));
#43708=CARTESIAN_POINT('Ctrl Pts',(-0.04624019674556,-0.074092190342946,
-0.266829242094308));
#43709=CARTESIAN_POINT('Ctrl Pts',(0.0371479911127987,-0.0790432490549754,
-0.260480351749662));
#43710=CARTESIAN_POINT('Ctrl Pts',(0.0865523022001051,-0.0116836402180771,
-0.254131461405018));
#43711=CARTESIAN_POINT('Ctrl Pts',(0.0567764831078735,0.0663644440252806,
-0.247782571060372));
#43712=CARTESIAN_POINT('Ctrl Pts',(-0.0249398298746646,0.083700736858798,
-0.241433680715727));
#43713=CARTESIAN_POINT('Ctrl Pts',(-0.0838405859519216,0.0244655801509781,
-0.235084790371081));
#43714=CARTESIAN_POINT('Ctrl Pts',(-0.0660419551699266,-0.0571512783952807,
-0.228735900026436));
#43715=CARTESIAN_POINT('Ctrl Pts',(0.0121734464516189,-0.0864847712974369,
-0.222387009681791));
#43716=CARTESIAN_POINT('Ctrl Pts',(0.0792522861301636,-0.0366999129159682,
-0.216038119337145));
#43717=CARTESIAN_POINT('Ctrl Pts',(0.0738292261096514,0.046658909512726,
-0.2096892289925));
#43718=CARTESIAN_POINT('Ctrl Pts',(0.000865412281594935,0.0873330380008177,
-0.203340338647855));
#43719=CARTESIAN_POINT('Ctrl Pts',(-0.0728901015412066,0.0481128003995335,
-0.19699144830321));
#43720=CARTESIAN_POINT('Ctrl Pts',(-0.0799639953229482,-0.0351221855348143,
-0.190642557958564));
#43721=CARTESIAN_POINT('Ctrl Pts',(-0.0138849007021918,-0.0862265504199637,
-0.184293667613919));
#43722=CARTESIAN_POINT('Ctrl Pts',(0.0648964354273228,-0.058448790699953,
-0.177944777269274));
#43723=CARTESIAN_POINT('Ctrl Pts',(0.0843089497489975,0.0227993301675411,
-0.171595886924629));
#43724=CARTESIAN_POINT('Ctrl Pts',(0.0265936067550599,0.0831900747965725,
-0.165246996579983));
#43725=CARTESIAN_POINT('Ctrl Pts',(-0.0554502081000843,0.0674765358488189,
-0.158898106235338));
#43726=CARTESIAN_POINT('Ctrl Pts',(-0.0867668372949077,-0.00996616291323742,
-0.152549215890693));
#43727=CARTESIAN_POINT('Ctrl Pts',(-0.0387070745970641,-0.0782915758141884,
-0.146200325546048));
#43728=CARTESIAN_POINT('Ctrl Pts',(0.0447628522836712,-0.0749939700395087,
-0.139851435201402));
#43729=CARTESIAN_POINT('Ctrl Pts',(0.087282643466595,-0.00309007448744508,
-0.133502544856757));
#43730=CARTESIAN_POINT('Ctrl Pts',(0.0499541717674709,0.071640695279081,
-0.127153654512112));
#43731=CARTESIAN_POINT('Ctrl Pts',(-0.0330735811680512,0.0808328325728891,
-0.120804764167467));
#43732=CARTESIAN_POINT('Ctrl Pts',(-0.085844821795195,0.0160771470229162,
-0.114455873822821));
#43733=CARTESIAN_POINT('Ctrl Pts',(-0.0600831596815059,-0.0633862974745522,
-0.108106983478176));
#43734=CARTESIAN_POINT('Ctrl Pts',(0.0206440375741234,-0.0848624350572862,
-0.101758093133531));
#43735=CARTESIAN_POINT('Ctrl Pts',(0.082485545799834,-0.0287043654232375,
-0.0954092027888854));
#43736=CARTESIAN_POINT('Ctrl Pts',(0.0688673405223371,0.0537131333497329,
-0.0890603124442403));
#43737=CARTESIAN_POINT('Ctrl Pts',(-0.00775246097108719,0.0869925938161997,
-0.0827114220995948));
#43738=CARTESIAN_POINT('Ctrl Pts',(-0.0772799446548373,0.0406890788545673,
-0.0763625317549497));
#43739=CARTESIAN_POINT('Ctrl Pts',(-0.0761102151939444,-0.0428376792374824,
-0.0700136414103042));
#43740=CARTESIAN_POINT('Ctrl Pts',(-0.00531238129869321,-0.0871756978467261,
-0.0636647510656592));
#43741=CARTESIAN_POINT('Ctrl Pts',(0.0703441200498545,-0.0517629077348786,
-0.057315860721014));
#43742=CARTESIAN_POINT('Ctrl Pts',(0.0816504534154235,0.0310031138252487,
-0.0509669703763687));
#43743=CARTESIAN_POINT('Ctrl Pts',(0.018256572744571,0.0854081115037233,
-0.0446180800317234));
#43744=CARTESIAN_POINT('Ctrl Pts',(-0.0618304901277434,0.0616771115320737,
-0.0382691896870782));
#43745=CARTESIAN_POINT('Ctrl Pts',(-0.0853694083299616,-0.0184726619229722,
-0.0319202993424328));
#43746=CARTESIAN_POINT('Ctrl Pts',(-0.0307802095667008,-0.0817325634071313,
-0.0255714089977876));
#43747=CARTESIAN_POINT('Ctrl Pts',(0.0519101991153633,-0.070203724673642,
-0.0192225186531423));
#43748=CARTESIAN_POINT('Ctrl Pts',(0.087221607922,0.0055148339217558,-0.012873628308497));
#43749=CARTESIAN_POINT('Ctrl Pts',(0.0425233986596825,0.0762578617636718,
-0.00652473796385174));
#43750=CARTESIAN_POINT('Ctrl Pts',(-0.0128860952859686,0.0768027655795051,
-0.00229214440075486));
#43751=CARTESIAN_POINT('Ctrl Pts',(-0.0345944601705076,0.0653026287794846,
-0.000175847619206415));
#43752=CARTESIAN_POINT('Ctrl Pts',(-0.0452560140322605,0.0854280329804675,
-0.013325));
#43753=CARTESIAN_POINT('Ctrl Pts',(-0.0168574189684875,0.100472359437059,
-0.0154412967815485));
#43754=CARTESIAN_POINT('Ctrl Pts',(0.0193855636241788,0.100115941464152,
-0.0175575935630971));
#43755=CARTESIAN_POINT('Ctrl Pts',(0.0472526556882942,0.084513550663045,
-0.0196738903446456));
#43756=CARTESIAN_POINT('Ctrl Pts',(0.0751197477524064,0.0689111598619393,
-0.0217901871261938));
#43757=CARTESIAN_POINT('Ctrl Pts',(0.0946109492879698,0.0380627962326364,
-0.0239064839077421));
#43758=CARTESIAN_POINT('Ctrl Pts',(0.0966575639340093,0.0061296120449364,
-0.0260227806892903));
#43759=CARTESIAN_POINT('Ctrl Pts',(0.0987041785800492,-0.0258035721427672,
-0.0281390774708388));
#43760=CARTESIAN_POINT('Ctrl Pts',(0.0833062063365607,-0.0588215768888681,
-0.0302553742523873));
#43761=CARTESIAN_POINT('Ctrl Pts',(0.0575781375370112,-0.0778442249194746,
-0.0323716710339359));
#43762=CARTESIAN_POINT('Ctrl Pts',(0.0318500687374624,-0.0968668729500805,
-0.0344879678154843));
#43763=CARTESIAN_POINT('Ctrl Pts',(-0.00420809661814683,-0.101894164265193,
-0.0366042645970328));
#43764=CARTESIAN_POINT('Ctrl Pts',(-0.0341393236135845,-0.0906151825524714,
-0.0387205613785813));
#43765=CARTESIAN_POINT('Ctrl Pts',(-0.0640705506090213,-0.0793362008397503,
-0.0408368581601297));
#43766=CARTESIAN_POINT('Ctrl Pts',(-0.0878748392442869,-0.0517509460991965,
-0.042953154941678));
#43767=CARTESIAN_POINT('Ctrl Pts',(-0.0946447667888051,-0.0204831736031495,
-0.0450694517232264));
#43768=CARTESIAN_POINT('Ctrl Pts',(-0.0960917122047474,-0.0138002719350931,
-0.0455217705858284));
#43769=CARTESIAN_POINT('Ctrl Pts',(-0.0967605098021332,-0.00694914892060837,
-0.0459740894484305));
#43770=CARTESIAN_POINT('Ctrl Pts',(-0.0966970977580488,-8.58596968723868E-5,
-0.0464264083110326));
#43771=CARTESIAN_POINT('Origin',(0.194007127343405,-0.0342086910003853,
0.04));
#43772=CARTESIAN_POINT('',(0.18738691397118,-0.0314029373205391,0.04));
#43773=CARTESIAN_POINT('',(0.186826537413779,-0.0345809907026646,0.04));
#43774=CARTESIAN_POINT('Origin',(0.,0.,0.04));
#43775=CARTESIAN_POINT('',(0.181204626554246,-0.0319512646907152,0.04));
#43776=CARTESIAN_POINT('',(0.208025165376232,-0.02957246303897,0.04));
#43777=CARTESIAN_POINT('',(0.181204626554246,-0.0319512646907152,0.04));
#43778=CARTESIAN_POINT('Origin',(0.181204626554246,-0.0319512646907152,
0.04));
#43779=CARTESIAN_POINT('',(0.186826537413779,-0.0345809907026646,0.185));
#43780=CARTESIAN_POINT('',(0.186826537413779,-0.0345809907026646,0.0925));
#43781=CARTESIAN_POINT('',(0.181204626554246,-0.0319512646907152,0.191));
#43782=CARTESIAN_POINT('',(0.181204626554246,-0.0319512646907152,0.04));
#43783=CARTESIAN_POINT('Ctrl Pts',(0.186826537413779,-0.0345809907026646,
0.185));
#43784=CARTESIAN_POINT('Ctrl Pts',(0.183970486442383,-0.033245033637782,
0.188051499118437));
#43785=CARTESIAN_POINT('Ctrl Pts',(0.181204626554246,-0.0319512646907152,
0.191));
#43786=CARTESIAN_POINT('Origin',(0.208025165376232,-0.02957246303897,0.04));
#43787=CARTESIAN_POINT('',(0.18738691397118,-0.0314029373205391,0.185));
#43788=CARTESIAN_POINT('',(0.18738691397118,-0.0314029373205391,0.0925));
#43789=CARTESIAN_POINT('Ctrl Pts',(0.181204626554246,-0.0319512646907152,
0.191));
#43790=CARTESIAN_POINT('Ctrl Pts',(0.18424617972193,-0.0316814993535168,
0.188051499118469));
#43791=CARTESIAN_POINT('Ctrl Pts',(0.18738691397118,-0.0314029373205392,
0.185));
#43792=CARTESIAN_POINT('Origin',(0.185119446294824,-0.0673779682351569,
0.04));
#43793=CARTESIAN_POINT('',(0.179087022852749,-0.0634652522703487,0.04));
#43794=CARTESIAN_POINT('',(0.17798329649608,-0.0664977155125527,0.04));
#43795=CARTESIAN_POINT('Origin',(0.,0.,0.04));
#43796=CARTESIAN_POINT('',(0.172903442224607,-0.0629317063719232,0.04));
#43797=CARTESIAN_POINT('',(0.19972959136832,-0.0652463817528892,0.04));
#43798=CARTESIAN_POINT('',(0.172903442224607,-0.0629317063719232,0.04));
#43799=CARTESIAN_POINT('Origin',(0.172903442224607,-0.0629317063719232,
0.04));
#43800=CARTESIAN_POINT('',(0.17798329649608,-0.0664977155125527,0.185));
#43801=CARTESIAN_POINT('',(0.17798329649608,-0.0664977155125527,0.0925));
#43802=CARTESIAN_POINT('',(0.172903442224607,-0.0629317063719232,0.191));
#43803=CARTESIAN_POINT('',(0.172903442224607,-0.0629317063719232,0.04));
#43804=CARTESIAN_POINT('Ctrl Pts',(0.17798329649608,-0.0664977155125527,
0.185));
#43805=CARTESIAN_POINT('Ctrl Pts',(0.17540262186618,-0.0646861065908373,
0.188051499118472));
#43806=CARTESIAN_POINT('Ctrl Pts',(0.172903442224607,-0.0629317063719232,
0.191));
#43807=CARTESIAN_POINT('Origin',(0.19972959136832,-0.0652463817528892,0.04));
#43808=CARTESIAN_POINT('',(0.179087022852749,-0.0634652522703487,0.185));
#43809=CARTESIAN_POINT('',(0.179087022852749,-0.0634652522703487,0.0925));
#43810=CARTESIAN_POINT('Ctrl Pts',(0.172903442224607,-0.0629317063719232,
0.191));
#43811=CARTESIAN_POINT('Ctrl Pts',(0.17594563162456,-0.063194199541203,
0.188051499118452));
#43812=CARTESIAN_POINT('Ctrl Pts',(0.179087022852749,-0.0634652522703487,
0.185));
#43813=CARTESIAN_POINT('Origin',(0.170607004545534,-0.0985000000000001,
0.04));
#43814=CARTESIAN_POINT('',(0.165345663167344,-0.0935992076448907,0.04));
#43815=CARTESIAN_POINT('',(0.163732123178242,-0.0963939408860593,0.04));
#43816=CARTESIAN_POINT('Origin',(0.,0.,0.04));
#43817=CARTESIAN_POINT('',(0.159348674296337,-0.0920000000000001,0.04));
#43818=CARTESIAN_POINT('',(0.185365334794732,-0.098937822173509,0.04));
#43819=CARTESIAN_POINT('',(0.159348674296337,-0.0920000000000001,0.04));
#43820=CARTESIAN_POINT('Origin',(0.159348674296337,-0.0920000000000001,
0.04));
#43821=CARTESIAN_POINT('',(0.163732123178242,-0.0963939408860593,0.185));
#43822=CARTESIAN_POINT('',(0.163732123178242,-0.0963939408860593,0.0925));
#43823=CARTESIAN_POINT('',(0.159348674296337,-0.0920000000000001,0.191));
#43824=CARTESIAN_POINT('',(0.159348674296337,-0.0920000000000001,0.04));
#43825=CARTESIAN_POINT('Ctrl Pts',(0.163732123178242,-0.0963939408860593,
0.185));
#43826=CARTESIAN_POINT('Ctrl Pts',(0.161505237382642,-0.0941617249279212,
0.188051499118436));
#43827=CARTESIAN_POINT('Ctrl Pts',(0.159348674296337,-0.0920000000000001,
0.191));
#43828=CARTESIAN_POINT('Origin',(0.185365334794732,-0.098937822173509,0.04));
#43829=CARTESIAN_POINT('',(0.165345663167344,-0.0935992076448907,0.185));
#43830=CARTESIAN_POINT('',(0.165345663167344,-0.0935992076448907,0.0925));
#43831=CARTESIAN_POINT('Ctrl Pts',(0.159348674296337,-0.0920000000000001,
0.191));
#43832=CARTESIAN_POINT('Ctrl Pts',(0.162299064543036,-0.0927867759536363,
0.188051499118462));
#43833=CARTESIAN_POINT('Ctrl Pts',(0.165345663167344,-0.0935992076448907,
0.185));
#43834=CARTESIAN_POINT('Origin',(0.150910755294439,-0.126629159108248,0.04));
#43835=CARTESIAN_POINT('',(0.146580359175541,-0.120889198458627,0.04));
#43836=CARTESIAN_POINT('',(0.144506032150084,-0.123361285143431,0.04));
#43837=CARTESIAN_POINT('Origin',(0.,0.,0.04));
#43838=CARTESIAN_POINT('',(0.140952177533892,-0.118272920182323,0.04));
#43839=CARTESIAN_POINT('',(0.165368846322791,-0.129623086932341,0.04));
#43840=CARTESIAN_POINT('',(0.140952177533892,-0.118272920182323,0.04));
#43841=CARTESIAN_POINT('Origin',(0.140952177533892,-0.118272920182323,0.04));
#43842=CARTESIAN_POINT('',(0.144506032150084,-0.123361285143431,0.185));
#43843=CARTESIAN_POINT('',(0.144506032150084,-0.123361285143431,0.0925));
#43844=CARTESIAN_POINT('',(0.140952177533892,-0.118272920182323,0.191));
#43845=CARTESIAN_POINT('',(0.140952177533892,-0.118272920182323,0.04));
#43846=CARTESIAN_POINT('Ctrl Pts',(0.144506032150084,-0.123361285143431,
0.185));
#43847=CARTESIAN_POINT('Ctrl Pts',(0.1427005979868,-0.120776286901188,0.188051499118426));
#43848=CARTESIAN_POINT('Ctrl Pts',(0.140952177533892,-0.118272920182323,
0.191));
#43849=CARTESIAN_POINT('Origin',(0.165368846322791,-0.129623086932341,0.04));
#43850=CARTESIAN_POINT('',(0.146580359175541,-0.120889198458627,0.185));
#43851=CARTESIAN_POINT('',(0.146580359175541,-0.120889198458627,0.0925));
#43852=CARTESIAN_POINT('Ctrl Pts',(0.140952177533892,-0.118272920182323,
0.191));
#43853=CARTESIAN_POINT('Ctrl Pts',(0.143721122512686,-0.1195600731311,0.188051499118447));
#43854=CARTESIAN_POINT('Ctrl Pts',(0.146580359175541,-0.120889198458627,
0.185));
#43855=CARTESIAN_POINT('Origin',(0.126629159108248,-0.150910755294439,0.04));
#43856=CARTESIAN_POINT('',(0.123361285143431,-0.144506032150084,0.04));
#43857=CARTESIAN_POINT('',(0.120889198458627,-0.146580359175541,0.04));
#43858=CARTESIAN_POINT('Origin',(0.,0.,0.04));
#43859=CARTESIAN_POINT('',(0.118272920182323,-0.140952177533892,0.04));
#43860=CARTESIAN_POINT('',(0.140347709136006,-0.15636981978718,0.04));
#43861=CARTESIAN_POINT('',(0.118272920182323,-0.140952177533892,0.04));
#43862=CARTESIAN_POINT('Origin',(0.118272920182323,-0.140952177533892,0.04));
#43863=CARTESIAN_POINT('',(0.120889198458627,-0.146580359175541,0.185));
#43864=CARTESIAN_POINT('',(0.120889198458627,-0.146580359175541,0.0925));
#43865=CARTESIAN_POINT('',(0.118272920182323,-0.140952177533892,0.191));
#43866=CARTESIAN_POINT('',(0.118272920182323,-0.140952177533892,0.04));
#43867=CARTESIAN_POINT('Ctrl Pts',(0.120889198458627,-0.146580359175541,
0.185));
#43868=CARTESIAN_POINT('Ctrl Pts',(0.119560073131107,-0.143721122512702,
0.18805149911843));
#43869=CARTESIAN_POINT('Ctrl Pts',(0.118272920182323,-0.140952177533892,
0.191));
#43870=CARTESIAN_POINT('Origin',(0.140347709136006,-0.15636981978718,0.04));
#43871=CARTESIAN_POINT('',(0.123361285143431,-0.144506032150084,0.185));
#43872=CARTESIAN_POINT('',(0.123361285143431,-0.144506032150084,0.0925));
#43873=CARTESIAN_POINT('Ctrl Pts',(0.118272920182323,-0.140952177533892,
0.191));
#43874=CARTESIAN_POINT('Ctrl Pts',(0.120776286901169,-0.142700597986787,
0.188051499118449));
#43875=CARTESIAN_POINT('Ctrl Pts',(0.123361285143431,-0.144506032150084,
0.185));
#43876=CARTESIAN_POINT('Origin',(0.0985,-0.170607004545534,0.04));
#43877=CARTESIAN_POINT('',(0.0963939408860592,-0.163732123178242,0.04));
#43878=CARTESIAN_POINT('',(0.0935992076448907,-0.165345663167344,0.04));
#43879=CARTESIAN_POINT('Origin',(0.,0.,0.04));
#43880=CARTESIAN_POINT('',(0.092,-0.159348674296337,0.04));
#43881=CARTESIAN_POINT('',(0.111062177826491,-0.178365334794732,0.04));
#43882=CARTESIAN_POINT('',(0.092,-0.159348674296337,0.04));
#43883=CARTESIAN_POINT('Origin',(0.092,-0.159348674296337,0.04));
#43884=CARTESIAN_POINT('',(0.0935992076448907,-0.165345663167344,0.185));
#43885=CARTESIAN_POINT('',(0.0935992076448907,-0.165345663167344,0.0925));
#43886=CARTESIAN_POINT('',(0.092,-0.159348674296337,0.191));
#43887=CARTESIAN_POINT('',(0.092,-0.159348674296337,0.04));
#43888=CARTESIAN_POINT('Ctrl Pts',(0.0935992076448907,-0.165345663167344,
0.185));
#43889=CARTESIAN_POINT('Ctrl Pts',(0.0927867759536364,-0.162299064543037,
0.188051499118462));
#43890=CARTESIAN_POINT('Ctrl Pts',(0.092,-0.159348674296337,0.191));
#43891=CARTESIAN_POINT('Origin',(0.111062177826491,-0.178365334794732,0.04));
#43892=CARTESIAN_POINT('',(0.0963939408860592,-0.163732123178242,0.185));
#43893=CARTESIAN_POINT('',(0.0963939408860592,-0.163732123178242,0.0925));
#43894=CARTESIAN_POINT('Ctrl Pts',(0.092,-0.159348674296337,0.191));
#43895=CARTESIAN_POINT('Ctrl Pts',(0.0941617249279249,-0.161505237382646,
0.18805149911843));
#43896=CARTESIAN_POINT('Ctrl Pts',(0.0963939408860592,-0.163732123178242,
0.185));
#43897=CARTESIAN_POINT('Origin',(0.0673779682351567,-0.185119446294824,
0.04));
#43898=CARTESIAN_POINT('',(0.0664977155125524,-0.17798329649608,0.04));
#43899=CARTESIAN_POINT('',(0.0634652522703484,-0.179087022852749,0.04));
#43900=CARTESIAN_POINT('Origin',(0.,0.,0.04));
#43901=CARTESIAN_POINT('',(0.062931706371923,-0.172903442224607,0.04));
#43902=CARTESIAN_POINT('',(0.0784020784438917,-0.194941309361761,0.04));
#43903=CARTESIAN_POINT('',(0.062931706371923,-0.172903442224607,0.04));
#43904=CARTESIAN_POINT('Origin',(0.062931706371923,-0.172903442224607,0.04));
#43905=CARTESIAN_POINT('',(0.0634652522703484,-0.179087022852749,0.185));
#43906=CARTESIAN_POINT('',(0.0634652522703484,-0.179087022852749,0.0925));
#43907=CARTESIAN_POINT('',(0.062931706371923,-0.172903442224607,0.191));
#43908=CARTESIAN_POINT('',(0.062931706371923,-0.172903442224607,0.04));
#43909=CARTESIAN_POINT('Ctrl Pts',(0.0634652522703485,-0.179087022852749,
0.185));
#43910=CARTESIAN_POINT('Ctrl Pts',(0.0631941995412026,-0.175945631624558,
0.188051499118454));
#43911=CARTESIAN_POINT('Ctrl Pts',(0.062931706371923,-0.172903442224607,
0.191));
#43912=CARTESIAN_POINT('Origin',(0.0784020784438917,-0.194941309361761,
0.04));
#43913=CARTESIAN_POINT('',(0.0664977155125524,-0.17798329649608,0.185));
#43914=CARTESIAN_POINT('',(0.0664977155125524,-0.17798329649608,0.0925));
#43915=CARTESIAN_POINT('Ctrl Pts',(0.062931706371923,-0.172903442224607,
0.191));
#43916=CARTESIAN_POINT('Ctrl Pts',(0.0646861065908383,-0.175402621866182,
0.18805149911847));
#43917=CARTESIAN_POINT('Ctrl Pts',(0.0664977155125524,-0.17798329649608,
0.185));
#43918=CARTESIAN_POINT('Origin',(0.0342086910003852,-0.194007127343405,
0.04));
#43919=CARTESIAN_POINT('',(0.0345809907026645,-0.186826537413779,0.04));
#43920=CARTESIAN_POINT('',(0.031402937320539,-0.18738691397118,0.04));
#43921=CARTESIAN_POINT('Origin',(0.,0.,0.04));
#43922=CARTESIAN_POINT('',(0.0319512646907151,-0.181204626554246,0.04));
#43923=CARTESIAN_POINT('',(0.0433597715811408,-0.205594090888895,0.04));
#43924=CARTESIAN_POINT('',(0.0319512646907151,-0.181204626554246,0.04));
#43925=CARTESIAN_POINT('Origin',(0.0319512646907151,-0.181204626554246,
0.04));
#43926=CARTESIAN_POINT('',(0.031402937320539,-0.18738691397118,0.185));
#43927=CARTESIAN_POINT('',(0.031402937320539,-0.18738691397118,0.0925));
#43928=CARTESIAN_POINT('',(0.0319512646907151,-0.181204626554246,0.191));
#43929=CARTESIAN_POINT('',(0.0319512646907151,-0.181204626554246,0.04));
#43930=CARTESIAN_POINT('Ctrl Pts',(0.031402937320539,-0.18738691397118,
0.185));
#43931=CARTESIAN_POINT('Ctrl Pts',(0.0316814993535159,-0.184246179721939,
0.18805149911846));
#43932=CARTESIAN_POINT('Ctrl Pts',(0.0319512646907151,-0.181204626554246,
0.191));
#43933=CARTESIAN_POINT('Origin',(0.0433597715811408,-0.205594090888895,
0.04));
#43934=CARTESIAN_POINT('',(0.0345809907026646,-0.186826537413779,0.185));
#43935=CARTESIAN_POINT('',(0.0345809907026646,-0.186826537413779,0.0925));
#43936=CARTESIAN_POINT('Ctrl Pts',(0.0319512646907151,-0.181204626554246,
0.191));
#43937=CARTESIAN_POINT('Ctrl Pts',(0.0332450336377804,-0.18397048644238,
0.188051499118441));
#43938=CARTESIAN_POINT('Ctrl Pts',(0.0345809907026645,-0.186826537413779,
0.185));
#43939=CARTESIAN_POINT('Origin',(-4.16333634234434E-17,-0.197,0.04));
#43940=CARTESIAN_POINT('',(0.00161353998910185,-0.18999314853095,0.04));
#43941=CARTESIAN_POINT('',(-0.00161353998910192,-0.18999314853095,0.04));
#43942=CARTESIAN_POINT('Origin',(0.,0.,0.04));
#43943=CARTESIAN_POINT('',(-3.46944695195361E-17,-0.184,0.04));
#43944=CARTESIAN_POINT('',(0.00699999999999997,-0.21,0.04));
#43945=CARTESIAN_POINT('',(-3.46944695195361E-17,-0.184,0.04));
#43946=CARTESIAN_POINT('Origin',(-3.46944695195361E-17,-0.184,0.04));
#43947=CARTESIAN_POINT('',(-0.00161353998910191,-0.18999314853095,0.185));
#43948=CARTESIAN_POINT('',(-0.00161353998910191,-0.18999314853095,0.0925));
#43949=CARTESIAN_POINT('',(-3.46944695195361E-17,-0.184,0.191));
#43950=CARTESIAN_POINT('',(-3.46944695195361E-17,-0.184,0.04));
#43951=CARTESIAN_POINT('Ctrl Pts',(-0.0016135399891019,-0.18999314853095,
0.185));
#43952=CARTESIAN_POINT('Ctrl Pts',(-0.000793827160417415,-0.18694850088155,
0.18805149911845));
#43953=CARTESIAN_POINT('Ctrl Pts',(-3.46944695195361E-17,-0.184,0.191));
#43954=CARTESIAN_POINT('Origin',(0.00699999999999997,-0.21,0.04));
#43955=CARTESIAN_POINT('',(0.00161353998910184,-0.18999314853095,0.185));
#43956=CARTESIAN_POINT('',(0.00161353998910184,-0.18999314853095,0.0925));
#43957=CARTESIAN_POINT('Ctrl Pts',(-3.46944695195361E-17,-0.184,0.191));
#43958=CARTESIAN_POINT('Ctrl Pts',(0.000793827160417323,-0.18694850088155,
0.18805149911845));
#43959=CARTESIAN_POINT('Ctrl Pts',(0.00161353998910184,-0.18999314853095,
0.185));
#43960=CARTESIAN_POINT('Origin',(-0.0342086910003853,-0.194007127343405,
0.04));
#43961=CARTESIAN_POINT('',(-0.0314029373205391,-0.18738691397118,0.04));
#43962=CARTESIAN_POINT('',(-0.0345809907026646,-0.186826537413779,0.04));
#43963=CARTESIAN_POINT('Origin',(0.,0.,0.04));
#43964=CARTESIAN_POINT('',(-0.0319512646907152,-0.181204626554246,0.04));
#43965=CARTESIAN_POINT('',(-0.0295724630389699,-0.208025165376232,0.04));
#43966=CARTESIAN_POINT('',(-0.0319512646907152,-0.181204626554246,0.04));
#43967=CARTESIAN_POINT('Origin',(-0.0319512646907152,-0.181204626554246,
0.04));
#43968=CARTESIAN_POINT('',(-0.0345809907026646,-0.186826537413779,0.185));
#43969=CARTESIAN_POINT('',(-0.0345809907026646,-0.186826537413779,0.0925));
#43970=CARTESIAN_POINT('',(-0.0319512646907152,-0.181204626554246,0.191));
#43971=CARTESIAN_POINT('',(-0.0319512646907152,-0.181204626554246,0.04));
#43972=CARTESIAN_POINT('Ctrl Pts',(-0.0345809907026646,-0.186826537413779,
0.185));
#43973=CARTESIAN_POINT('Ctrl Pts',(-0.033245033637776,-0.18397048644237,
0.188051499118451));
#43974=CARTESIAN_POINT('Ctrl Pts',(-0.0319512646907152,-0.181204626554246,
0.191));
#43975=CARTESIAN_POINT('Origin',(-0.0295724630389699,-0.208025165376232,
0.04));
#43976=CARTESIAN_POINT('',(-0.0314029373205391,-0.18738691397118,0.185));
#43977=CARTESIAN_POINT('',(-0.0314029373205391,-0.18738691397118,0.0925));
#43978=CARTESIAN_POINT('Ctrl Pts',(-0.0319512646907152,-0.181204626554246,
0.191));
#43979=CARTESIAN_POINT('Ctrl Pts',(-0.0316814993535157,-0.184246179721942,
0.188051499118457));
#43980=CARTESIAN_POINT('Ctrl Pts',(-0.0314029373205391,-0.18738691397118,
0.185));
#43981=CARTESIAN_POINT('Origin',(-0.0673779682351569,-0.185119446294824,
0.04));
#43982=CARTESIAN_POINT('',(-0.0634652522703487,-0.179087022852749,0.04));
#43983=CARTESIAN_POINT('',(-0.0664977155125527,-0.17798329649608,0.04));
#43984=CARTESIAN_POINT('Origin',(0.,0.,0.04));
#43985=CARTESIAN_POINT('',(-0.0629317063719232,-0.172903442224607,0.04));
#43986=CARTESIAN_POINT('',(-0.0652463817528892,-0.19972959136832,0.04));
#43987=CARTESIAN_POINT('',(-0.0629317063719232,-0.172903442224607,0.04));
#43988=CARTESIAN_POINT('Origin',(-0.0629317063719232,-0.172903442224607,
0.04));
#43989=CARTESIAN_POINT('',(-0.0664977155125527,-0.17798329649608,0.185));
#43990=CARTESIAN_POINT('',(-0.0664977155125527,-0.17798329649608,0.0925));
#43991=CARTESIAN_POINT('',(-0.0629317063719232,-0.172903442224607,0.191));
#43992=CARTESIAN_POINT('',(-0.0629317063719232,-0.172903442224607,0.04));
#43993=CARTESIAN_POINT('Ctrl Pts',(-0.0664977155125527,-0.17798329649608,
0.185));
#43994=CARTESIAN_POINT('Ctrl Pts',(-0.0646861065908368,-0.175402621866179,
0.188051499118473));
#43995=CARTESIAN_POINT('Ctrl Pts',(-0.0629317063719232,-0.172903442224607,
0.191));
#43996=CARTESIAN_POINT('Origin',(-0.0652463817528892,-0.19972959136832,
0.04));
#43997=CARTESIAN_POINT('',(-0.0634652522703487,-0.179087022852749,0.185));
#43998=CARTESIAN_POINT('',(-0.0634652522703487,-0.179087022852749,0.0925));
#43999=CARTESIAN_POINT('Ctrl Pts',(-0.0629317063719232,-0.172903442224607,
0.191));
#44000=CARTESIAN_POINT('Ctrl Pts',(-0.0631941995412029,-0.175945631624558,
0.188051499118454));
#44001=CARTESIAN_POINT('Ctrl Pts',(-0.0634652522703487,-0.179087022852749,
0.185));
#44002=CARTESIAN_POINT('Origin',(-0.0985000000000001,-0.170607004545534,
0.04));
#44003=CARTESIAN_POINT('',(-0.0935992076448907,-0.165345663167344,0.04));
#44004=CARTESIAN_POINT('',(-0.0963939408860593,-0.163732123178242,0.04));
#44005=CARTESIAN_POINT('Origin',(0.,0.,0.04));
#44006=CARTESIAN_POINT('',(-0.0920000000000001,-0.159348674296337,0.04));
#44007=CARTESIAN_POINT('',(-0.098937822173509,-0.185365334794732,0.04));
#44008=CARTESIAN_POINT('',(-0.0920000000000001,-0.159348674296337,0.04));
#44009=CARTESIAN_POINT('Origin',(-0.0920000000000001,-0.159348674296337,
0.04));
#44010=CARTESIAN_POINT('',(-0.0963939408860593,-0.163732123178242,0.185));
#44011=CARTESIAN_POINT('',(-0.0963939408860593,-0.163732123178242,0.0925));
#44012=CARTESIAN_POINT('',(-0.0920000000000001,-0.159348674296337,0.191));
#44013=CARTESIAN_POINT('',(-0.0920000000000001,-0.159348674296337,0.04));
#44014=CARTESIAN_POINT('Ctrl Pts',(-0.0963939408860593,-0.163732123178242,
0.185));
#44015=CARTESIAN_POINT('Ctrl Pts',(-0.0941617249279212,-0.161505237382642,
0.188051499118436));
#44016=CARTESIAN_POINT('Ctrl Pts',(-0.0920000000000001,-0.159348674296337,
0.191));
#44017=CARTESIAN_POINT('Origin',(-0.098937822173509,-0.185365334794732,
0.04));
#44018=CARTESIAN_POINT('',(-0.0935992076448907,-0.165345663167344,0.185));
#44019=CARTESIAN_POINT('',(-0.0935992076448907,-0.165345663167344,0.0925));
#44020=CARTESIAN_POINT('Ctrl Pts',(-0.0920000000000001,-0.159348674296337,
0.191));
#44021=CARTESIAN_POINT('Ctrl Pts',(-0.0927867759536363,-0.162299064543036,
0.188051499118462));
#44022=CARTESIAN_POINT('Ctrl Pts',(-0.0935992076448907,-0.165345663167344,
0.185));
#44023=CARTESIAN_POINT('Origin',(-0.126629159108248,-0.150910755294439,
0.04));
#44024=CARTESIAN_POINT('',(-0.120889198458627,-0.146580359175541,0.04));
#44025=CARTESIAN_POINT('',(-0.123361285143431,-0.144506032150084,0.04));
#44026=CARTESIAN_POINT('Origin',(0.,0.,0.04));
#44027=CARTESIAN_POINT('',(-0.118272920182323,-0.140952177533892,0.04));
#44028=CARTESIAN_POINT('',(-0.12962308693234,-0.165368846322791,0.04));
#44029=CARTESIAN_POINT('',(-0.118272920182323,-0.140952177533892,0.04));
#44030=CARTESIAN_POINT('Origin',(-0.118272920182323,-0.140952177533892,
0.04));
#44031=CARTESIAN_POINT('',(-0.123361285143431,-0.144506032150084,0.185));
#44032=CARTESIAN_POINT('',(-0.123361285143431,-0.144506032150084,0.0925));
#44033=CARTESIAN_POINT('',(-0.118272920182323,-0.140952177533892,0.191));
#44034=CARTESIAN_POINT('',(-0.118272920182323,-0.140952177533892,0.04));
#44035=CARTESIAN_POINT('Ctrl Pts',(-0.123361285143431,-0.144506032150084,
0.185));
#44036=CARTESIAN_POINT('Ctrl Pts',(-0.120776286901195,-0.142700597986805,
0.188051499118418));
#44037=CARTESIAN_POINT('Ctrl Pts',(-0.118272920182323,-0.140952177533892,
0.191));
#44038=CARTESIAN_POINT('Origin',(-0.12962308693234,-0.165368846322791,0.04));
#44039=CARTESIAN_POINT('',(-0.120889198458627,-0.146580359175541,0.185));
#44040=CARTESIAN_POINT('',(-0.120889198458627,-0.146580359175541,0.0925));
#44041=CARTESIAN_POINT('Ctrl Pts',(-0.118272920182323,-0.140952177533892,
0.191));
#44042=CARTESIAN_POINT('Ctrl Pts',(-0.119560073131103,-0.143721122512692,
0.188051499118441));
#44043=CARTESIAN_POINT('Ctrl Pts',(-0.120889198458627,-0.146580359175541,
0.185));
#44044=CARTESIAN_POINT('Origin',(-0.150910755294439,-0.126629159108248,
0.04));
#44045=CARTESIAN_POINT('',(-0.144506032150084,-0.123361285143431,0.04));
#44046=CARTESIAN_POINT('',(-0.146580359175541,-0.120889198458627,0.04));
#44047=CARTESIAN_POINT('Origin',(0.,0.,0.04));
#44048=CARTESIAN_POINT('',(-0.140952177533892,-0.118272920182323,0.04));
#44049=CARTESIAN_POINT('',(-0.15636981978718,-0.140347709136006,0.04));
#44050=CARTESIAN_POINT('',(-0.140952177533892,-0.118272920182323,0.04));
#44051=CARTESIAN_POINT('Origin',(-0.140952177533892,-0.118272920182323,
0.04));
#44052=CARTESIAN_POINT('',(-0.146580359175541,-0.120889198458627,0.185));
#44053=CARTESIAN_POINT('',(-0.146580359175541,-0.120889198458627,0.0925));
#44054=CARTESIAN_POINT('',(-0.140952177533892,-0.118272920182323,0.191));
#44055=CARTESIAN_POINT('',(-0.140952177533892,-0.118272920182323,0.04));
#44056=CARTESIAN_POINT('Ctrl Pts',(-0.146580359175541,-0.120889198458627,
0.185));
#44057=CARTESIAN_POINT('Ctrl Pts',(-0.14372112251267,-0.119560073131093,
0.188051499118464));
#44058=CARTESIAN_POINT('Ctrl Pts',(-0.140952177533892,-0.118272920182323,
0.191));
#44059=CARTESIAN_POINT('Origin',(-0.15636981978718,-0.140347709136006,0.04));
#44060=CARTESIAN_POINT('',(-0.144506032150084,-0.123361285143431,0.185));
#44061=CARTESIAN_POINT('',(-0.144506032150084,-0.123361285143431,0.0925));
#44062=CARTESIAN_POINT('Ctrl Pts',(-0.140952177533892,-0.118272920182323,
0.191));
#44063=CARTESIAN_POINT('Ctrl Pts',(-0.142700597986788,-0.120776286901171,
0.188051499118446));
#44064=CARTESIAN_POINT('Ctrl Pts',(-0.144506032150084,-0.123361285143431,
0.185));
#44065=CARTESIAN_POINT('Origin',(-0.170607004545534,-0.0985,0.04));
#44066=CARTESIAN_POINT('',(-0.163732123178242,-0.0963939408860592,0.04));
#44067=CARTESIAN_POINT('',(-0.165345663167344,-0.0935992076448906,0.04));
#44068=CARTESIAN_POINT('Origin',(0.,0.,0.04));
#44069=CARTESIAN_POINT('',(-0.159348674296337,-0.092,0.04));
#44070=CARTESIAN_POINT('',(-0.178365334794732,-0.111062177826491,0.04));
#44071=CARTESIAN_POINT('',(-0.159348674296337,-0.092,0.04));
#44072=CARTESIAN_POINT('Origin',(-0.159348674296337,-0.092,0.04));
#44073=CARTESIAN_POINT('',(-0.165345663167344,-0.0935992076448906,0.185));
#44074=CARTESIAN_POINT('',(-0.165345663167344,-0.0935992076448906,0.0925));
#44075=CARTESIAN_POINT('',(-0.159348674296337,-0.0919999999999999,0.191));
#44076=CARTESIAN_POINT('',(-0.159348674296337,-0.092,0.04));
#44077=CARTESIAN_POINT('Ctrl Pts',(-0.165345663167344,-0.0935992076448906,
0.185));
#44078=CARTESIAN_POINT('Ctrl Pts',(-0.16229906454304,-0.0927867759536372,
0.188051499118458));
#44079=CARTESIAN_POINT('Ctrl Pts',(-0.159348674296337,-0.0919999999999999,
0.191));
#44080=CARTESIAN_POINT('Origin',(-0.178365334794732,-0.111062177826491,
0.04));
#44081=CARTESIAN_POINT('',(-0.163732123178242,-0.0963939408860592,0.185));
#44082=CARTESIAN_POINT('',(-0.163732123178242,-0.0963939408860592,0.0925));
#44083=CARTESIAN_POINT('Ctrl Pts',(-0.159348674296337,-0.0919999999999999,
0.191));
#44084=CARTESIAN_POINT('Ctrl Pts',(-0.161505237382618,-0.0941617249278968,
0.188051499118469));
#44085=CARTESIAN_POINT('Ctrl Pts',(-0.163732123178242,-0.0963939408860592,
0.185));
#44086=CARTESIAN_POINT('Origin',(-0.185119446294824,-0.0673779682351567,
0.04));
#44087=CARTESIAN_POINT('',(-0.17798329649608,-0.0664977155125525,0.04));
#44088=CARTESIAN_POINT('',(-0.179087022852749,-0.0634652522703485,0.04));
#44089=CARTESIAN_POINT('Origin',(0.,0.,0.04));
#44090=CARTESIAN_POINT('',(-0.172903442224607,-0.062931706371923,0.04));
#44091=CARTESIAN_POINT('',(-0.194941309361761,-0.0784020784438918,0.04));
#44092=CARTESIAN_POINT('',(-0.172903442224607,-0.062931706371923,0.04));
#44093=CARTESIAN_POINT('Origin',(-0.172903442224607,-0.062931706371923,
0.04));
#44094=CARTESIAN_POINT('',(-0.179087022852749,-0.0634652522703485,0.185));
#44095=CARTESIAN_POINT('',(-0.179087022852749,-0.0634652522703485,0.0925));
#44096=CARTESIAN_POINT('',(-0.172903442224607,-0.062931706371923,0.191));
#44097=CARTESIAN_POINT('',(-0.172903442224607,-0.062931706371923,0.04));
#44098=CARTESIAN_POINT('Ctrl Pts',(-0.179087022852749,-0.0634652522703485,
0.185));
#44099=CARTESIAN_POINT('Ctrl Pts',(-0.175945631624537,-0.0631941995412009,
0.188051499118474));
#44100=CARTESIAN_POINT('Ctrl Pts',(-0.172903442224607,-0.062931706371923,
0.191));
#44101=CARTESIAN_POINT('Origin',(-0.194941309361761,-0.0784020784438918,
0.04));
#44102=CARTESIAN_POINT('',(-0.17798329649608,-0.0664977155125525,0.185));
#44103=CARTESIAN_POINT('',(-0.17798329649608,-0.0664977155125525,0.0925));
#44104=CARTESIAN_POINT('Ctrl Pts',(-0.172903442224607,-0.062931706371923,
0.191));
#44105=CARTESIAN_POINT('Ctrl Pts',(-0.175402621866193,-0.0646861065908464,
0.188051499118456));
#44106=CARTESIAN_POINT('Ctrl Pts',(-0.17798329649608,-0.0664977155125525,
0.185));
#44107=CARTESIAN_POINT('Origin',(-0.194007127343405,-0.0342086910003852,
0.04));
#44108=CARTESIAN_POINT('',(-0.186826537413779,-0.0345809907026646,0.04));
#44109=CARTESIAN_POINT('',(-0.18738691397118,-0.031402937320539,0.04));
#44110=CARTESIAN_POINT('Origin',(0.,0.,0.04));
#44111=CARTESIAN_POINT('',(-0.181204626554246,-0.0319512646907151,0.04));
#44112=CARTESIAN_POINT('',(-0.205594090888895,-0.0433597715811408,0.04));
#44113=CARTESIAN_POINT('',(-0.181204626554246,-0.0319512646907151,0.04));
#44114=CARTESIAN_POINT('Origin',(-0.181204626554246,-0.0319512646907151,
0.04));
#44115=CARTESIAN_POINT('',(-0.18738691397118,-0.031402937320539,0.185));
#44116=CARTESIAN_POINT('',(-0.18738691397118,-0.031402937320539,0.0925));
#44117=CARTESIAN_POINT('',(-0.181204626554246,-0.0319512646907151,0.191));
#44118=CARTESIAN_POINT('',(-0.181204626554246,-0.0319512646907151,0.04));
#44119=CARTESIAN_POINT('Ctrl Pts',(-0.18738691397118,-0.031402937320539,
0.185));
#44120=CARTESIAN_POINT('Ctrl Pts',(-0.184246179721915,-0.031681499353518,
0.188051499118483));
#44121=CARTESIAN_POINT('Ctrl Pts',(-0.181204626554246,-0.0319512646907151,
0.191));
#44122=CARTESIAN_POINT('Origin',(-0.205594090888895,-0.0433597715811408,
0.04));
#44123=CARTESIAN_POINT('',(-0.186826537413779,-0.0345809907026646,0.185));
#44124=CARTESIAN_POINT('',(-0.186826537413779,-0.0345809907026646,0.0925));
#44125=CARTESIAN_POINT('Ctrl Pts',(-0.181204626554246,-0.0319512646907151,
0.191));
#44126=CARTESIAN_POINT('Ctrl Pts',(-0.183970486442384,-0.0332450336377824,
0.188051499118436));
#44127=CARTESIAN_POINT('Ctrl Pts',(-0.186826537413779,-0.0345809907026646,
0.185));
#44128=CARTESIAN_POINT('Origin',(-0.197,2.08166817117217E-17,0.04));
#44129=CARTESIAN_POINT('',(-0.18999314853095,-0.00161353998910186,0.04));
#44130=CARTESIAN_POINT('',(-0.19,-2.32682891837997E-17,0.04));
#44131=CARTESIAN_POINT('Origin',(0.,0.,0.04));
#44132=CARTESIAN_POINT('',(-0.184,2.08166817117217E-17,0.04));
#44133=CARTESIAN_POINT('',(-0.21,-0.00699999999999998,0.04));
#44134=CARTESIAN_POINT('',(-0.18999314853095,0.0016135399891019,0.04));
#44135=CARTESIAN_POINT('',(-0.184,2.08166817117217E-17,0.04));
#44136=CARTESIAN_POINT('Origin',(0.,0.,0.04));
#44137=CARTESIAN_POINT('Origin',(-0.184,2.08166817117217E-17,0.04));
#44138=CARTESIAN_POINT('',(-0.18999314853095,0.00161353998910189,0.185));
#44139=CARTESIAN_POINT('',(-0.18999314853095,0.00161353998910189,0.0925));
#44140=CARTESIAN_POINT('',(-0.184,2.08166817117217E-17,0.191));
#44141=CARTESIAN_POINT('',(-0.184,2.08166817117217E-17,0.04));
#44142=CARTESIAN_POINT('Ctrl Pts',(-0.18999314853095,0.00161353998910189,
0.185));
#44143=CARTESIAN_POINT('Ctrl Pts',(-0.186948500881544,0.000793827160415821,
0.188051499118456));
#44144=CARTESIAN_POINT('Ctrl Pts',(-0.184,2.08166817117217E-17,0.191));
#44145=CARTESIAN_POINT('Origin',(-0.21,-0.00699999999999998,0.04));
#44146=CARTESIAN_POINT('',(-0.18999314853095,-0.00161353998910186,0.185));
#44147=CARTESIAN_POINT('',(-0.18999314853095,-0.00161353998910186,0.0925));
#44148=CARTESIAN_POINT('Ctrl Pts',(-0.184,2.08166817117217E-17,0.191));
#44149=CARTESIAN_POINT('Ctrl Pts',(-0.186948500881545,-0.000793827160416021,
0.188051499118455));
#44150=CARTESIAN_POINT('Ctrl Pts',(-0.18999314853095,-0.00161353998910185,
0.185));
#44151=CARTESIAN_POINT('Origin',(-0.194007127343405,0.0342086910003854,
0.04));
#44152=CARTESIAN_POINT('',(-0.18738691397118,0.0314029373205392,0.04));
#44153=CARTESIAN_POINT('',(-0.186826537413779,0.0345809907026647,0.04));
#44154=CARTESIAN_POINT('Origin',(0.,0.,0.04));
#44155=CARTESIAN_POINT('',(-0.181204626554246,0.0319512646907152,0.04));
#44156=CARTESIAN_POINT('',(-0.208025165376232,0.02957246303897,0.04));
#44157=CARTESIAN_POINT('',(-0.181204626554246,0.0319512646907152,0.04));
#44158=CARTESIAN_POINT('Origin',(-0.181204626554246,0.0319512646907152,
0.04));
#44159=CARTESIAN_POINT('',(-0.186826537413779,0.0345809907026647,0.185));
#44160=CARTESIAN_POINT('',(-0.186826537413779,0.0345809907026647,0.0925));
#44161=CARTESIAN_POINT('',(-0.181204626554246,0.0319512646907153,0.191));
#44162=CARTESIAN_POINT('',(-0.181204626554246,0.0319512646907152,0.04));
#44163=CARTESIAN_POINT('Ctrl Pts',(-0.186826537413779,0.0345809907026647,
0.185));
#44164=CARTESIAN_POINT('Ctrl Pts',(-0.183970486442384,0.0332450336377824,
0.188051499118436));
#44165=CARTESIAN_POINT('Ctrl Pts',(-0.181204626554246,0.0319512646907153,
0.191));
#44166=CARTESIAN_POINT('Origin',(-0.208025165376232,0.02957246303897,0.04));
#44167=CARTESIAN_POINT('',(-0.18738691397118,0.0314029373205392,0.185));
#44168=CARTESIAN_POINT('',(-0.18738691397118,0.0314029373205392,0.0925));
#44169=CARTESIAN_POINT('Ctrl Pts',(-0.181204626554246,0.0319512646907153,
0.191));
#44170=CARTESIAN_POINT('Ctrl Pts',(-0.184246179721934,0.0316814993535164,
0.188051499118464));
#44171=CARTESIAN_POINT('Ctrl Pts',(-0.18738691397118,0.0314029373205392,
0.185));
#44172=CARTESIAN_POINT('Origin',(-0.185119446294824,0.0673779682351568,
0.04));
#44173=CARTESIAN_POINT('',(-0.179087022852749,0.0634652522703486,0.04));
#44174=CARTESIAN_POINT('',(-0.17798329649608,0.0664977155125526,0.04));
#44175=CARTESIAN_POINT('Origin',(0.,0.,0.04));
#44176=CARTESIAN_POINT('',(-0.172903442224607,0.0629317063719231,0.04));
#44177=CARTESIAN_POINT('',(-0.199729591368321,0.0652463817528891,0.04));
#44178=CARTESIAN_POINT('',(-0.172903442224607,0.0629317063719231,0.04));
#44179=CARTESIAN_POINT('Origin',(-0.172903442224607,0.0629317063719231,
0.04));
#44180=CARTESIAN_POINT('',(-0.17798329649608,0.0664977155125526,0.185));
#44181=CARTESIAN_POINT('',(-0.17798329649608,0.0664977155125526,0.0925));
#44182=CARTESIAN_POINT('',(-0.172903442224607,0.0629317063719231,0.191));
#44183=CARTESIAN_POINT('',(-0.172903442224607,0.0629317063719231,0.04));
#44184=CARTESIAN_POINT('Ctrl Pts',(-0.17798329649608,0.0664977155125526,
0.185));
#44185=CARTESIAN_POINT('Ctrl Pts',(-0.175402621866187,0.0646861065908417,
0.188051499118464));
#44186=CARTESIAN_POINT('Ctrl Pts',(-0.172903442224607,0.0629317063719231,
0.191));
#44187=CARTESIAN_POINT('Origin',(-0.199729591368321,0.0652463817528891,
0.04));
#44188=CARTESIAN_POINT('',(-0.179087022852749,0.0634652522703485,0.185));
#44189=CARTESIAN_POINT('',(-0.179087022852749,0.0634652522703485,0.0925));
#44190=CARTESIAN_POINT('Ctrl Pts',(-0.172903442224607,0.0629317063719231,
0.191));
#44191=CARTESIAN_POINT('Ctrl Pts',(-0.175945631624522,0.0631941995411996,
0.188051499118489));
#44192=CARTESIAN_POINT('Ctrl Pts',(-0.179087022852749,0.0634652522703486,
0.185));
#44193=CARTESIAN_POINT('Origin',(-0.170607004545534,0.0985,0.04));
#44194=CARTESIAN_POINT('',(-0.165345663167344,0.0935992076448906,0.04));
#44195=CARTESIAN_POINT('',(-0.163732123178242,0.0963939408860592,0.04));
#44196=CARTESIAN_POINT('Origin',(0.,0.,0.04));
#44197=CARTESIAN_POINT('',(-0.159348674296337,0.092,0.04));
#44198=CARTESIAN_POINT('',(-0.185365334794732,0.098937822173509,0.04));
#44199=CARTESIAN_POINT('',(-0.159348674296337,0.092,0.04));
#44200=CARTESIAN_POINT('Origin',(-0.159348674296337,0.092,0.04));
#44201=CARTESIAN_POINT('',(-0.163732123178242,0.0963939408860592,0.185));
#44202=CARTESIAN_POINT('',(-0.163732123178242,0.0963939408860592,0.0925));
#44203=CARTESIAN_POINT('',(-0.159348674296337,0.092,0.191));
#44204=CARTESIAN_POINT('',(-0.159348674296337,0.092,0.04));
#44205=CARTESIAN_POINT('Ctrl Pts',(-0.163732123178242,0.0963939408860592,
0.185));
#44206=CARTESIAN_POINT('Ctrl Pts',(-0.161505237382624,0.0941617249279029,
0.18805149911846));
#44207=CARTESIAN_POINT('Ctrl Pts',(-0.159348674296337,0.092,0.191));
#44208=CARTESIAN_POINT('Origin',(-0.185365334794732,0.098937822173509,0.04));
#44209=CARTESIAN_POINT('',(-0.165345663167344,0.0935992076448906,0.185));
#44210=CARTESIAN_POINT('',(-0.165345663167344,0.0935992076448906,0.0925));
#44211=CARTESIAN_POINT('Ctrl Pts',(-0.159348674296337,0.092,0.191));
#44212=CARTESIAN_POINT('Ctrl Pts',(-0.162299064543065,0.0927867759536439,
0.188051499118434));
#44213=CARTESIAN_POINT('Ctrl Pts',(-0.165345663167344,0.0935992076448907,
0.185));
#44214=CARTESIAN_POINT('Origin',(-0.150910755294439,0.126629159108248,0.04));
#44215=CARTESIAN_POINT('',(-0.146580359175541,0.120889198458627,0.04));
#44216=CARTESIAN_POINT('',(-0.144506032150084,0.123361285143431,0.04));
#44217=CARTESIAN_POINT('Origin',(0.,0.,0.04));
#44218=CARTESIAN_POINT('',(-0.140952177533892,0.118272920182323,0.04));
#44219=CARTESIAN_POINT('',(-0.165368846322791,0.12962308693234,0.04));
#44220=CARTESIAN_POINT('',(-0.140952177533892,0.118272920182323,0.04));
#44221=CARTESIAN_POINT('Origin',(-0.140952177533892,0.118272920182323,0.04));
#44222=CARTESIAN_POINT('',(-0.144506032150084,0.123361285143431,0.185));
#44223=CARTESIAN_POINT('',(-0.144506032150084,0.123361285143431,0.0925));
#44224=CARTESIAN_POINT('',(-0.140952177533892,0.118272920182323,0.191));
#44225=CARTESIAN_POINT('',(-0.140952177533892,0.118272920182323,0.04));
#44226=CARTESIAN_POINT('Ctrl Pts',(-0.144506032150084,0.123361285143431,
0.185));
#44227=CARTESIAN_POINT('Ctrl Pts',(-0.142700597986805,0.120776286901195,
0.188051499118418));
#44228=CARTESIAN_POINT('Ctrl Pts',(-0.140952177533892,0.118272920182323,
0.191));
#44229=CARTESIAN_POINT('Origin',(-0.165368846322791,0.12962308693234,0.04));
#44230=CARTESIAN_POINT('',(-0.146580359175541,0.120889198458627,0.185));
#44231=CARTESIAN_POINT('',(-0.146580359175541,0.120889198458627,0.0925));
#44232=CARTESIAN_POINT('Ctrl Pts',(-0.140952177533892,0.118272920182323,
0.191));
#44233=CARTESIAN_POINT('Ctrl Pts',(-0.143721122512692,0.119560073131103,
0.188051499118441));
#44234=CARTESIAN_POINT('Ctrl Pts',(-0.146580359175541,0.120889198458627,
0.185));
#44235=CARTESIAN_POINT('Origin',(-0.126629159108248,0.150910755294439,0.04));
#44236=CARTESIAN_POINT('',(-0.123361285143431,0.144506032150084,0.04));
#44237=CARTESIAN_POINT('',(-0.120889198458627,0.146580359175541,0.04));
#44238=CARTESIAN_POINT('Origin',(0.,0.,0.04));
#44239=CARTESIAN_POINT('',(-0.118272920182323,0.140952177533892,0.04));
#44240=CARTESIAN_POINT('',(-0.140347709136006,0.15636981978718,0.04));
#44241=CARTESIAN_POINT('',(-0.118272920182323,0.140952177533892,0.04));
#44242=CARTESIAN_POINT('Origin',(-0.118272920182323,0.140952177533892,0.04));
#44243=CARTESIAN_POINT('',(-0.120889198458627,0.146580359175541,0.185));
#44244=CARTESIAN_POINT('',(-0.120889198458627,0.146580359175541,0.0925));
#44245=CARTESIAN_POINT('',(-0.118272920182323,0.140952177533892,0.191));
#44246=CARTESIAN_POINT('',(-0.118272920182323,0.140952177533892,0.04));
#44247=CARTESIAN_POINT('Ctrl Pts',(-0.120889198458627,0.146580359175541,
0.185));
#44248=CARTESIAN_POINT('Ctrl Pts',(-0.1195600731311,0.143721122512687,0.188051499118446));
#44249=CARTESIAN_POINT('Ctrl Pts',(-0.118272920182323,0.140952177533892,
0.191));
#44250=CARTESIAN_POINT('Origin',(-0.140347709136006,0.15636981978718,0.04));
#44251=CARTESIAN_POINT('',(-0.123361285143431,0.144506032150084,0.185));
#44252=CARTESIAN_POINT('',(-0.123361285143431,0.144506032150084,0.0925));
#44253=CARTESIAN_POINT('Ctrl Pts',(-0.118272920182323,0.140952177533892,
0.191));
#44254=CARTESIAN_POINT('Ctrl Pts',(-0.120776286901187,0.142700597986799,
0.188051499118427));
#44255=CARTESIAN_POINT('Ctrl Pts',(-0.123361285143431,0.144506032150084,
0.185));
#44256=CARTESIAN_POINT('Origin',(-0.0985,0.170607004545534,0.04));
#44257=CARTESIAN_POINT('',(-0.0963939408860591,0.163732123178242,0.04));
#44258=CARTESIAN_POINT('',(-0.0935992076448906,0.165345663167344,0.04));
#44259=CARTESIAN_POINT('Origin',(0.,0.,0.04));
#44260=CARTESIAN_POINT('',(-0.092,0.159348674296337,0.04));
#44261=CARTESIAN_POINT('',(-0.111062177826491,0.178365334794732,0.04));
#44262=CARTESIAN_POINT('',(-0.092,0.159348674296337,0.04));
#44263=CARTESIAN_POINT('Origin',(-0.092,0.159348674296337,0.04));
#44264=CARTESIAN_POINT('',(-0.0935992076448906,0.165345663167344,0.185));
#44265=CARTESIAN_POINT('',(-0.0935992076448906,0.165345663167344,0.0925));
#44266=CARTESIAN_POINT('',(-0.092,0.159348674296337,0.191));
#44267=CARTESIAN_POINT('',(-0.092,0.159348674296337,0.04));
#44268=CARTESIAN_POINT('Ctrl Pts',(-0.0935992076448906,0.165345663167344,
0.185));
#44269=CARTESIAN_POINT('Ctrl Pts',(-0.0927867759536353,0.162299064543033,
0.188051499118466));
#44270=CARTESIAN_POINT('Ctrl Pts',(-0.092,0.159348674296337,0.191));
#44271=CARTESIAN_POINT('Origin',(-0.111062177826491,0.178365334794732,0.04));
#44272=CARTESIAN_POINT('',(-0.0963939408860592,0.163732123178242,0.185));
#44273=CARTESIAN_POINT('',(-0.0963939408860592,0.163732123178242,0.0925));
#44274=CARTESIAN_POINT('Ctrl Pts',(-0.092,0.159348674296337,0.191));
#44275=CARTESIAN_POINT('Ctrl Pts',(-0.0941617249279073,0.161505237382628,
0.188051499118454));
#44276=CARTESIAN_POINT('Ctrl Pts',(-0.0963939408860592,0.163732123178242,
0.185));
#44277=CARTESIAN_POINT('Origin',(-0.0673779682351567,0.185119446294824,
0.04));
#44278=CARTESIAN_POINT('',(-0.0664977155125525,0.17798329649608,0.04));
#44279=CARTESIAN_POINT('',(-0.0634652522703485,0.179087022852749,0.04));
#44280=CARTESIAN_POINT('Origin',(0.,0.,0.04));
#44281=CARTESIAN_POINT('',(-0.062931706371923,0.172903442224607,0.04));
#44282=CARTESIAN_POINT('',(-0.0784020784438918,0.194941309361761,0.04));
#44283=CARTESIAN_POINT('',(-0.062931706371923,0.172903442224607,0.04));
#44284=CARTESIAN_POINT('Origin',(-0.062931706371923,0.172903442224607,0.04));
#44285=CARTESIAN_POINT('',(-0.0634652522703485,0.179087022852749,0.185));
#44286=CARTESIAN_POINT('',(-0.0634652522703485,0.179087022852749,0.0925));
#44287=CARTESIAN_POINT('',(-0.062931706371923,0.172903442224607,0.191));
#44288=CARTESIAN_POINT('',(-0.062931706371923,0.172903442224607,0.04));
#44289=CARTESIAN_POINT('Ctrl Pts',(-0.0634652522703485,0.179087022852749,
0.185));
#44290=CARTESIAN_POINT('Ctrl Pts',(-0.0631941995412009,0.175945631624537,
0.188051499118474));
#44291=CARTESIAN_POINT('Ctrl Pts',(-0.062931706371923,0.172903442224607,
0.191));
#44292=CARTESIAN_POINT('Origin',(-0.0784020784438918,0.194941309361761,
0.04));
#44293=CARTESIAN_POINT('',(-0.0664977155125525,0.17798329649608,0.185));
#44294=CARTESIAN_POINT('',(-0.0664977155125525,0.17798329649608,0.0925));
#44295=CARTESIAN_POINT('Ctrl Pts',(-0.062931706371923,0.172903442224607,
0.191));
#44296=CARTESIAN_POINT('Ctrl Pts',(-0.0646861065908464,0.175402621866193,
0.188051499118456));
#44297=CARTESIAN_POINT('Ctrl Pts',(-0.0664977155125525,0.17798329649608,
0.185));
#44298=CARTESIAN_POINT('Origin',(-0.0342086910003853,0.194007127343405,
0.04));
#44299=CARTESIAN_POINT('',(-0.0345809907026646,0.186826537413779,0.04));
#44300=CARTESIAN_POINT('',(-0.0314029373205391,0.18738691397118,0.04));
#44301=CARTESIAN_POINT('Origin',(0.,0.,0.04));
#44302=CARTESIAN_POINT('',(-0.0319512646907152,0.181204626554246,0.04));
#44303=CARTESIAN_POINT('',(-0.0433597715811408,0.205594090888895,0.04));
#44304=CARTESIAN_POINT('',(-0.0319512646907152,0.181204626554246,0.04));
#44305=CARTESIAN_POINT('Origin',(-0.0319512646907152,0.181204626554246,
0.04));
#44306=CARTESIAN_POINT('',(-0.0314029373205391,0.18738691397118,0.185));
#44307=CARTESIAN_POINT('',(-0.0314029373205391,0.18738691397118,0.0925));
#44308=CARTESIAN_POINT('',(-0.0319512646907152,0.181204626554246,0.191));
#44309=CARTESIAN_POINT('',(-0.0319512646907152,0.181204626554246,0.04));
#44310=CARTESIAN_POINT('Ctrl Pts',(-0.0314029373205391,0.18738691397118,
0.185));
#44311=CARTESIAN_POINT('Ctrl Pts',(-0.031681499353516,0.184246179721939,
0.18805149911846));
#44312=CARTESIAN_POINT('Ctrl Pts',(-0.0319512646907152,0.181204626554246,
0.191));
#44313=CARTESIAN_POINT('Origin',(-0.0433597715811408,0.205594090888895,
0.04));
#44314=CARTESIAN_POINT('',(-0.0345809907026646,0.186826537413779,0.185));
#44315=CARTESIAN_POINT('',(-0.0345809907026646,0.186826537413779,0.0925));
#44316=CARTESIAN_POINT('Ctrl Pts',(-0.0319512646907152,0.181204626554246,
0.191));
#44317=CARTESIAN_POINT('Ctrl Pts',(-0.033245033637777,0.183970486442373,
0.188051499118448));
#44318=CARTESIAN_POINT('Ctrl Pts',(-0.0345809907026646,0.186826537413779,
0.185));
#44319=CARTESIAN_POINT('Origin',(1.38777878078145E-17,0.197,0.04));
#44320=CARTESIAN_POINT('',(-0.00161353998910187,0.18999314853095,0.04));
#44321=CARTESIAN_POINT('',(0.00161353998910189,0.18999314853095,0.04));
#44322=CARTESIAN_POINT('Origin',(0.,0.,0.04));
#44323=CARTESIAN_POINT('',(6.93889390390723E-18,0.184,0.04));
#44324=CARTESIAN_POINT('',(-0.00699999999999999,0.21,0.04));
#44325=CARTESIAN_POINT('',(6.93889390390723E-18,0.184,0.04));
#44326=CARTESIAN_POINT('Origin',(6.93889390390723E-18,0.184,0.04));
#44327=CARTESIAN_POINT('',(0.00161353998910188,0.18999314853095,0.185));
#44328=CARTESIAN_POINT('',(0.00161353998910188,0.18999314853095,0.0925));
#44329=CARTESIAN_POINT('',(6.93889390390723E-18,0.184,0.191));
#44330=CARTESIAN_POINT('',(6.93889390390723E-18,0.184,0.04));
#44331=CARTESIAN_POINT('Ctrl Pts',(0.00161353998910188,0.18999314853095,
0.185));
#44332=CARTESIAN_POINT('Ctrl Pts',(0.000793827160417808,0.186948500881552,
0.188051499118448));
#44333=CARTESIAN_POINT('Ctrl Pts',(6.93889390390723E-18,0.184,0.191));
#44334=CARTESIAN_POINT('Origin',(-0.00699999999999999,0.21,0.04));
#44335=CARTESIAN_POINT('',(-0.00161353998910187,0.18999314853095,0.185));
#44336=CARTESIAN_POINT('',(-0.00161353998910187,0.18999314853095,0.0925));
#44337=CARTESIAN_POINT('Ctrl Pts',(6.93889390390723E-18,0.184,0.191));
#44338=CARTESIAN_POINT('Ctrl Pts',(-0.000793827160415599,0.186948500881544,
0.188051499118456));
#44339=CARTESIAN_POINT('Ctrl Pts',(-0.00161353998910187,0.18999314853095,
0.185));
#44340=CARTESIAN_POINT('Origin',(0.0342086910003853,0.194007127343405,0.04));
#44341=CARTESIAN_POINT('',(0.0314029373205391,0.18738691397118,0.04));
#44342=CARTESIAN_POINT('',(0.0345809907026646,0.186826537413779,0.04));
#44343=CARTESIAN_POINT('Origin',(0.,0.,0.04));
#44344=CARTESIAN_POINT('',(0.0319512646907152,0.181204626554246,0.04));
#44345=CARTESIAN_POINT('',(0.02957246303897,0.208025165376232,0.04));
#44346=CARTESIAN_POINT('',(0.0319512646907152,0.181204626554246,0.04));
#44347=CARTESIAN_POINT('Origin',(0.0319512646907152,0.181204626554246,0.04));
#44348=CARTESIAN_POINT('',(0.0345809907026646,0.186826537413779,0.185));
#44349=CARTESIAN_POINT('',(0.0345809907026646,0.186826537413779,0.0925));
#44350=CARTESIAN_POINT('',(0.0319512646907152,0.181204626554246,0.191));
#44351=CARTESIAN_POINT('',(0.0319512646907152,0.181204626554246,0.04));
#44352=CARTESIAN_POINT('Ctrl Pts',(0.0345809907026646,0.186826537413779,
0.185));
#44353=CARTESIAN_POINT('Ctrl Pts',(0.0332450336377822,0.183970486442384,
0.188051499118437));
#44354=CARTESIAN_POINT('Ctrl Pts',(0.0319512646907152,0.181204626554246,
0.191));
#44355=CARTESIAN_POINT('Origin',(0.02957246303897,0.208025165376232,0.04));
#44356=CARTESIAN_POINT('',(0.0314029373205391,0.18738691397118,0.185));
#44357=CARTESIAN_POINT('',(0.0314029373205391,0.18738691397118,0.0925));
#44358=CARTESIAN_POINT('Ctrl Pts',(0.0319512646907152,0.181204626554246,
0.191));
#44359=CARTESIAN_POINT('Ctrl Pts',(0.0316814993535166,0.184246179721932,
0.188051499118467));
#44360=CARTESIAN_POINT('Ctrl Pts',(0.0314029373205392,0.18738691397118,
0.185));
#44361=CARTESIAN_POINT('Origin',(0.0673779682351568,0.185119446294824,0.04));
#44362=CARTESIAN_POINT('',(0.0634652522703486,0.179087022852749,0.04));
#44363=CARTESIAN_POINT('',(0.0664977155125526,0.17798329649608,0.04));
#44364=CARTESIAN_POINT('Origin',(0.,0.,0.04));
#44365=CARTESIAN_POINT('',(0.0629317063719231,0.172903442224607,0.04));
#44366=CARTESIAN_POINT('',(0.0652463817528891,0.199729591368321,0.04));
#44367=CARTESIAN_POINT('',(0.0629317063719231,0.172903442224607,0.04));
#44368=CARTESIAN_POINT('Origin',(0.0629317063719231,0.172903442224607,0.04));
#44369=CARTESIAN_POINT('',(0.0664977155125526,0.17798329649608,0.185));
#44370=CARTESIAN_POINT('',(0.0664977155125526,0.17798329649608,0.0925));
#44371=CARTESIAN_POINT('',(0.0629317063719231,0.172903442224607,0.191));
#44372=CARTESIAN_POINT('',(0.0629317063719231,0.172903442224607,0.04));
#44373=CARTESIAN_POINT('Ctrl Pts',(0.0664977155125526,0.17798329649608,
0.185));
#44374=CARTESIAN_POINT('Ctrl Pts',(0.0646861065908417,0.175402621866187,
0.188051499118464));
#44375=CARTESIAN_POINT('Ctrl Pts',(0.0629317063719231,0.172903442224607,
0.191));
#44376=CARTESIAN_POINT('Origin',(0.0652463817528891,0.199729591368321,0.04));
#44377=CARTESIAN_POINT('',(0.0634652522703485,0.179087022852749,0.185));
#44378=CARTESIAN_POINT('',(0.0634652522703485,0.179087022852749,0.0925));
#44379=CARTESIAN_POINT('Ctrl Pts',(0.0629317063719231,0.172903442224607,
0.191));
#44380=CARTESIAN_POINT('Ctrl Pts',(0.0631941995411996,0.175945631624522,
0.188051499118489));
#44381=CARTESIAN_POINT('Ctrl Pts',(0.0634652522703486,0.179087022852749,
0.185));
#44382=CARTESIAN_POINT('Origin',(0.0985,0.170607004545534,0.04));
#44383=CARTESIAN_POINT('',(0.0935992076448906,0.165345663167344,0.04));
#44384=CARTESIAN_POINT('',(0.0963939408860592,0.163732123178242,0.04));
#44385=CARTESIAN_POINT('Origin',(0.,0.,0.04));
#44386=CARTESIAN_POINT('',(0.092,0.159348674296337,0.04));
#44387=CARTESIAN_POINT('',(0.098937822173509,0.185365334794732,0.04));
#44388=CARTESIAN_POINT('',(0.092,0.159348674296337,0.04));
#44389=CARTESIAN_POINT('Origin',(0.092,0.159348674296337,0.04));
#44390=CARTESIAN_POINT('',(0.0963939408860592,0.163732123178242,0.185));
#44391=CARTESIAN_POINT('',(0.0963939408860592,0.163732123178242,0.0925));
#44392=CARTESIAN_POINT('',(0.092,0.159348674296337,0.191));
#44393=CARTESIAN_POINT('',(0.092,0.159348674296337,0.04));
#44394=CARTESIAN_POINT('Ctrl Pts',(0.0963939408860592,0.163732123178242,
0.185));
#44395=CARTESIAN_POINT('Ctrl Pts',(0.0941617249279218,0.161505237382642,
0.188051499118435));
#44396=CARTESIAN_POINT('Ctrl Pts',(0.092,0.159348674296337,0.191));
#44397=CARTESIAN_POINT('Origin',(0.098937822173509,0.185365334794732,0.04));
#44398=CARTESIAN_POINT('',(0.0935992076448906,0.165345663167344,0.185));
#44399=CARTESIAN_POINT('',(0.0935992076448906,0.165345663167344,0.0925));
#44400=CARTESIAN_POINT('Ctrl Pts',(0.092,0.159348674296337,0.191));
#44401=CARTESIAN_POINT('Ctrl Pts',(0.0927867759536358,0.162299064543034,
0.188051499118464));
#44402=CARTESIAN_POINT('Ctrl Pts',(0.0935992076448907,0.165345663167344,
0.185));
#44403=CARTESIAN_POINT('Origin',(0.126629159108248,0.150910755294439,0.04));
#44404=CARTESIAN_POINT('',(0.120889198458627,0.146580359175541,0.04));
#44405=CARTESIAN_POINT('',(0.123361285143431,0.144506032150084,0.04));
#44406=CARTESIAN_POINT('Origin',(0.,0.,0.04));
#44407=CARTESIAN_POINT('',(0.118272920182323,0.140952177533892,0.04));
#44408=CARTESIAN_POINT('',(0.12962308693234,0.165368846322791,0.04));
#44409=CARTESIAN_POINT('',(0.118272920182323,0.140952177533892,0.04));
#44410=CARTESIAN_POINT('Origin',(0.118272920182323,0.140952177533892,0.04));
#44411=CARTESIAN_POINT('',(0.123361285143431,0.144506032150084,0.185));
#44412=CARTESIAN_POINT('',(0.123361285143431,0.144506032150084,0.0925));
#44413=CARTESIAN_POINT('',(0.118272920182323,0.140952177533892,0.191));
#44414=CARTESIAN_POINT('',(0.118272920182323,0.140952177533892,0.04));
#44415=CARTESIAN_POINT('Ctrl Pts',(0.123361285143431,0.144506032150084,
0.185));
#44416=CARTESIAN_POINT('Ctrl Pts',(0.120776286901163,0.142700597986783,
0.188051499118455));
#44417=CARTESIAN_POINT('Ctrl Pts',(0.118272920182323,0.140952177533892,
0.191));
#44418=CARTESIAN_POINT('Origin',(0.12962308693234,0.165368846322791,0.04));
#44419=CARTESIAN_POINT('',(0.120889198458627,0.146580359175541,0.185));
#44420=CARTESIAN_POINT('',(0.120889198458627,0.146580359175541,0.0925));
#44421=CARTESIAN_POINT('Ctrl Pts',(0.118272920182323,0.140952177533892,
0.191));
#44422=CARTESIAN_POINT('Ctrl Pts',(0.119560073131097,0.14372112251268,0.188051499118454));
#44423=CARTESIAN_POINT('Ctrl Pts',(0.120889198458627,0.146580359175541,
0.185));
#44424=CARTESIAN_POINT('Origin',(0.150910755294439,0.126629159108248,0.04));
#44425=CARTESIAN_POINT('',(0.144506032150084,0.123361285143431,0.04));
#44426=CARTESIAN_POINT('',(0.146580359175541,0.120889198458627,0.04));
#44427=CARTESIAN_POINT('Origin',(0.,0.,0.04));
#44428=CARTESIAN_POINT('',(0.140952177533892,0.118272920182323,0.04));
#44429=CARTESIAN_POINT('',(0.15636981978718,0.140347709136006,0.04));
#44430=CARTESIAN_POINT('',(0.140952177533892,0.118272920182323,0.04));
#44431=CARTESIAN_POINT('Origin',(0.140952177533892,0.118272920182323,0.04));
#44432=CARTESIAN_POINT('',(0.146580359175541,0.120889198458627,0.185));
#44433=CARTESIAN_POINT('',(0.146580359175541,0.120889198458627,0.0925));
#44434=CARTESIAN_POINT('',(0.140952177533892,0.118272920182323,0.191));
#44435=CARTESIAN_POINT('',(0.140952177533892,0.118272920182323,0.04));
#44436=CARTESIAN_POINT('Ctrl Pts',(0.146580359175541,0.120889198458627,
0.185));
#44437=CARTESIAN_POINT('Ctrl Pts',(0.14372112251267,0.119560073131093,0.188051499118464));
#44438=CARTESIAN_POINT('Ctrl Pts',(0.140952177533892,0.118272920182323,
0.191));
#44439=CARTESIAN_POINT('Origin',(0.15636981978718,0.140347709136006,0.04));
#44440=CARTESIAN_POINT('',(0.144506032150084,0.123361285143431,0.185));
#44441=CARTESIAN_POINT('',(0.144506032150084,0.123361285143431,0.0925));
#44442=CARTESIAN_POINT('Ctrl Pts',(0.140952177533892,0.118272920182323,
0.191));
#44443=CARTESIAN_POINT('Ctrl Pts',(0.142700597986788,0.120776286901171,
0.188051499118446));
#44444=CARTESIAN_POINT('Ctrl Pts',(0.144506032150084,0.123361285143431,
0.185));
#44445=CARTESIAN_POINT('Origin',(0.170607004545534,0.0985,0.04));
#44446=CARTESIAN_POINT('',(0.163732123178242,0.0963939408860592,0.04));
#44447=CARTESIAN_POINT('',(0.165345663167344,0.0935992076448906,0.04));
#44448=CARTESIAN_POINT('Origin',(0.,0.,0.04));
#44449=CARTESIAN_POINT('',(0.159348674296337,0.092,0.04));
#44450=CARTESIAN_POINT('',(0.178365334794732,0.111062177826491,0.04));
#44451=CARTESIAN_POINT('',(0.159348674296337,0.092,0.04));
#44452=CARTESIAN_POINT('Origin',(0.159348674296337,0.092,0.04));
#44453=CARTESIAN_POINT('',(0.165345663167344,0.0935992076448906,0.185));
#44454=CARTESIAN_POINT('',(0.165345663167344,0.0935992076448906,0.0925));
#44455=CARTESIAN_POINT('',(0.159348674296337,0.092,0.191));
#44456=CARTESIAN_POINT('',(0.159348674296337,0.092,0.04));
#44457=CARTESIAN_POINT('Ctrl Pts',(0.165345663167344,0.0935992076448906,
0.185));
#44458=CARTESIAN_POINT('Ctrl Pts',(0.162299064543034,0.0927867759536356,
0.188051499118465));
#44459=CARTESIAN_POINT('Ctrl Pts',(0.159348674296337,0.092,0.191));
#44460=CARTESIAN_POINT('Origin',(0.178365334794732,0.111062177826491,0.04));
#44461=CARTESIAN_POINT('',(0.163732123178242,0.0963939408860592,0.185));
#44462=CARTESIAN_POINT('',(0.163732123178242,0.0963939408860592,0.0925));
#44463=CARTESIAN_POINT('Ctrl Pts',(0.159348674296337,0.092,0.191));
#44464=CARTESIAN_POINT('Ctrl Pts',(0.161505237382625,0.0941617249279039,
0.188051499118459));
#44465=CARTESIAN_POINT('Ctrl Pts',(0.163732123178242,0.0963939408860592,
0.185));
#44466=CARTESIAN_POINT('Origin',(0.185119446294824,0.0673779682351567,0.04));
#44467=CARTESIAN_POINT('',(0.17798329649608,0.0664977155125525,0.04));
#44468=CARTESIAN_POINT('',(0.179087022852749,0.0634652522703485,0.04));
#44469=CARTESIAN_POINT('Origin',(0.,0.,0.04));
#44470=CARTESIAN_POINT('',(0.172903442224607,0.062931706371923,0.04));
#44471=CARTESIAN_POINT('',(0.194941309361761,0.0784020784438918,0.04));
#44472=CARTESIAN_POINT('',(0.172903442224607,0.062931706371923,0.04));
#44473=CARTESIAN_POINT('Origin',(0.172903442224607,0.062931706371923,0.04));
#44474=CARTESIAN_POINT('',(0.179087022852749,0.0634652522703485,0.185));
#44475=CARTESIAN_POINT('',(0.179087022852749,0.0634652522703485,0.0925));
#44476=CARTESIAN_POINT('',(0.172903442224607,0.062931706371923,0.191));
#44477=CARTESIAN_POINT('',(0.172903442224607,0.062931706371923,0.04));
#44478=CARTESIAN_POINT('Ctrl Pts',(0.179087022852749,0.0634652522703485,
0.185));
#44479=CARTESIAN_POINT('Ctrl Pts',(0.175945631624537,0.0631941995412009,
0.188051499118474));
#44480=CARTESIAN_POINT('Ctrl Pts',(0.172903442224607,0.062931706371923,
0.191));
#44481=CARTESIAN_POINT('Origin',(0.194941309361761,0.0784020784438918,0.04));
#44482=CARTESIAN_POINT('',(0.17798329649608,0.0664977155125525,0.185));
#44483=CARTESIAN_POINT('',(0.17798329649608,0.0664977155125525,0.0925));
#44484=CARTESIAN_POINT('Ctrl Pts',(0.172903442224607,0.062931706371923,
0.191));
#44485=CARTESIAN_POINT('Ctrl Pts',(0.175402621866193,0.0646861065908464,
0.188051499118456));
#44486=CARTESIAN_POINT('Ctrl Pts',(0.17798329649608,0.0664977155125525,
0.185));
#44487=CARTESIAN_POINT('Origin',(0.194007127343405,0.0342086910003853,0.04));
#44488=CARTESIAN_POINT('',(0.186826537413779,0.0345809907026646,0.04));
#44489=CARTESIAN_POINT('',(0.18738691397118,0.0314029373205391,0.04));
#44490=CARTESIAN_POINT('Origin',(0.,0.,0.04));
#44491=CARTESIAN_POINT('',(0.181204626554246,0.0319512646907152,0.04));
#44492=CARTESIAN_POINT('',(0.205594090888895,0.0433597715811408,0.04));
#44493=CARTESIAN_POINT('',(0.181204626554246,0.0319512646907152,0.04));
#44494=CARTESIAN_POINT('Origin',(0.181204626554246,0.0319512646907152,0.04));
#44495=CARTESIAN_POINT('',(0.18738691397118,0.0314029373205391,0.185));
#44496=CARTESIAN_POINT('',(0.18738691397118,0.0314029373205391,0.0925));
#44497=CARTESIAN_POINT('',(0.181204626554246,0.0319512646907152,0.191));
#44498=CARTESIAN_POINT('',(0.181204626554246,0.0319512646907152,0.04));
#44499=CARTESIAN_POINT('Ctrl Pts',(0.18738691397118,0.0314029373205391,
0.185));
#44500=CARTESIAN_POINT('Ctrl Pts',(0.184246179721932,0.0316814993535165,
0.188051499118466));
#44501=CARTESIAN_POINT('Ctrl Pts',(0.181204626554246,0.0319512646907152,
0.191));
#44502=CARTESIAN_POINT('Origin',(0.205594090888895,0.0433597715811408,0.04));
#44503=CARTESIAN_POINT('',(0.186826537413779,0.0345809907026646,0.185));
#44504=CARTESIAN_POINT('',(0.186826537413779,0.0345809907026646,0.0925));
#44505=CARTESIAN_POINT('Ctrl Pts',(0.181204626554246,0.0319512646907152,
0.191));
#44506=CARTESIAN_POINT('Ctrl Pts',(0.183970486442399,0.0332450336377893,
0.18805149911842));
#44507=CARTESIAN_POINT('Ctrl Pts',(0.186826537413779,0.0345809907026646,
0.185));
#44508=CARTESIAN_POINT('Origin',(0.,0.,0.0925));
#44509=CARTESIAN_POINT('Origin',(0.,0.,0.185));
#44510=CARTESIAN_POINT('Origin',(0.,0.,0.185));
#44511=CARTESIAN_POINT('Origin',(0.,0.,0.185));
#44512=CARTESIAN_POINT('Origin',(0.,0.,0.185));
#44513=CARTESIAN_POINT('Origin',(0.,0.,0.185));
#44514=CARTESIAN_POINT('Origin',(0.,0.,0.185));
#44515=CARTESIAN_POINT('Origin',(0.,0.,0.185));
#44516=CARTESIAN_POINT('Origin',(0.,0.,0.185));
#44517=CARTESIAN_POINT('Origin',(0.,0.,0.185));
#44518=CARTESIAN_POINT('Origin',(0.,0.,0.185));
#44519=CARTESIAN_POINT('Origin',(0.,0.,0.185));
#44520=CARTESIAN_POINT('Origin',(0.,0.,0.185));
#44521=CARTESIAN_POINT('Origin',(0.,0.,0.185));
#44522=CARTESIAN_POINT('Origin',(0.,0.,0.185));
#44523=CARTESIAN_POINT('Origin',(0.,0.,0.185));
#44524=CARTESIAN_POINT('Origin',(0.,0.,0.185));
#44525=CARTESIAN_POINT('Origin',(0.,0.,0.185));
#44526=CARTESIAN_POINT('',(-0.19,-2.32682891837997E-17,0.));
#44527=CARTESIAN_POINT('',(-0.19,-2.32682891837997E-17,0.0925));
#44528=CARTESIAN_POINT('Origin',(0.,0.,0.));
#44529=CARTESIAN_POINT('Origin',(0.,0.,0.185));
#44530=CARTESIAN_POINT('Origin',(0.,0.,0.185));
#44531=CARTESIAN_POINT('Origin',(0.,0.,0.185));
#44532=CARTESIAN_POINT('Origin',(0.,0.,0.185));
#44533=CARTESIAN_POINT('Origin',(0.,0.,0.185));
#44534=CARTESIAN_POINT('Origin',(0.,0.,0.185));
#44535=CARTESIAN_POINT('Origin',(0.,0.,0.185));
#44536=CARTESIAN_POINT('Origin',(0.,0.,0.185));
#44537=CARTESIAN_POINT('Origin',(0.,0.,0.185));
#44538=CARTESIAN_POINT('Origin',(0.,0.,0.185));
#44539=CARTESIAN_POINT('Origin',(0.,0.,0.185));
#44540=CARTESIAN_POINT('Origin',(0.,0.,0.185));
#44541=CARTESIAN_POINT('Origin',(0.,0.,0.185));
#44542=CARTESIAN_POINT('Origin',(0.,0.,0.185));
#44543=CARTESIAN_POINT('Origin',(0.,0.,0.185));
#44544=CARTESIAN_POINT('Origin',(0.,0.,0.185));
#44545=CARTESIAN_POINT('Origin',(0.,0.,0.185));
#44546=CARTESIAN_POINT('',(0.18999314853095,0.00161353998910188,0.185));
#44547=CARTESIAN_POINT('Origin',(0.,0.,0.185));
#44548=CARTESIAN_POINT('',(0.18999314853095,0.00161353998910188,0.04));
#44549=CARTESIAN_POINT('',(0.18999314853095,0.00161353998910188,0.0925));
#44550=CARTESIAN_POINT('',(0.18999314853095,-0.00161353998910189,0.04));
#44551=CARTESIAN_POINT('Origin',(0.,0.,0.04));
#44552=CARTESIAN_POINT('',(0.18999314853095,-0.00161353998910189,0.185));
#44553=CARTESIAN_POINT('',(0.18999314853095,-0.00161353998910189,0.0925));
#44554=CARTESIAN_POINT('Origin',(0.,0.,0.185));
#44555=CARTESIAN_POINT('Origin',(0.184,0.,0.04));
#44556=CARTESIAN_POINT('',(0.184,0.,0.04));
#44557=CARTESIAN_POINT('',(0.184,0.,0.04));
#44558=CARTESIAN_POINT('',(0.184,0.,0.191));
#44559=CARTESIAN_POINT('',(0.184,0.,0.04));
#44560=CARTESIAN_POINT('Ctrl Pts',(0.18999314853095,-0.00161353998910188,
0.185));
#44561=CARTESIAN_POINT('Ctrl Pts',(0.186948500881579,-0.000793827160425129,
0.188051499118421));
#44562=CARTESIAN_POINT('Ctrl Pts',(0.184,0.,0.191));
#44563=CARTESIAN_POINT('Origin',(0.21,0.007,0.04));
#44564=CARTESIAN_POINT('Ctrl Pts',(0.184,0.,0.191));
#44565=CARTESIAN_POINT('Ctrl Pts',(0.1869485008816,0.000793827160430761,
0.1880514991184));
#44566=CARTESIAN_POINT('Ctrl Pts',(0.18999314853095,0.00161353998910188,
0.185));
#44567=CARTESIAN_POINT('',(0.21,0.007,0.04));
#44568=CARTESIAN_POINT('Origin',(0.197,0.,0.04));
#44569=CARTESIAN_POINT('Origin',(0.,0.,0.1925));
#44570=CARTESIAN_POINT('',(-0.175,-2.14313189850787E-17,0.2));
#44571=CARTESIAN_POINT('Origin',(0.,0.,0.2));
#44572=CARTESIAN_POINT('',(-0.1825,-2.23498040844392E-17,0.1925));
#44573=CARTESIAN_POINT('Origin',(0.,0.,0.078849364905389));
#44574=CARTESIAN_POINT('',(0.,0.,0.0566987298107781));
#44575=CARTESIAN_POINT('',(-0.0677181486487011,8.29308139868164E-18,0.1));
#44576=CARTESIAN_POINT('',(-0.0346410161513776,-4.24230095489963E-18,0.078849364905389));
#44577=CARTESIAN_POINT('Origin',(0.,0.,0.1));
#44578=CARTESIAN_POINT('Origin',(0.,0.0866025403784439,0.2));
#44579=CARTESIAN_POINT('',(5.30287619362453E-18,0.0866025403784439,0.2));
#44580=CARTESIAN_POINT('',(0.075,0.0433012701892219,0.2));
#44581=CARTESIAN_POINT('',(0.01875,0.0757772228311384,0.2));
#44582=CARTESIAN_POINT('',(0.,0.0866025403784439,0.1));
#44583=CARTESIAN_POINT('',(5.30287619362453E-18,0.0866025403784439,0.2));
#44584=CARTESIAN_POINT('',(0.075,0.0433012701892219,0.1));
#44585=CARTESIAN_POINT('',(0.075,0.0433012701892219,0.1));
#44586=CARTESIAN_POINT('',(0.075,0.0433012701892219,0.2));
#44587=CARTESIAN_POINT('Origin',(-0.075,0.0433012701892219,0.2));
#44588=CARTESIAN_POINT('',(-0.075,0.0433012701892219,0.2));
#44589=CARTESIAN_POINT('',(-0.05625,0.0541265877365274,0.2));
#44590=CARTESIAN_POINT('',(-0.075,0.0433012701892219,0.1));
#44591=CARTESIAN_POINT('',(-0.075,0.0433012701892219,0.2));
#44592=CARTESIAN_POINT('',(5.30287619362453E-18,0.0866025403784439,0.1));
#44593=CARTESIAN_POINT('Origin',(-0.075,-0.0433012701892219,0.2));
#44594=CARTESIAN_POINT('',(-0.075,-0.0433012701892219,0.2));
#44595=CARTESIAN_POINT('',(-0.075,-0.021650635094611,0.2));
#44596=CARTESIAN_POINT('',(-0.075,-0.0433012701892219,0.1));
#44597=CARTESIAN_POINT('',(-0.075,-0.0433012701892219,0.2));
#44598=CARTESIAN_POINT('',(-0.075,0.0433012701892219,0.1));
#44599=CARTESIAN_POINT('Origin',(-1.38777878078145E-17,-0.0866025403784439,
0.2));
#44600=CARTESIAN_POINT('',(-1.59086285808736E-17,-0.0866025403784439,0.2));
#44601=CARTESIAN_POINT('',(-0.01875,-0.0757772228311384,0.2));
#44602=CARTESIAN_POINT('',(-1.38777878078145E-17,-0.0866025403784439,0.1));
#44603=CARTESIAN_POINT('',(-1.59086285808736E-17,-0.0866025403784439,0.2));
#44604=CARTESIAN_POINT('',(-0.075,-0.0433012701892219,0.1));
#44605=CARTESIAN_POINT('Origin',(0.075,-0.043301270189222,0.2));
#44606=CARTESIAN_POINT('',(0.075,-0.043301270189222,0.2));
#44607=CARTESIAN_POINT('',(0.05625,-0.0541265877365275,0.2));
#44608=CARTESIAN_POINT('',(0.075,-0.043301270189222,0.1));
#44609=CARTESIAN_POINT('',(0.075,-0.043301270189222,0.2));
#44610=CARTESIAN_POINT('',(-1.59086285808736E-17,-0.0866025403784439,0.1));
#44611=CARTESIAN_POINT('Origin',(0.075,0.0433012701892219,0.2));
#44612=CARTESIAN_POINT('',(0.075,0.021650635094611,0.2));
#44613=CARTESIAN_POINT('',(0.075,-0.043301270189222,0.1));
#44614=CARTESIAN_POINT('Origin',(0.,0.,0.1));
#44615=CARTESIAN_POINT('Origin',(0.076,0.,-1.2));
#44616=CARTESIAN_POINT('',(-0.076,-9.30731567351988E-18,-1.2));
#44617=CARTESIAN_POINT('Origin',(0.,0.,-1.2));
#44618=CARTESIAN_POINT('Origin',(0.,0.,-1.188));
#44619=CARTESIAN_POINT('',(-0.088,-1.07768918324967E-17,-1.188));
#44620=CARTESIAN_POINT('Origin',(0.,0.,-0.593));
#44621=CARTESIAN_POINT('Origin',(0.,0.,-0.013325));
#44622=CARTESIAN_POINT('Origin',(0.,0.,-0.005));
#44623=CARTESIAN_POINT('',(-0.11,-1.34711147906209E-17,-3.46944695195361E-18));
#44624=CARTESIAN_POINT('Origin',(0.,0.,0.));
#44625=CARTESIAN_POINT('',(-0.105,-1.28587913910472E-17,-0.005));
#44626=CARTESIAN_POINT('Origin',(0.19,0.,0.));
#44627=CARTESIAN_POINT('Origin',(0.,0.,0.2));
#54975=UNCERTAINTY_MEASURE_WITH_UNIT(LENGTH_MEASURE(0.001),#55003,
'DISTANCE_ACCURACY_VALUE',
'Maximum model space distance between geometric entities at asserted c
onnectivities');
#54980=UNCERTAINTY_MEASURE_WITH_UNIT(LENGTH_MEASURE(0.001),#55003,
'DISTANCE_ACCURACY_VALUE',
'Maximum model space distance between geometric entities at asserted c
onnectivities');
#54997=(
GEOMETRIC_REPRESENTATION_CONTEXT(3)
GLOBAL_UNCERTAINTY_ASSIGNED_CONTEXT((#54975))
GLOBAL_UNIT_ASSIGNED_CONTEXT((#55003,#55005,#55006))
REPRESENTATION_CONTEXT('','3D')
);
#55002=(
GEOMETRIC_REPRESENTATION_CONTEXT(3)
GLOBAL_UNCERTAINTY_ASSIGNED_CONTEXT((#54980))
GLOBAL_UNIT_ASSIGNED_CONTEXT((#55003,#55005,#55006))
REPRESENTATION_CONTEXT('','3D')
);
#55003=(
LENGTH_UNIT()
NAMED_UNIT(*)
SI_UNIT(.CENTI.,.METRE.)
);
#55005=(
NAMED_UNIT(*)
PLANE_ANGLE_UNIT()
SI_UNIT($,.RADIAN.)
);
#55006=(
NAMED_UNIT(*)
SI_UNIT($,.STERADIAN.)
SOLID_ANGLE_UNIT()
);
#55023=SHAPE_DEFINITION_REPRESENTATION(#55044,#55119);
#55044=PRODUCT_DEFINITION_SHAPE('',$,#55141);
#55119=SHAPE_REPRESENTATION('',(#26252),#54997);
#55124=PRODUCT_DEFINITION_CONTEXT('part definition',#55189,'design');
#55141=PRODUCT_DEFINITION('2026-10-18-23-36-52-332',
'15_ISO_4762_M2x12_A2',#55162,#55124);
#55162=PRODUCT_DEFINITION_FORMATION('',$,#55207);
#55189=APPLICATION_CONTEXT(
'Core Data for Automotive Mechanical Design Process');
#55190=PRODUCT_CONTEXT('part definition',#55189,'mechanical');
#55207=PRODUCT('2026-10-18-23-36-52-332','15_ISO_4762_M2x12_A2',$,(#55190));
#55387=COLOUR_RGB('Black',0.12,0.14,0.17);
#55388=FILL_AREA_STYLE_COLOUR('',#55387);
#55389=FILL_AREA_STYLE('',(#55388));
#55390=SURFACE_STYLE_FILL_AREA(#55389);
#55391=SURFACE_SIDE_STYLE('',(#55390));
#55392=SURFACE_STYLE_USAGE(.BOTH.,#55391);
#55393=PRESENTATION_STYLE_ASSIGNMENT((#55392));
ENDSEC;
END-ISO-10303-21;
